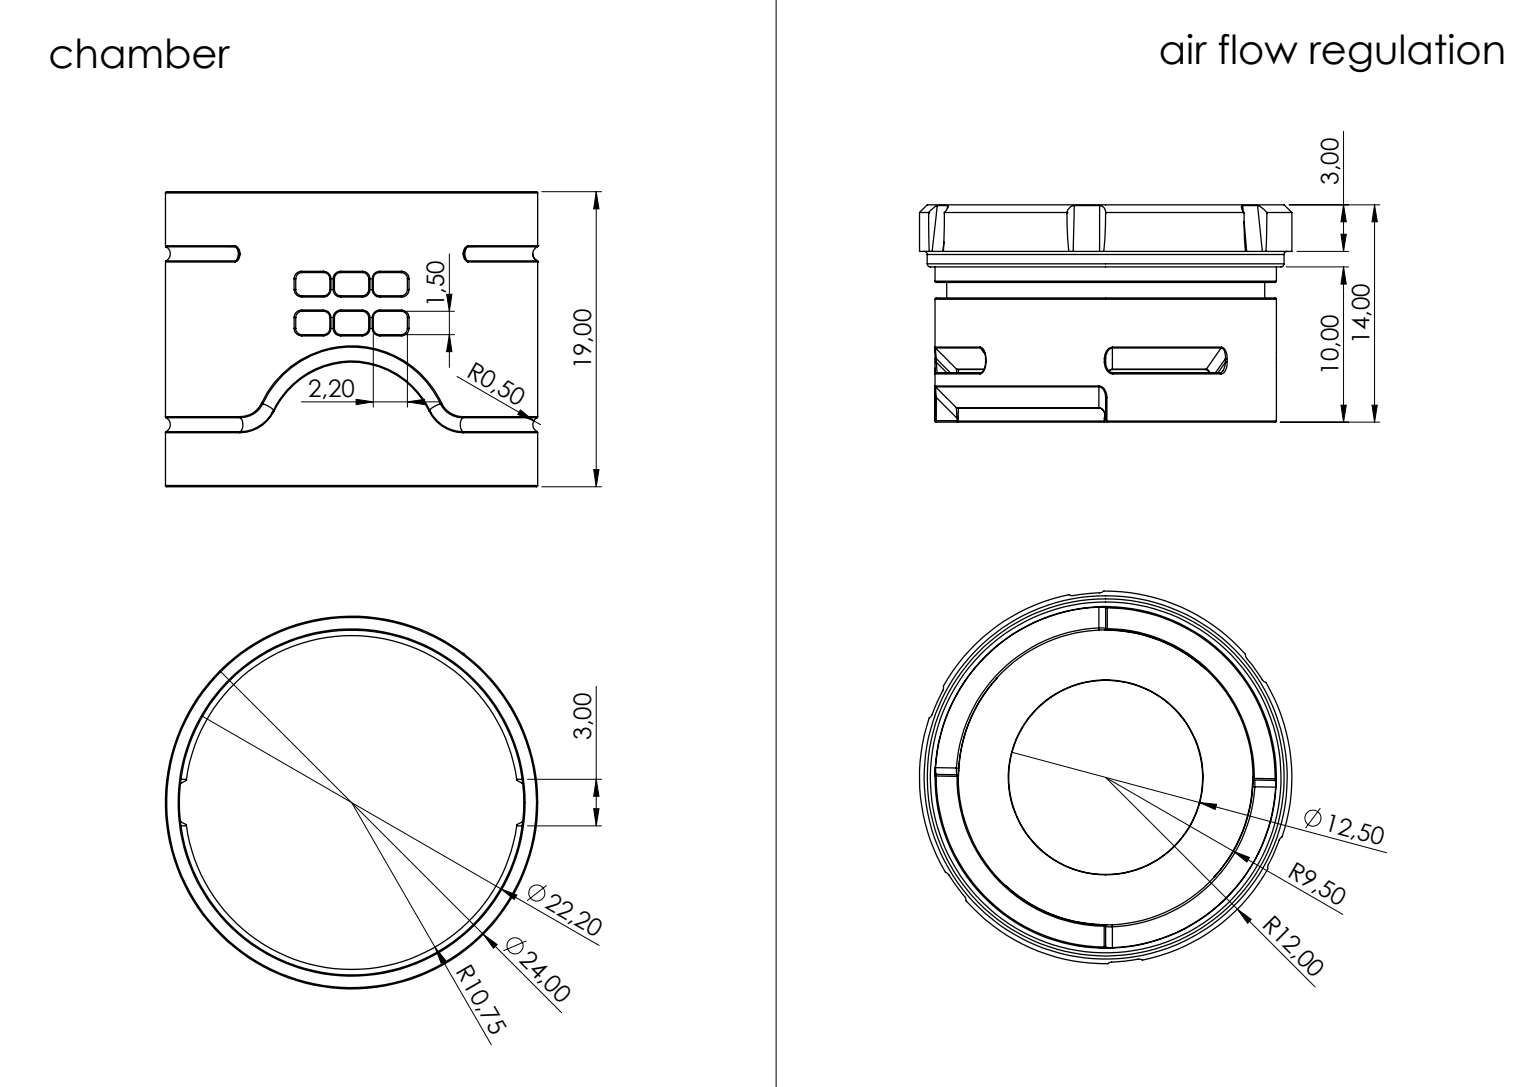
ISO-10303-21;
HEADER;
FILE_DESCRIPTION (('STEP AP214'),
    '1' );
FILE_NAME ('air flow regulation.step',
    '2026-10-05T20:10:51',
    ( '' ),
    ( '' ),
    'SwSTEP 2.0',
    'SolidWorks 2020',
    '' );
FILE_SCHEMA (( 'AUTOMOTIVE_DESIGN' ));
ENDSEC;

DATA;
#10=CARTESIAN_POINT ( 'NONE',  ( 8.996750068618124985, 1.000000000000000888, 7.838941051145326355 ) ) ;
#11=ADVANCED_FACE ( 'NONE', ( #143939 ), #115364, .T. ) ;
#35=CARTESIAN_POINT ( 'NONE',  ( -0.4382560683119374190, -5.166862915010145052, -10.99126615174919408 ) ) ;
#43=CARTESIAN_POINT ( 'NONE',  ( 0.000000000000000000, 4.000000000000003553, 0.000000000000000000 ) ) ;
#68=EDGE_LOOP ( 'NONE', ( #150530, #161755, #187821, #170704 ) ) ;
#69=CARTESIAN_POINT ( 'NONE',  ( 6.731761806397376091, -7.792646766724933727, 6.779954559072931985 ) ) ;
#135=ORIENTED_EDGE ( 'NONE', *, *, #160637, .F. ) ;
#138=CARTESIAN_POINT ( 'NONE',  ( 6.446420058208158110, -6.527411821100059797, 7.058808231563617142 ) ) ;
#156=VERTEX_POINT ( 'NONE', #175348 ) ;
#179=DIRECTION ( 'NONE',  ( 0.000000000000000000, 0.000000000000000000, -1.000000000000000000 ) ) ;
#202=CARTESIAN_POINT ( 'NONE',  ( 0.3663205537283338309, -5.223179855899201307, 10.97093617010627220 ) ) ;
#238=CARTESIAN_POINT ( 'NONE',  ( -6.451695228975252050, -8.176248043968191936, -7.005920419303019564 ) ) ;
#294=CARTESIAN_POINT ( 'NONE',  ( 7.654042494670958593E-16, 3.079999999999999183, -6.250000000000000000 ) ) ;
#317=VECTOR ( 'NONE', #161091, 1000.000000000000114 ) ;
#322=VERTEX_POINT ( 'NONE', #162281 ) ;
#357=PRESENTATION_STYLE_ASSIGNMENT (( #184467 ) ) ;
#401=VERTEX_POINT ( 'NONE', #180650 ) ;
#455=CARTESIAN_POINT ( 'NONE',  ( -10.99896775280371486, -5.324706741106397523, 0.1653080603930973391 ) ) ;
#523=CARTESIAN_POINT ( 'NONE',  ( 10.39230484541318589, 3.447199233515649386, -6.000000000000107470 ) ) ;
#529=( GEOMETRIC_REPRESENTATION_CONTEXT ( 3 ) GLOBAL_UNCERTAINTY_ASSIGNED_CONTEXT ( ( #23794 ) ) GLOBAL_UNIT_ASSIGNED_CONTEXT ( ( #120191, #135322, #18334 ) ) REPRESENTATION_CONTEXT ( 'NONE', 'WORKASPACE' ) );
#551=CARTESIAN_POINT ( 'NONE',  ( 10.99431798667268190, -5.199791778944933718, -0.3617173305618991974 ) ) ;
#571=AXIS2_PLACEMENT_3D ( 'NONE', #49828, #181943, #33573 ) ;
#585=CARTESIAN_POINT ( 'NONE',  ( -6.905598574191406769, -7.287292132484036955, -6.905598574191375683 ) ) ;
#620=CIRCLE ( 'NONE', #184019, 0.07999999999999951594 ) ;
#629=CARTESIAN_POINT ( 'NONE',  ( -0.1007670162816230591, -8.052608368926286175, -9.499791922504428499 ) ) ;
#644=CARTESIAN_POINT ( 'NONE',  ( 10.91970695577495043, 0.000000000000000000, 5.204170427930421283E-15 ) ) ;
#661=ORIENTED_EDGE ( 'NONE', *, *, #178265, .T. ) ;
#727=ORIENTED_EDGE ( 'NONE', *, *, #105154, .T. ) ;
#734=CARTESIAN_POINT ( 'NONE',  ( -7.235142258280575334, -6.594478602024302027, 7.235142258280601091 ) ) ;
#788=CARTESIAN_POINT ( 'NONE',  ( 6.717278222822382183, -7.473374494058216300, -6.830415307812249814 ) ) ;
#833=VECTOR ( 'NONE', #207710, 1000.000000000000000 ) ;
#842=ORIENTED_EDGE ( 'NONE', *, *, #62981, .F. ) ;
#869=AXIS2_PLACEMENT_3D ( 'NONE', #75473, #189221, #172990 ) ;
#886=UNCERTAINTY_MEASURE_WITH_UNIT (LENGTH_MEASURE( 1.000000000000000082E-05 ), #29913, 'distance_accuracy_value', 'NONE');
#918=CARTESIAN_POINT ( 'NONE',  ( -7.986233326679965216, -6.863455982311493564, 7.564733433744408764 ) ) ;
#954=EDGE_CURVE ( 'NONE', #82527, #56186, #181684, .T. ) ;
#1031=MECHANICAL_DESIGN_GEOMETRIC_PRESENTATION_REPRESENTATION('',(#101406),#122221);
#1044=DIRECTION ( 'NONE',  ( 0.000000000000000000, 1.000000000000000000, 0.000000000000000000 ) ) ;
#1055=CARTESIAN_POINT ( 'NONE',  ( 7.721398836998391246, -5.907420853759296264, 7.721398836998372595 ) ) ;
#1065=CARTESIAN_POINT ( 'NONE',  ( 0.000000000000000000, -9.063431457505059186, 0.000000000000000000 ) ) ;
#1080=CARTESIAN_POINT ( 'NONE',  ( 9.000007961041747606, 1.000000000000000888, 7.937244906211794238 ) ) ;
#1108=SURFACE_SIDE_STYLE ('',( #195073 ) ) ;
#1115=DIRECTION ( 'NONE',  ( 0.000000000000000000, 1.000000000000000000, 0.000000000000000000 ) ) ;
#1118=CARTESIAN_POINT ( 'NONE',  ( -5.204170427930421283E-15, -5.907420853759282053, 10.91970695577496997 ) ) ;
#1120=CARTESIAN_POINT ( 'NONE',  ( -0.08058608058609216529, -9.999999999999994671, -10.99970480893080271 ) ) ;
#1172=ADVANCED_FACE ( 'NONE', ( #46789 ), #131277, .T. ) ;
#1181=CARTESIAN_POINT ( 'NONE',  ( 0.07999999999999327094, -8.407420853759283830, 10.91970695577496286 ) ) ;
#1230=ORIENTED_EDGE ( 'NONE', *, *, #175281, .T. ) ;
#1236=CARTESIAN_POINT ( 'NONE',  ( 9.606148981167590861, -6.583980363595129504, -0.4355862708379804604 ) ) ;
#1239=CARTESIAN_POINT ( 'NONE',  ( -2.467126471220350226, 3.603011019375347068, 11.63837686854861886 ) ) ;
#1249=( GEOMETRIC_REPRESENTATION_CONTEXT ( 3 ) GLOBAL_UNCERTAINTY_ASSIGNED_CONTEXT ( ( #40635 ) ) GLOBAL_UNIT_ASSIGNED_CONTEXT ( ( #90258, #110825, #176833 ) ) REPRESENTATION_CONTEXT ( 'NONE', 'WORKASPACE' ) );
#1258=ORIENTED_EDGE ( 'NONE', *, *, #48325, .T. ) ;
#1267=ADVANCED_FACE ( 'NONE', ( #96609 ), #117015, .T. ) ;
#1301=VERTEX_POINT ( 'NONE', #170096 ) ;
#1303=ORIENTED_EDGE ( 'NONE', *, *, #173163, .T. ) ;
#1316=CARTESIAN_POINT ( 'NONE',  ( 9.499633409936901529, -9.910600865424404660, -0.08345703571627054174 ) ) ;
#1328=CARTESIAN_POINT ( 'NONE',  ( 9.578206935409037115, -9.746166700193986898, -0.1671882239534273895 ) ) ;
#1382=CARTESIAN_POINT ( 'NONE',  ( 7.752014238602739730E-16, 1.000000000000002665, -6.329999999999995630 ) ) ;
#1403=CARTESIAN_POINT ( 'NONE',  ( 2.494940289813108780, 3.499999999999989342, -11.73777120880564695 ) ) ;
#1422=CARTESIAN_POINT ( 'NONE',  ( -0.2887529476172396303, 1.000000000000000888, 11.89119375935166012 ) ) ;
#1434=( LENGTH_UNIT ( ) NAMED_UNIT ( * ) SI_UNIT ( .MILLI., .METRE. ) );
#1461=VECTOR ( 'NONE', #26119, 1000.000000000000000 ) ;
#1465=CARTESIAN_POINT ( 'NONE',  ( -6.766604819867150233, -7.256397064628574256, -6.766604819867120035 ) ) ;
#1472=DIRECTION ( 'NONE',  ( 0.000000000000000000, -1.000000000000000000, 0.000000000000000000 ) ) ;
#1528=CARTESIAN_POINT ( 'NONE',  ( -10.96107445065241315, -5.401429653175735979, 0.1376292675369562291 ) ) ;
#1532=( NAMED_UNIT ( * ) SI_UNIT ( $, .STERADIAN. ) SOLID_ANGLE_UNIT ( ) );
#1572=CARTESIAN_POINT ( 'NONE',  ( 9.611540586923190688, -6.723650695528643695, -0.1589091098076216013 ) ) ;
#1578=CARTESIAN_POINT ( 'NONE',  ( -4.480158349507305421E-13, -7.034525084948354490, 10.67552547708289268 ) ) ;
#1583=ORIENTED_EDGE ( 'NONE', *, *, #204878, .F. ) ;
#1589=CARTESIAN_POINT ( 'NONE',  ( -6.756361134959188774, -6.891066458783145166, -6.828399852920279400 ) ) ;
#1658=CARTESIAN_POINT ( 'NONE',  ( -11.00029519899100450, -6.134628647623513231, 8.483881999699072196E-15 ) ) ;
#1659=ADVANCED_FACE ( 'NONE', ( #152790 ), #205507, .T. ) ;
#1684=UNCERTAINTY_MEASURE_WITH_UNIT (LENGTH_MEASURE( 1.000000000000000082E-05 ), #105985, 'distance_accuracy_value', 'NONE');
#1708=CARTESIAN_POINT ( 'NONE',  ( -0.4644097342743139234, -8.233137084989849086, -9.488641820551089623 ) ) ;
#1746=DIRECTION ( 'NONE',  ( 0.03984146075563027578, 0.000000000000000000, 0.9992060137953822085 ) ) ;
#1753=DIRECTION ( 'NONE',  ( 0.000000000000000000, -1.084202172485501594E-14, -1.000000000000000000 ) ) ;
#1763=CARTESIAN_POINT ( 'NONE',  ( -6.735629246274043785E-15, -9.954379061088852509, 9.579665937614933569 ) ) ;
#1771=CARTESIAN_POINT ( 'NONE',  ( -7.721398836998370818, -5.907420853759296264, 7.721398836998400128 ) ) ;
#1785=DIRECTION ( 'NONE',  ( 0.9999455182791219254, 0.000000000000000000, -0.01043841336116897722 ) ) ;
#1801=VERTEX_POINT ( 'NONE', #63560 ) ;
#1811=CARTESIAN_POINT ( 'NONE',  ( -7.636191794455529092, -6.027819618361862197, 7.636191794455553961 ) ) ;
#1832=ORIENTED_EDGE ( 'NONE', *, *, #152899, .F. ) ;
#1838=CARTESIAN_POINT ( 'NONE',  ( 9.490416961614043245, -9.037429132956701139, -0.4317745627846678591 ) ) ;
#1871=VERTEX_POINT ( 'NONE', #114513 ) ;
#1887=CARTESIAN_POINT ( 'NONE',  ( 9.797921721691059460, 3.956598013261175772, 6.103348209225848642 ) ) ;
#1896=SURFACE_STYLE_FILL_AREA ( #165491 ) ;
#1902=ORIENTED_EDGE ( 'NONE', *, *, #91274, .F. ) ;
#1928=EDGE_CURVE ( 'NONE', #32900, #45587, #28933, .T. ) ;
#1931=CARTESIAN_POINT ( 'NONE',  ( 0.3618152180564599973, -5.223163831703878657, 10.97113184882214298 ) ) ;
#1978=DIRECTION ( 'NONE',  ( -0.9988044021632737079, 2.913101175831703182E-16, 0.04888523518676889112 ) ) ;
#2059=CIRCLE ( 'NONE', #123265, 0.08000000000000020983 ) ;
#2106=DIRECTION ( 'NONE',  ( 0.000000000000000000, 1.000000000000000000, 0.000000000000000000 ) ) ;
#2129=FACE_OUTER_BOUND ( 'NONE', #90690, .T. ) ;
#2169=EDGE_CURVE ( 'NONE', #89957, #26009, #98210, .T. ) ;
#2173=CARTESIAN_POINT ( 'NONE',  ( -0.3459972005395436367, -9.006862989983622114, 9.494064636159285087 ) ) ;
#2192=DIRECTION ( 'NONE',  ( 0.000000000000000000, 0.000000000000000000, -1.000000000000000000 ) ) ;
#2211=CARTESIAN_POINT ( 'NONE',  ( 11.29689844398643395, -5.530538574611989056, 9.269928574751062911E-15 ) ) ;
#2212=CIRCLE ( 'NONE', #109479, 10.99999999999999112 ) ;
#2238=CARTESIAN_POINT ( 'NONE',  ( -6.717278222822391953, 7.849261790823902629, 6.830415307812263137 ) ) ;
#2254=ORIENTED_EDGE ( 'NONE', *, *, #31074, .T. ) ;
#2263=CARTESIAN_POINT ( 'NONE',  ( 10.54982673430220252, -8.131911363926706215, -0.6210660986541617357 ) ) ;
#2298=B_SPLINE_CURVE_WITH_KNOTS ( 'NONE', 3,
 ( #197808, #82989, #212983, #98207, #49441, #15846 ),
 .UNSPECIFIED., .F., .F.,
 ( 4, 2, 4 ),
 ( 0.000000000000000000, 0.001226111284895915667, 0.002452222569791831768 ),
 .UNSPECIFIED. ) ;
#2309=CARTESIAN_POINT ( 'NONE',  ( -9.834497819152506537, 3.956598013261176217, -6.044631300485411529 ) ) ;
#2315=CARTESIAN_POINT ( 'NONE',  ( 0.4373225248172820656, -7.723431457505077979, -10.96785329849813273 ) ) ;
#2329=ORIENTED_EDGE ( 'NONE', *, *, #181317, .T. ) ;
#2362=ORIENTED_EDGE ( 'NONE', *, *, #105101, .T. ) ;
#2376=DIRECTION ( 'NONE',  ( 0.000000000000000000, -1.000000000000000000, 0.000000000000000000 ) ) ;
#2379=CARTESIAN_POINT ( 'NONE',  ( -10.99958311221863028, -9.919613946868093279, 0.09579086958121280082 ) ) ;
#2389=EDGE_CURVE ( 'NONE', #80737, #93709, #181246, .T. ) ;
#2405=CARTESIAN_POINT ( 'NONE',  ( 10.99943760478736010, -9.902953797791681723, -0.1112316694888297319 ) ) ;
#2480=CARTESIAN_POINT ( 'NONE',  ( -2.423460580168067757, 1.405705671057797312, 11.75284646727700455 ) ) ;
#2486=( NAMED_UNIT ( * ) PLANE_ANGLE_UNIT ( ) SI_UNIT ( $, .RADIAN. ) );
#2534=ORIENTED_EDGE ( 'NONE', *, *, #164125, .F. ) ;
#2539=CARTESIAN_POINT ( 'NONE',  ( 6.634380643896210294, -6.684699857435318471, 6.783773228136968036 ) ) ;
#2559=ORIENTED_EDGE ( 'NONE', *, *, #185505, .F. ) ;
#2599=CARTESIAN_POINT ( 'NONE',  ( -10.97067990664313264, -5.250949308401990479, 0.2977236940312626978 ) ) ;
#2601=CARTESIAN_POINT ( 'NONE',  ( 4.806723615010448736E-13, -7.868798029037617603, -9.500000000000001776 ) ) ;
#2610=CARTESIAN_POINT ( 'NONE',  ( 0.2619794211619203006, -6.848541063415906294, 10.99716886186657838 ) ) ;
#2635=EDGE_CURVE ( 'NONE', #192481, #119756, #206152, .T. ) ;
#2639=CARTESIAN_POINT ( 'NONE',  ( 9.484899655072776881, -6.713792789267319705, -0.3525790917591882789 ) ) ;
#2656=CARTESIAN_POINT ( 'NONE',  ( -5.204170427930421283E-15, 3.447199233515649386, -11.99999999999998224 ) ) ;
#2666=CARTESIAN_POINT ( 'NONE',  ( 0.4355862708379890647, -6.583980363594969631, 9.606148981167454082 ) ) ;
#2672=( GEOMETRIC_REPRESENTATION_CONTEXT ( 3 ) GLOBAL_UNCERTAINTY_ASSIGNED_CONTEXT ( ( #41987 ) ) GLOBAL_UNIT_ASSIGNED_CONTEXT ( ( #14906, #152407, #132983 ) ) REPRESENTATION_CONTEXT ( 'NONE', 'WORKASPACE' ) );
#2715=SURFACE_STYLE_USAGE ( .BOTH. , #5913 ) ;
#2753=STYLED_ITEM ( 'NONE', ( #168925 ), #37195 ) ;
#2797=ORIENTED_EDGE ( 'NONE', *, *, #2169, .T. ) ;
#2814=DIRECTION ( 'NONE',  ( -1.000000000000000000, 0.000000000000000000, 0.000000000000000000 ) ) ;
#2827=CARTESIAN_POINT ( 'NONE',  ( 1.730579039399254279E-05, -9.953931234596407052, 9.500331159997204011 ) ) ;
#2829=CIRCLE ( 'NONE', #144696, 0.07999999999999993228 ) ;
#2849=CARTESIAN_POINT ( 'NONE',  ( -7.727353211424288659, -6.453073674884717725, 7.679448064523577422 ) ) ;
#2852=CARTESIAN_POINT ( 'NONE',  ( -1.179069862577986269E-15, -8.198316280121948907, -9.513083155459820972 ) ) ;
#2865=EDGE_LOOP ( 'NONE', ( #190728, #42834, #5149, #106081 ) ) ;
#2870=EDGE_LOOP ( 'NONE', ( #204909, #147403, #53351, #186088 ) ) ;
#2889=ORIENTED_EDGE ( 'NONE', *, *, #89791, .F. ) ;
#2907=ORIENTED_EDGE ( 'NONE', *, *, #117967, .T. ) ;
#2920=DIRECTION ( 'NONE',  ( 1.561558963378126405E-12, 1.000000000000000000, 1.535693738323023938E-12 ) ) ;
#2921=CARTESIAN_POINT ( 'NONE',  ( -7.834948825496940827, -6.134628647623485698, -7.720982897393570354 ) ) ;
#2970=B_SPLINE_CURVE_WITH_KNOTS ( 'NONE', 3,
 ( #68679, #58594, #2610, #119655, #169405, #70808 ),
 .UNSPECIFIED., .F., .F.,
 ( 4, 2, 4 ),
 ( 0.000000000000000000, 0.0003147459536107388863, 0.0006294919072214776642 ),
 .UNSPECIFIED. ) ;
#2972=ORIENTED_EDGE ( 'NONE', *, *, #194076, .T. ) ;
#3055=CARTESIAN_POINT ( 'NONE',  ( -7.887197531381538340, -6.766388843766927508, 7.667935170093262975 ) ) ;
#3059=EDGE_LOOP ( 'NONE', ( #52191, #98069, #29595, #193700 ) ) ;
#3073=VECTOR ( 'NONE', #149450, 1000.000000000000000 ) ;
#3089=CARTESIAN_POINT ( 'NONE',  ( -0.3728355200475085285, -6.583727468837148322, -9.609247538825096413 ) ) ;
#3131=CARTESIAN_POINT ( 'NONE',  ( 9.007749180437182090, 1.970899860167747653, 7.589917856494929893 ) ) ;
#3155=CARTESIAN_POINT ( 'NONE',  ( -0.04481625915950731426, -9.999534456186221831, -9.500049708090200440 ) ) ;
#3160=ORIENTED_EDGE ( 'NONE', *, *, #11469, .F. ) ;
#3163=CARTESIAN_POINT ( 'NONE',  ( -0.09481041353608977984, -9.919511983836045488, -9.499526882191805299 ) ) ;
#3172=CARTESIAN_POINT ( 'NONE',  ( 0.07917133907661091929, -6.459673408256485949, 11.00057242252814760 ) ) ;
#3175=ORIENTED_EDGE ( 'NONE', *, *, #3623, .T. ) ;
#3181=CARTESIAN_POINT ( 'NONE',  ( 6.773846765317333762, -7.246166700180801001, 6.773846765317311558 ) ) ;
#3188=CARTESIAN_POINT ( 'NONE',  ( -9.499606442108964544, -9.746166700193986898, 0.08647222121513538362 ) ) ;
#3190=CARTESIAN_POINT ( 'NONE',  ( 0.000000000000000000, -7.723431457505077979, 0.000000000000000000 ) ) ;
#3195=SURFACE_SIDE_STYLE ('',( #85540 ) ) ;
#3197=EDGE_LOOP ( 'NONE', ( #209100, #72520, #9846, #141144 ) ) ;
#3207=CARTESIAN_POINT ( 'NONE',  ( -10.97895254167818990, -5.212340523078042409, 0.4373349612950744314 ) ) ;
#3210=ADVANCED_FACE ( 'NONE', ( #41628 ), #28556, .T. ) ;
#3214=ORIENTED_EDGE ( 'NONE', *, *, #200691, .T. ) ;
#3236=FILL_AREA_STYLE ('',( #151664 ) ) ;
#3309=CARTESIAN_POINT ( 'NONE',  ( -6.940534579975167873, -6.675176078274437153, 6.653311379900154421 ) ) ;
#3313=ORIENTED_EDGE ( 'NONE', *, *, #102930, .F. ) ;
#3370=FACE_OUTER_BOUND ( 'NONE', #25693, .T. ) ;
#3393=( GEOMETRIC_REPRESENTATION_CONTEXT ( 3 ) GLOBAL_UNCERTAINTY_ASSIGNED_CONTEXT ( ( #195972 ) ) GLOBAL_UNIT_ASSIGNED_CONTEXT ( ( #189438, #41080, #178527 ) ) REPRESENTATION_CONTEXT ( 'NONE', 'WORKASPACE' ) );
#3427=EDGE_LOOP ( 'NONE', ( #194768, #195116, #182169, #158522 ) ) ;
#3440=ORIENTED_EDGE ( 'NONE', *, *, #3532, .T. ) ;
#3449=CARTESIAN_POINT ( 'NONE',  ( -6.773376349083140013, -7.473374494058229622, -6.661184041420940893 ) ) ;
#3461=FACE_OUTER_BOUND ( 'NONE', #173063, .T. ) ;
#3469=CARTESIAN_POINT ( 'NONE',  ( 6.756361134959112391, -6.891066458783287274, 6.828399852920186142 ) ) ;
#3472=CARTESIAN_POINT ( 'NONE',  ( 0.000000000000000000, 1.000000000000000888, 0.000000000000000000 ) ) ;
#3532=EDGE_CURVE ( 'NONE', #157260, #71638, #13059, .T. ) ;
#3537=EDGE_CURVE ( 'NONE', #105884, #200355, #58064, .T. ) ;
#3541=B_SPLINE_CURVE_WITH_KNOTS ( 'NONE', 3,
 ( #196882, #64746, #148151, #181682 ),
 .UNSPECIFIED., .F., .F.,
 ( 4, 4 ),
 ( 0.000000000000000000, 9.170750102249441526E-05 ),
 .UNSPECIFIED. ) ;
#3557=DIRECTION ( 'NONE',  ( 0.000000000000000000, 1.000000000000000000, 0.000000000000000000 ) ) ;
#3571=EDGE_CURVE ( 'NONE', #129112, #183707, #115658, .T. ) ;
#3605=DIRECTION ( 'NONE',  ( 0.000000000000000000, -1.000000000000000000, 0.000000000000000000 ) ) ;
#3611=FACE_OUTER_BOUND ( 'NONE', #77172, .T. ) ;
#3621=FACE_OUTER_BOUND ( 'NONE', #70263, .T. ) ;
#3623=EDGE_CURVE ( 'NONE', #183133, #82411, #22756, .T. ) ;
#3629=CARTESIAN_POINT ( 'NONE',  ( -6.661184042391488980, -7.215568602681072363, 6.773376348128680391 ) ) ;
#3669=CIRCLE ( 'NONE', #187065, 8.049999999999993605 ) ;
#3716=CARTESIAN_POINT ( 'NONE',  ( -6.484567079770451770, -6.583980363594983842, -7.100579091573043122 ) ) ;
#3751=CARTESIAN_POINT ( 'NONE',  ( 10.94526678918447971, -5.600264386821002915, -0.03132844593992607785 ) ) ;
#3792=EDGE_CURVE ( 'NONE', #191954, #56186, #148063, .T. ) ;
#3806=UNCERTAINTY_MEASURE_WITH_UNIT (LENGTH_MEASURE( 1.000000000000000082E-05 ), #124958, 'distance_accuracy_value', 'NONE');
#3815=VECTOR ( 'NONE', #3943, 1000.000000000000000 ) ;
#3829=CARTESIAN_POINT ( 'NONE',  ( 0.08058608058607032165, -5.907420853759267843, -10.99970480893079916 ) ) ;
#3861=( NAMED_UNIT ( * ) PLANE_ANGLE_UNIT ( ) SI_UNIT ( $, .RADIAN. ) );
#3864=ORIENTED_EDGE ( 'NONE', *, *, #113758, .T. ) ;
#3916=DIRECTION ( 'NONE',  ( 0.000000000000000000, 0.000000000000000000, -1.000000000000000000 ) ) ;
#3937=AXIS2_PLACEMENT_3D ( 'NONE', #168326, #86007, #119639 ) ;
#3943=DIRECTION ( 'NONE',  ( 0.000000000000000000, 1.000000000000000000, 0.000000000000000000 ) ) ;
#3968=ORIENTED_EDGE ( 'NONE', *, *, #108052, .T. ) ;
#3990=FACE_OUTER_BOUND ( 'NONE', #157458, .T. ) ;
#4030=AXIS2_PLACEMENT_3D ( 'NONE', #178607, #77890, #98413 ) ;
#4095=B_SPLINE_CURVE_WITH_KNOTS ( 'NONE', 3,
 ( #171376, #88001, #55498, #187619, #185480, #54437, #37105, #20833 ),
 .UNSPECIFIED., .F., .F.,
 ( 4, 2, 2, 4 ),
 ( 0.000000000000000000, 0.0002185754043082796050, 0.0004371508086165592100, 0.0008743016172331182032 ),
 .UNSPECIFIED. ) ;
#4097=DIRECTION ( 'NONE',  ( 0.000000000000000000, 1.000000000000000000, 0.000000000000000000 ) ) ;
#4115=( LENGTH_UNIT ( ) NAMED_UNIT ( * ) SI_UNIT ( .MILLI., .METRE. ) );
#4172=EDGE_CURVE ( 'NONE', #157711, #182623, #58845, .T. ) ;
#4190=CARTESIAN_POINT ( 'NONE',  ( 0.000000000000000000, -7.666862915010147717, 0.000000000000000000 ) ) ;
#4201=EDGE_CURVE ( 'NONE', #168636, #175139, #105282, .T. ) ;
#4238=CARTESIAN_POINT ( 'NONE',  ( 0.01400375820003852204, -6.304807775344445808, 11.00039779440905896 ) ) ;
#4241=ORIENTED_EDGE ( 'NONE', *, *, #201124, .T. ) ;
#4271=CARTESIAN_POINT ( 'NONE',  ( -9.827407719474578585, -6.362962251424048254, 0.4359508081056245876 ) ) ;
#4299=ORIENTED_EDGE ( 'NONE', *, *, #14312, .F. ) ;
#4370=CARTESIAN_POINT ( 'NONE',  ( 7.720982897393571243, -5.907420853759296264, -7.834948825496923952 ) ) ;
#4376=CARTESIAN_POINT ( 'NONE',  ( -6.775478006741569637, -7.217909409563595169, 6.775478006741592729 ) ) ;
#4419=VECTOR ( 'NONE', #202531, 1000.000000000000000 ) ;
#4429=ADVANCED_FACE ( 'NONE', ( #170516 ), #84039, .T. ) ;
#4434=CARTESIAN_POINT ( 'NONE',  ( -10.87798840695972302, -6.646059016331640201, 0.1412570932018041570 ) ) ;
#4475=CARTESIAN_POINT ( 'NONE',  ( 10.14031698345507060, 3.934660213246449434, -5.561808457406779205 ) ) ;
#4491=CARTESIAN_POINT ( 'NONE',  ( -2.927345865710861577E-15, -6.948429295162506847, 9.261794192843273876 ) ) ;
#4537=CARTESIAN_POINT ( 'NONE',  ( 0.000000000000000000, -8.233137084989836652, 0.000000000000000000 ) ) ;
#4542=EDGE_CURVE ( 'NONE', #29585, #38980, #65003, .T. ) ;
#4548=CIRCLE ( 'NONE', #18331, 0.07999999999999982125 ) ;
#4566=AXIS2_PLACEMENT_3D ( 'NONE', #192689, #160212, #195917 ) ;
#4569=DIRECTION ( 'NONE',  ( 0.5254827454987551771, 0.7071067811865540120, 0.4731467892558094412 ) ) ;
#4615=CARTESIAN_POINT ( 'NONE',  ( -0.1236583036082171405, 1.000000000000000888, 11.99936284241579898 ) ) ;
#4627=( NAMED_UNIT ( * ) SI_UNIT ( $, .STERADIAN. ) SOLID_ANGLE_UNIT ( ) );
#4635=CARTESIAN_POINT ( 'NONE',  ( 0.08058608058607655278, -9.999999999999994671, 10.99970480893082225 ) ) ;
#4639=AXIS2_PLACEMENT_3D ( 'NONE', #184989, #4097, #134162 ) ;
#4660=FACE_OUTER_BOUND ( 'NONE', #40687, .T. ) ;
#4686=CARTESIAN_POINT ( 'NONE',  ( -4.218316008240990271E-13, -9.350066838357692589, -9.500000000000001776 ) ) ;
#4702=CIRCLE ( 'NONE', #129312, 0.08000000000000020983 ) ;
#4715=PLANE ( 'NONE',  #59335 ) ;
#4737=CARTESIAN_POINT ( 'NONE',  ( -9.579603127937250662, 7.849261790823902629, 0.08720040834116031536 ) ) ;
#4739=EDGE_LOOP ( 'NONE', ( #128508, #164924 ) ) ;
#4750=B_SPLINE_CURVE_WITH_KNOTS ( 'NONE', 3,
 ( #36336, #102414, #20080, #70954 ),
 .UNSPECIFIED., .F., .F.,
 ( 4, 4 ),
 ( 0.000000000000000000, 0.0002909236271752618720 ),
 .UNSPECIFIED. ) ;
#4751=CARTESIAN_POINT ( 'NONE',  ( -10.99915817693634246, -6.765468805240992367, 0.1539349733294695932 ) ) ;
#4765=ORIENTED_EDGE ( 'NONE', *, *, #43078, .F. ) ;
#4771=EDGE_LOOP ( 'NONE', ( #69677, #173344, #50516, #196043 ) ) ;
#4774=CARTESIAN_POINT ( 'NONE',  ( 7.834948825496932834, -5.907420853759296264, 7.720982897393583677 ) ) ;
#4778=CARTESIAN_POINT ( 'NONE',  ( -6.594971855056635412, -6.631671885544847989, -6.818239715405305823 ) ) ;
#4816=LINE ( 'NONE', #124042, #176034 ) ;
#4824=CARTESIAN_POINT ( 'NONE',  ( -7.720982897393583677, -5.907420853759296264, 7.834948825496934610 ) ) ;
#4845=CIRCLE ( 'NONE', #198605, 0.07999999999999993228 ) ;
#4848=EDGE_CURVE ( 'NONE', #183021, #118273, #2829, .T. ) ;
#4893=CARTESIAN_POINT ( 'NONE',  ( -1.572671215950735155E-14, -5.754340240174835586, -10.93220419382470610 ) ) ;
#4931=CARTESIAN_POINT ( 'NONE',  ( 0.000000000000000000, 0.000000000000000000, 0.000000000000000000 ) ) ;
#4952=CARTESIAN_POINT ( 'NONE',  ( 0.09916492693107491208, -9.920000000000095852, 9.499482423651659957 ) ) ;
#4954=CARTESIAN_POINT ( 'NONE',  ( 11.01272219801454888, 3.870433085555837316, -3.737564583532788642 ) ) ;
#4991=ORIENTED_EDGE ( 'NONE', *, *, #160078, .T. ) ;
#5003=AXIS2_PLACEMENT_3D ( 'NONE', #41374, #207035, #158314 ) ;
#5004=CARTESIAN_POINT ( 'NONE',  ( -10.91927143613604301, -9.998067526917992609, 0.1131244342389375046 ) ) ;
#5011=FACE_OUTER_BOUND ( 'NONE', #54886, .T. ) ;
#5044=STYLED_ITEM ( 'NONE', ( #7200 ), #90432 ) ;
#5053=AXIS2_PLACEMENT_3D ( 'NONE', #95542, #28374, #127032 ) ;
#5060=DIRECTION ( 'NONE',  ( -1.224646799147353207E-16, 0.000000000000000000, 1.000000000000000000 ) ) ;
#5108=CARTESIAN_POINT ( 'NONE',  ( -10.99953061226852746, -9.919996481109292219, 0.1022074249660880618 ) ) ;
#5149=ORIENTED_EDGE ( 'NONE', *, *, #164009, .T. ) ;
#5154=UNCERTAINTY_MEASURE_WITH_UNIT (LENGTH_MEASURE( 1.000000000000000082E-05 ), #1434, 'distance_accuracy_value', 'NONE');
#5161=EDGE_CURVE ( 'NONE', #214101, #184826, #67037, .T. ) ;
#5170=CIRCLE ( 'NONE', #77857, 9.636568542494918788 ) ;
#5178=CARTESIAN_POINT ( 'NONE',  ( 0.3868239129443627466, 2.972657967446813654, -11.65375889120575792 ) ) ;
#5201=SURFACE_STYLE_FILL_AREA ( #185033 ) ;
#5208=CARTESIAN_POINT ( 'NONE',  ( -0.4365953560983779069, -5.836144560139977955, -10.35465518852990385 ) ) ;
#5240=FACE_OUTER_BOUND ( 'NONE', #185647, .T. ) ;
#5287=ORIENTED_EDGE ( 'NONE', *, *, #128928, .T. ) ;
#5289=DIRECTION ( 'NONE',  ( 0.000000000000000000, 1.000000000000000000, 0.000000000000000000 ) ) ;
#5297=CARTESIAN_POINT ( 'NONE',  ( 0.4635785636673696586, -6.836568542494932288, 10.85353573482940703 ) ) ;
#5306=CIRCLE ( 'NONE', #119525, 10.86343145750506878 ) ;
#5313=DIRECTION ( 'NONE',  ( 0.000000000000000000, 0.000000000000000000, -1.000000000000000000 ) ) ;
#5319=EDGE_CURVE ( 'NONE', #74967, #176780, #106660, .T. ) ;
#5368=DIRECTION ( 'NONE',  ( 0.000000000000000000, 0.000000000000000000, 1.000000000000000000 ) ) ;
#5370=CIRCLE ( 'NONE', #33087, 10.91999999999999105 ) ;
#5371=CARTESIAN_POINT ( 'NONE',  ( 1.408343819019456176E-15, 0.7999999999999951594, 11.50000000000000000 ) ) ;
#5380=ORIENTED_EDGE ( 'NONE', *, *, #64826, .F. ) ;
#5382=EDGE_CURVE ( 'NONE', #18903, #170487, #159341, .T. ) ;
#5400=DIRECTION ( 'NONE',  ( 0.000000000000000000, 3.252606517456504467E-14, -1.000000000000000000 ) ) ;
#5413=ADVANCED_FACE ( 'NONE', ( #11130 ), #44741, .F. ) ;
#5435=CARTESIAN_POINT ( 'NONE',  ( 7.720982915750170150, -5.743759731405705615, -7.834948807407336346 ) ) ;
#5439=ORIENTED_EDGE ( 'NONE', *, *, #188097, .F. ) ;
#5447=VERTEX_POINT ( 'NONE', #144402 ) ;
#5468=CARTESIAN_POINT ( 'NONE',  ( 3.742823004191514212E-13, -7.217909409572238033, -9.581972888692755319 ) ) ;
#5480=CARTESIAN_POINT ( 'NONE',  ( -1.038038101541534383E-14, -8.644755361503008828, -10.68216772480108823 ) ) ;
#5492=DIRECTION ( 'NONE',  ( 0.000000000000000000, 0.000000000000000000, -1.000000000000000000 ) ) ;
#5506=DIRECTION ( 'NONE',  ( 0.000000000000000000, 1.000000000000000000, 0.000000000000000000 ) ) ;
#5511=ORIENTED_EDGE ( 'NONE', *, *, #96073, .T. ) ;
#5521=CARTESIAN_POINT ( 'NONE',  ( -7.503460210123537699, -6.893136966056810699, -8.043985462411194831 ) ) ;
#5546=ORIENTED_EDGE ( 'NONE', *, *, #102930, .T. ) ;
#5555=DIRECTION ( 'NONE',  ( 0.000000000000000000, 1.000000000000000000, 0.000000000000000000 ) ) ;
#5557=ORIENTED_EDGE ( 'NONE', *, *, #174069, .T. ) ;
#5562=EDGE_CURVE ( 'NONE', #151754, #8301, #113631, .T. ) ;
#5564=CARTESIAN_POINT ( 'NONE',  ( 0.4355862708379926174, -6.583980363595115293, 9.606148981167594414 ) ) ;
#5592=CARTESIAN_POINT ( 'NONE',  ( 0.4356160240586420263, -9.063431457505059186, -9.626717610576610795 ) ) ;
#5597=FACE_OUTER_BOUND ( 'NONE', #187539, .T. ) ;
#5625=CARTESIAN_POINT ( 'NONE',  ( 7.636191794455520210, -6.027819618361872855, -7.636191794455548632 ) ) ;
#5681=CARTESIAN_POINT ( 'NONE',  ( 0.3553982319964839043, -6.532648833121156962, 9.473247973006321487 ) ) ;
#5685=CARTESIAN_POINT ( 'NONE',  ( -5.204170427930421283E-15, -8.763419982614969683, 10.56339547890107688 ) ) ;
#5692=ORIENTED_EDGE ( 'NONE', *, *, #107653, .F. ) ;
#5694=CARTESIAN_POINT ( 'NONE',  ( -0.01138762994425885841, -7.792108994756149265, -9.500479199177400247 ) ) ;
#5732=CARTESIAN_POINT ( 'NONE',  ( 7.019253602638882761, -7.126685749119995528, 7.019253602638860556 ) ) ;
#5782=ADVANCED_FACE ( 'NONE', ( #190567 ), #108992, .T. ) ;
#5783=DIRECTION ( 'NONE',  ( 0.000000000000000000, 0.000000000000000000, -1.000000000000000000 ) ) ;
#5793=DIRECTION ( 'NONE',  ( 0.7408284471490504952, 0.000000000000000000, -0.6716942845482061220 ) ) ;
#5803=CARTESIAN_POINT ( 'NONE',  ( 10.99916818177027622, -10.00038292658552486, -0.1458870414463221132 ) ) ;
#5809=CARTESIAN_POINT ( 'NONE',  ( 0.4350533259329415481, -9.438199013093635514, -9.251577493846877331 ) ) ;
#5826=CARTESIAN_POINT ( 'NONE',  ( -10.99979681685432631, -6.306104522322589112, -0.07019693227476625497 ) ) ;
#5840=ORIENTED_EDGE ( 'NONE', *, *, #84110, .T. ) ;
#5886=FACE_OUTER_BOUND ( 'NONE', #3059, .T. ) ;
#5889=DIRECTION ( 'NONE',  ( -0.000000000000000000, -1.000000000000000000, -0.000000000000000000 ) ) ;
#5913=SURFACE_SIDE_STYLE ('',( #172731 ) ) ;
#5952=DIRECTION ( 'NONE',  ( 0.000000000000000000, 0.000000000000000000, -1.000000000000000000 ) ) ;
#6020=CARTESIAN_POINT ( 'NONE',  ( 10.95855051086948961, -7.723431457505071762, -0.6286713519883982970 ) ) ;
#6111=CARTESIAN_POINT ( 'NONE',  ( 9.499606442108984083, -9.580649465752458127, -0.08647222121308514864 ) ) ;
#6116=EDGE_CURVE ( 'NONE', #186972, #144331, #164280, .T. ) ;
#6124=CARTESIAN_POINT ( 'NONE',  ( -9.609247538824044810, -6.583727468838237229, 0.3728355200474647857 ) ) ;
#6152=CARTESIAN_POINT ( 'NONE',  ( 10.09384670631060921, -7.616807780225003377, 9.269928574751062911E-15 ) ) ;
#6238=DIRECTION ( 'NONE',  ( 0.000000000000000000, 1.000000000000000000, 0.000000000000000000 ) ) ;
#6255=EDGE_LOOP ( 'NONE', ( #29576, #72057, #160236, #82265 ) ) ;
#6259=ORIENTED_EDGE ( 'NONE', *, *, #211265, .F. ) ;
#6275=CARTESIAN_POINT ( 'NONE',  ( -11.40591166468356654, 3.507114751586590362, 3.706005353348402753 ) ) ;
#6313=CARTESIAN_POINT ( 'NONE',  ( 0.08058605481615531418, -8.243759731405756241, 10.99970480911961701 ) ) ;
#6325=EDGE_CURVE ( 'NONE', #54346, #18903, #212804, .T. ) ;
#6373=CARTESIAN_POINT ( 'NONE',  ( 0.000000000000000000, 3.799999999999998046, 0.000000000000000000 ) ) ;
#6381=CARTESIAN_POINT ( 'NONE',  ( -7.142181811248260459E-15, -6.134628647623513231, 10.91970695577494865 ) ) ;
#6397=PLANE ( 'NONE',  #161063 ) ;
#6402=CARTESIAN_POINT ( 'NONE',  ( 0.000000000000000000, 1.000000000000000888, 0.000000000000000000 ) ) ;
#6414=CARTESIAN_POINT ( 'NONE',  ( -9.251576347356463614, -6.938200158402487716, 0.4350533241460385336 ) ) ;
#6442=VERTEX_POINT ( 'NONE', #209050 ) ;
#6480=CARTESIAN_POINT ( 'NONE',  ( -2.494940289813118994, 3.499999999999989342, 11.73777120880565583 ) ) ;
#6485=AXIS2_PLACEMENT_3D ( 'NONE', #32500, #50884, #135352 ) ;
#6540=CARTESIAN_POINT ( 'NONE',  ( 2.494447209962474599, 3.467171072964057910, -11.73545145049397576 ) ) ;
#6558=CARTESIAN_POINT ( 'NONE',  ( -8.029456579251441184, -5.199789852012339786, 7.518896314322614849 ) ) ;
#6592=ORIENTED_EDGE ( 'NONE', *, *, #208257, .F. ) ;
#6599=DIRECTION ( 'NONE',  ( 0.000000000000000000, -1.000000000000000000, 0.000000000000000000 ) ) ;
#6602=CARTESIAN_POINT ( 'NONE',  ( -7.712222144930493073, -6.293595771081174739, -7.712222144930445999 ) ) ;
#6621=EDGE_CURVE ( 'NONE', #175139, #70421, #53455, .T. ) ;
#6637=DIRECTION ( 'NONE',  ( 0.000000000000000000, 0.000000000000000000, 1.000000000000000000 ) ) ;
#6640=B_SPLINE_CURVE_WITH_KNOTS ( 'NONE', 3,
 ( #136123, #105787, #55930, #53796, #167540, #169671, #21258, #87364, #121016, #153432, #188046, #154503, #88441, #5004, #104691, #71077 ),
 .UNSPECIFIED., .F., .F.,
 ( 4, 3, 3, 3, 3, 4 ),
 ( 0.000000000000000000, 2.208392919728564190E-05, 5.593630375490294554E-05, 8.978950068604114713E-05, 0.0001236430975991122182, 0.0001574962648025070408 ),
 .UNSPECIFIED. ) ;
#6641=EDGE_LOOP ( 'NONE', ( #175472, #208962, #21810, #13960 ) ) ;
#6643=VERTEX_POINT ( 'NONE', #57501 ) ;
#6659=CARTESIAN_POINT ( 'NONE',  ( -10.99943760478737786, -9.902953797791679946, 0.1112316694888332708 ) ) ;
#6663=CARTESIAN_POINT ( 'NONE',  ( -9.500370076773343442, -7.189371949516671023, 0.005973655271411463206 ) ) ;
#6678=CARTESIAN_POINT ( 'NONE',  ( 0.3870642018030800990, -8.176227079964631272, 9.516228778038660963 ) ) ;
#6691=DIRECTION ( 'NONE',  ( -0.6783731810844091381, 0.000000000000000000, -0.7347175152297780176 ) ) ;
#6748=CIRCLE ( 'NONE', #41284, 11.99999999999999112 ) ;
#6798=CARTESIAN_POINT ( 'NONE',  ( 0.07999999999999327094, -9.999999999999994671, 10.91970695577496286 ) ) ;
#6833=ORIENTED_EDGE ( 'NONE', *, *, #31446, .T. ) ;
#6852=CARTESIAN_POINT ( 'NONE',  ( 8.832353407160718817, 3.956598013261175772, 7.432338980325266853 ) ) ;
#6860=ORIENTED_EDGE ( 'NONE', *, *, #95154, .F. ) ;
#6880=FACE_OUTER_BOUND ( 'NONE', #198232, .T. ) ;
#6890=CARTESIAN_POINT ( 'NONE',  ( 0.000000000000000000, 7.849261790823902629, 8.049999999999993605 ) ) ;
#6892=AXIS2_PLACEMENT_3D ( 'NONE', #36732, #22605, #119127 ) ;
#6898=EDGE_CURVE ( 'NONE', #90583, #191645, #156657, .T. ) ;
#6925=DIRECTION ( 'NONE',  ( 0.000000000000000000, 1.000000000000000000, 0.000000000000000000 ) ) ;
#6944=CARTESIAN_POINT ( 'NONE',  ( 0.08641082498351806973, -9.914243671626374876, 10.99966068378002326 ) ) ;
#6990=CARTESIAN_POINT ( 'NONE',  ( -10.99622371251743225, -6.863149499369328055, 0.2970643657731258935 ) ) ;
#6993=FILL_AREA_STYLE_COLOUR ( '', #40467 ) ;
#7047=CARTESIAN_POINT ( 'NONE',  ( -0.08097581798161300470, -9.904508987438854106, -10.99970197202148547 ) ) ;
#7069=( LENGTH_UNIT ( ) NAMED_UNIT ( * ) SI_UNIT ( .MILLI., .METRE. ) );
#7086=CARTESIAN_POINT ( 'NONE',  ( -9.499623061593995388, -9.908700546396014275, 0.08463495275094737313 ) ) ;
#7087=CARTESIAN_POINT ( 'NONE',  ( 10.99039737178640230, -7.697079954928647716, -0.4645147939556434347 ) ) ;
#7104=CARTESIAN_POINT ( 'NONE',  ( 6.605500049835216103, -8.049367966558019560, 6.875062624577640058 ) ) ;
#7141=CARTESIAN_POINT ( 'NONE',  ( 9.043854491632929538, 2.018041202054163374, 8.143123160307325747 ) ) ;
#7151=ORIENTED_EDGE ( 'NONE', *, *, #126186, .T. ) ;
#7166=CARTESIAN_POINT ( 'NONE',  ( 2.530224277154552226, 2.018041202053995953, -11.90376931803466931 ) ) ;
#7171=VERTEX_POINT ( 'NONE', #30432 ) ;
#7194=EDGE_LOOP ( 'NONE', ( #98846, #38360, #129656, #61430 ) ) ;
#7195=ORIENTED_EDGE ( 'NONE', *, *, #161057, .F. ) ;
#7200=PRESENTATION_STYLE_ASSIGNMENT (( #189174 ) ) ;
#7307=PLANE ( 'NONE',  #52974 ) ;
#7333=CARTESIAN_POINT ( 'NONE',  ( -9.512045263456275990, -8.176568542494926817, 0.4655551865852147753 ) ) ;
#7358=CARTESIAN_POINT ( 'NONE',  ( -0.4362825330288316317, -6.085430761754772711, -10.10516068267230594 ) ) ;
#7379=CARTESIAN_POINT ( 'NONE',  ( -9.499562137383497529, -9.414773216041247395, 0.1228851354130223589 ) ) ;
#7382=CARTESIAN_POINT ( 'NONE',  ( 0.04325334852941317004, -8.075271019047999488, 11.00023204605253113 ) ) ;
#7438=VERTEX_POINT ( 'NONE', #17335 ) ;
#7451=CARTESIAN_POINT ( 'NONE',  ( -0.4373225248172924462, -7.723431457505077979, 10.96785329849814161 ) ) ;
#7456=EDGE_CURVE ( 'NONE', #6442, #201530, #213028, .T. ) ;
#7477=ORIENTED_EDGE ( 'NONE', *, *, #39920, .F. ) ;
#7484=DIRECTION ( 'NONE',  ( 0.000000000000000000, 0.000000000000000000, 1.000000000000000000 ) ) ;
#7489=ORIENTED_EDGE ( 'NONE', *, *, #207104, .F. ) ;
#7495=CARTESIAN_POINT ( 'NONE',  ( 7.245729715095587942, -5.507058666270979508, 7.863746947443980062 ) ) ;
#7506=CARTESIAN_POINT ( 'NONE',  ( 0.4363033266127375742, -8.563898737988809629, -10.12670668089735138 ) ) ;
#7536=VECTOR ( 'NONE', #199616, 1000.000000000000000 ) ;
#7539=CARTESIAN_POINT ( 'NONE',  ( -10.12536109763334835, -7.563986176625362212, 0.4645846211130850723 ) ) ;
#7559=CARTESIAN_POINT ( 'NONE',  ( 9.251576347356465391, -6.938200158402489492, -0.4350533241460284861 ) ) ;
#7617=CARTESIAN_POINT ( 'NONE',  ( -0.001121896803087802687, -7.189645481337962885, -9.584290747382974374 ) ) ;
#7649=DIRECTION ( 'NONE',  ( -0.000000000000000000, -1.000000000000000000, -0.000000000000000000 ) ) ;
#7685=EDGE_CURVE ( 'NONE', #45106, #127089, #57325, .T. ) ;
#7710=CARTESIAN_POINT ( 'NONE',  ( -3.577867169202164632E-15, -5.221050908132836454, 10.98765602437503652 ) ) ;
#7723=EDGE_CURVE ( 'NONE', #45056, #7438, #135925, .T. ) ;
#7729=DIRECTION ( 'NONE',  ( -0.000000000000000000, 1.000000000000000000, -0.000000000000000000 ) ) ;
#7730=FACE_OUTER_BOUND ( 'NONE', #105285, .T. ) ;
#7778=CARTESIAN_POINT ( 'NONE',  ( 7.821934338880105031, -6.709380320845391488, -7.553974597844388406 ) ) ;
#7819=CARTESIAN_POINT ( 'NONE',  ( -11.40591166468356654, 3.507114751586590362, 3.706005353348402753 ) ) ;
#7840=FILL_AREA_STYLE_COLOUR ( '', #145667 ) ;
#7841=CIRCLE ( 'NONE', #42522, 6.249999999999995559 ) ;
#7850=CARTESIAN_POINT ( 'NONE',  ( 0.07933194154488537597, -7.473374494045017968, -9.499668754385634628 ) ) ;
#7856=EDGE_CURVE ( 'NONE', #146171, #29173, #14129, .T. ) ;
#7893=ORIENTED_EDGE ( 'NONE', *, *, #126677, .T. ) ;
#7899=CARTESIAN_POINT ( 'NONE',  ( 0.000000000000000000, 1.000000000000000888, 0.000000000000000000 ) ) ;
#7932=CARTESIAN_POINT ( 'NONE',  ( -0.05648045292897504316, -9.990726591626529540, -10.91961852020054380 ) ) ;
#7938=SURFACE_STYLE_FILL_AREA ( #86005 ) ;
#7957=CARTESIAN_POINT ( 'NONE',  ( 10.99953061226852746, -9.919996481109301101, -0.1022074249662192763 ) ) ;
#7969=EDGE_CURVE ( 'NONE', #77260, #204799, #204949, .T. ) ;
#8006=DIRECTION ( 'NONE',  ( 0.000000000000000000, 0.000000000000000000, 1.000000000000000000 ) ) ;
#8011=CARTESIAN_POINT ( 'NONE',  ( -6.661184041420952440, -7.246166700180828535, 6.773376349083140013 ) ) ;
#8015=CARTESIAN_POINT ( 'NONE',  ( 8.103009739377979415, -6.893137084989842123, -7.439168848974011539 ) ) ;
#8062=DIRECTION ( 'NONE',  ( 0.000000000000000000, 0.000000000000000000, -1.000000000000000000 ) ) ;
#8122=( BOUNDED_SURFACE ( )  B_SPLINE_SURFACE ( 3, 2, ( 
 ( #131936, #98333, #148159 ),
 ( #78865, #114648, #214160 ),
 ( #64754, #17050, #182766 ),
 ( #48528, #130896, #180641 ) ),
 .UNSPECIFIED., .F., .F., .T. ) 
 B_SPLINE_SURFACE_WITH_KNOTS ( ( 4, 4 ),
 ( 3, 3 ),
 ( 0.000000000000000000, 9.170893476602704462E-05 ),
 ( 0.000000000000000000, 1.000000000000000000 ),
 .UNSPECIFIED. ) 
 GEOMETRIC_REPRESENTATION_ITEM ( )  RATIONAL_B_SPLINE_SURFACE ( (
 ( 1.000000000000000000, 0.7100530722026798802, 1.000000000000000000),
 ( 1.000000000000000000, 0.6998898451682473709, 1.000000000000000000),
 ( 1.000000000000000000, 0.6894756946157520883, 1.000000000000000000),
 ( 1.000000000000000000, 0.6787756258918292707, 1.000000000000000000) ) ) 
 REPRESENTATION_ITEM ( '' )  SURFACE ( )  );
#8158=SURFACE_STYLE_USAGE ( .BOTH. , #72072 ) ;
#8166=FACE_OUTER_BOUND ( 'NONE', #138541, .T. ) ;
#8174=CARTESIAN_POINT ( 'NONE',  ( -9.499607930503637832, -9.902952869712851935, 0.08630915044580420026 ) ) ;
#8191=CARTESIAN_POINT ( 'NONE',  ( 6.734029298721180723, -7.783114986501015409, 6.778728372092625243 ) ) ;
#8195=CARTESIAN_POINT ( 'NONE',  ( 0.000000000000000000, -6.583980363594990948, 0.000000000000000000 ) ) ;
#8224=SURFACE_SIDE_STYLE ('',( #191232 ) ) ;
#8280=CARTESIAN_POINT ( 'NONE',  ( 0.000000000000000000, 4.000000000000003553, 0.000000000000000000 ) ) ;
#8301=VERTEX_POINT ( 'NONE', #127865 ) ;
#8363=ADVANCED_FACE ( 'NONE', ( #62749 ), #34073, .T. ) ;
#8382=B_SPLINE_CURVE_WITH_KNOTS ( 'NONE', 3,
 ( #145180, #14041, #78000, #111641, #62810, #60680, #163527, #178716 ),
 .UNSPECIFIED., .F., .F.,
 ( 4, 2, 2, 4 ),
 ( 1.064888869118105810E-15, 0.0004636157603174413970, 0.0006954236404756280717, 0.0009272315206338146380 ),
 .UNSPECIFIED. ) ;
#8395=CARTESIAN_POINT ( 'NONE',  ( -0.09540182900466381843, -7.837949925775446580, 10.99983588129881618 ) ) ;
#8403=ORIENTED_EDGE ( 'NONE', *, *, #134540, .F. ) ;
#8427=ORIENTED_EDGE ( 'NONE', *, *, #18617, .F. ) ;
#8459=CARTESIAN_POINT ( 'NONE',  ( -0.4382560683119280931, -7.666862915010161039, 10.99126615174920651 ) ) ;
#8517=ORIENTED_EDGE ( 'NONE', *, *, #186328, .T. ) ;
#8544=DIRECTION ( 'NONE',  ( 0.000000000000000000, 1.000000000000000000, 0.000000000000000000 ) ) ;
#8550=DIRECTION ( 'NONE',  ( 0.000000000000000000, 0.000000000000000000, -1.000000000000000000 ) ) ;
#8585=CARTESIAN_POINT ( 'NONE',  ( 0.4373225248172820656, -7.723431457505077979, -10.96785329849813273 ) ) ;
#8630=CARTESIAN_POINT ( 'NONE',  ( 7.962224162659105708, -5.254973434576991842, -7.552496594302672506 ) ) ;
#8665=CARTESIAN_POINT ( 'NONE',  ( 10.91970695577495754, -6.134628647623513231, 0.08000000000000194456 ) ) ;
#8683=ORIENTED_EDGE ( 'NONE', *, *, #9580, .T. ) ;
#8694=ORIENTED_EDGE ( 'NONE', *, *, #200691, .F. ) ;
#8702=CARTESIAN_POINT ( 'NONE',  ( 10.39230484541318589, 3.447199233515649386, -6.000000000000107470 ) ) ;
#8705=CARTESIAN_POINT ( 'NONE',  ( -8.016215341155614738, -5.223177556212601047, 7.499070966594912235 ) ) ;
#8720=B_SPLINE_CURVE_WITH_KNOTS ( 'NONE', 3,
 ( #172114, #101773, #68180, #20504, #106092, #71377, #167841 ),
 .UNSPECIFIED., .F., .F.,
 ( 4, 3, 4 ),
 ( 0.0001932293135873436221, 0.0009000000018422016053, 0.002089330742406769661 ),
 .UNSPECIFIED. ) ;
#8729=DIRECTION ( 'NONE',  ( -0.06263215618328135670, 1.613675268591885659E-12, -0.9980366791916183145 ) ) ;
#8764=ADVANCED_FACE ( 'NONE', ( #64489 ), #70099, .F. ) ;
#8783=FACE_OUTER_BOUND ( 'NONE', #35541, .T. ) ;
#8785=DIRECTION ( 'NONE',  ( 0.000000000000000000, 0.000000000000000000, 1.000000000000000000 ) ) ;
#8792=ORIENTED_EDGE ( 'NONE', *, *, #52063, .F. ) ;
#8797=CARTESIAN_POINT ( 'NONE',  ( -10.99943592164172834, -8.407420853759269619, 0.1113975120798851026 ) ) ;
#8812=EDGE_CURVE ( 'NONE', #82411, #72492, #145783, .T. ) ;
#8825=ORIENTED_EDGE ( 'NONE', *, *, #7969, .T. ) ;
#8826=DIRECTION ( 'NONE',  ( -0.01043841336116890263, 0.000000000000000000, -0.9999455182791217034 ) ) ;
#8856=CARTESIAN_POINT ( 'NONE',  ( 1.255262969126035860E-15, 7.849261790823902629, -10.24999999999998934 ) ) ;
#8858=CARTESIAN_POINT ( 'NONE',  ( -0.005636796283178119316, -9.933099634201859374, -9.579656484007937678 ) ) ;
#8917=DIRECTION ( 'NONE',  ( 0.000000000000000000, 1.000000000000000000, 0.000000000000000000 ) ) ;
#8924=EDGE_LOOP ( 'NONE', ( #165319, #163579, #64494, #119140, #135611 ) ) ;
#8950=ADVANCED_FACE ( 'NONE', ( #72994 ), #17597, .T. ) ;
#8957=ORIENTED_EDGE ( 'NONE', *, *, #129734, .T. ) ;
#8989=FILL_AREA_STYLE ('',( #43654 ) ) ;
#9045=CARTESIAN_POINT ( 'NONE',  ( 0.4366903032816606411, -8.287795860939844772, -10.40306649911374670 ) ) ;
#9054=STYLED_ITEM ( 'NONE', ( #63098 ), #125431 ) ;
#9078=VERTEX_POINT ( 'NONE', #179964 ) ;
#9081=CARTESIAN_POINT ( 'NONE',  ( 6.818239715405162826, -6.631671885545136647, -6.594971855056806831 ) ) ;
#9112=CARTESIAN_POINT ( 'NONE',  ( -0.4648879685169910458, -7.768188185258928513, -9.920930332858617362 ) ) ;
#9155=CARTESIAN_POINT ( 'NONE',  ( -10.85353573482940881, -6.836568542494932288, 0.4635785636673760979 ) ) ;
#9212=CARTESIAN_POINT ( 'NONE',  ( -0.08058608058609216529, -9.902238891812018551, -10.99970480893080271 ) ) ;
#9298=CARTESIAN_POINT ( 'NONE',  ( 8.669853050660773164, 2.974000657017433102, 7.806370750281344861 ) ) ;
#9342=CARTESIAN_POINT ( 'NONE',  ( -0.4635785636673774857, -6.836568542494932288, -10.85353573482939460 ) ) ;
#9353=ORIENTED_EDGE ( 'NONE', *, *, #105154, .F. ) ;
#9354=CARTESIAN_POINT ( 'NONE',  ( 9.579764304849247125, -9.999999999999998224, -0.06720017513376763674 ) ) ;
#9357=CARTESIAN_POINT ( 'NONE',  ( 6.661184041420940005, -7.246166700180828535, -6.773376349083132908 ) ) ;
#9358=EDGE_CURVE ( 'NONE', #125304, #179210, #165876, .T. ) ;
#9360=AXIS2_PLACEMENT_3D ( 'NONE', #50594, #83082, #82023 ) ;
#9398=AXIS2_PLACEMENT_3D ( 'NONE', #1181, #31593, #131278 ) ;
#9414=CARTESIAN_POINT ( 'NONE',  ( 0.005636871015585881439, -9.933099847254503345, 10.91969863820290421 ) ) ;
#9476=ORIENTED_EDGE ( 'NONE', *, *, #200174, .F. ) ;
#9490=CONICAL_SURFACE ( 'NONE', #120261, 10.99999999999999112, 0.7853981633974425058 ) ;
#9496=CARTESIAN_POINT ( 'NONE',  ( 10.91838098853855321, -9.962496060591742975, -0.1694417511252848119 ) ) ;
#9507=CARTESIAN_POINT ( 'NONE',  ( -11.24798771954519871, -6.442483420751891288, 0.4630894006630780213 ) ) ;
#9518=MECHANICAL_DESIGN_GEOMETRIC_PRESENTATION_REPRESENTATION('',(#33791),#2672);
#9559=AXIS2_PLACEMENT_3D ( 'NONE', #91102, #41288, #177671 ) ;
#9567=DIRECTION ( 'NONE',  ( 0.000000000000000000, 0.000000000000000000, 1.000000000000000000 ) ) ;
#9573=CARTESIAN_POINT ( 'NONE',  ( 0.000000000000000000, 3.799999999999998046, 0.000000000000000000 ) ) ;
#9580=EDGE_CURVE ( 'NONE', #114068, #56213, #3541, .T. ) ;
#9635=DIRECTION ( 'NONE',  ( 0.9999580691339164940, -1.693994860858438588E-16, -0.009157509157509135383 ) ) ;
#9653=AXIS2_PLACEMENT_3D ( 'NONE', #148467, #183078, #34690 ) ;
#9711=CARTESIAN_POINT ( 'NONE',  ( -0.3617173305618593959, -5.199791778942955744, -10.99431798667224136 ) ) ;
#9742=COLOUR_RGB ( '', 0.40784314, 0.44705882, 0.49803922) ;
#9771=DIRECTION ( 'NONE',  ( -0.5000000000000102141, 0.000000000000000000, -0.8660254037844328234 ) ) ;
#9783=CARTESIAN_POINT ( 'NONE',  ( 0.08058608058607134861, -6.271284633940159559, -10.99970480893079916 ) ) ;
#9788=CARTESIAN_POINT ( 'NONE',  ( -9.946057155611605083, 2.515145635913770494, -6.189092007093218051 ) ) ;
#9808=ORIENTED_EDGE ( 'NONE', *, *, #78734, .F. ) ;
#9826=CARTESIAN_POINT ( 'NONE',  ( -9.499700864329909678, -7.154544010627095219, -0.07538891330675229208 ) ) ;
#9828=DIRECTION ( 'NONE',  ( -0.08676574618400526018, 0.9962285034897238045, -0.0006885664517735924335 ) ) ;
#9846=ORIENTED_EDGE ( 'NONE', *, *, #44338, .F. ) ;
#9849=CARTESIAN_POINT ( 'NONE',  ( -7.709579522695857001, -6.700642373080281544, -7.846302513400019940 ) ) ;
#9853=ORIENTED_EDGE ( 'NONE', *, *, #12404, .F. ) ;
#9860=CARTESIAN_POINT ( 'NONE',  ( 0.000000000000000000, -6.532648833121157850, 0.000000000000000000 ) ) ;
#9931=ORIENTED_EDGE ( 'NONE', *, *, #73977, .F. ) ;
#9978=ORIENTED_EDGE ( 'NONE', *, *, #82531, .T. ) ;
#10000=EDGE_LOOP ( 'NONE', ( #108378, #59114, #125054, #30437 ) ) ;
#10037=ORIENTED_EDGE ( 'NONE', *, *, #197437, .F. ) ;
#10040=LINE ( 'NONE', #109757, #116756 ) ;
#10143=CARTESIAN_POINT ( 'NONE',  ( 7.661067326845555137, -5.325441678136409784, 7.893838479094928751 ) ) ;
#10145=CARTESIAN_POINT ( 'NONE',  ( 0.08058608058607655278, -8.407420853759283830, 10.99970480893082225 ) ) ;
#10150=B_SPLINE_CURVE_WITH_KNOTS ( 'NONE', 3,
 ( #189465, #58404, #23754, #192645 ),
 .UNSPECIFIED., .F., .F.,
 ( 4, 4 ),
 ( 0.000000000000000000, 0.0002909236271752624683 ),
 .UNSPECIFIED. ) ;
#10155=EDGE_CURVE ( 'NONE', #31187, #101925, #6748, .T. ) ;
#10174=CARTESIAN_POINT ( 'NONE',  ( -0.4645846211130816306, -7.563986176625375535, -10.12536109763332526 ) ) ;
#10208=CIRCLE ( 'NONE', #134720, 10.99999999999999112 ) ;
#10241=VERTEX_POINT ( 'NONE', #173433 ) ;
#10291=ORIENTED_EDGE ( 'NONE', *, *, #105774, .F. ) ;
#10360=ORIENTED_EDGE ( 'NONE', *, *, #101405, .T. ) ;
#10370=CARTESIAN_POINT ( 'NONE',  ( 2.088542702721609690, 3.956598013261175772, -11.35310118413587510 ) ) ;
#10395=CARTESIAN_POINT ( 'NONE',  ( 0.08058608058607032165, -6.134628647623513231, -10.99970480893079916 ) ) ;
#10396=EDGE_CURVE ( 'NONE', #184431, #168636, #192837, .T. ) ;
#10466=CARTESIAN_POINT ( 'NONE',  ( 0.06712591543027901508, -9.995102890834049347, 10.91960056525075906 ) ) ;
#10471=CARTESIAN_POINT ( 'NONE',  ( -10.85277107007939001, 3.956598013261175772, 3.932872935640539414 ) ) ;
#10492=CARTESIAN_POINT ( 'NONE',  ( 6.640718169121218928, -6.363025497629811511, 7.257245574616259631 ) ) ;
#10530=ORIENTED_EDGE ( 'NONE', *, *, #128394, .T. ) ;
#10544=ORIENTED_EDGE ( 'NONE', *, *, #147046, .T. ) ;
#10587=CARTESIAN_POINT ( 'NONE',  ( -9.486534023829914730, -9.006863021369436950, 0.5123739589067574096 ) ) ;
#10610=EDGE_LOOP ( 'NONE', ( #177507, #184502, #89963, #50062 ) ) ;
#10624=PRESENTATION_STYLE_ASSIGNMENT (( #74585 ) ) ;
#10630=CARTESIAN_POINT ( 'NONE',  ( 0.08000000000000020983, 7.849261790823902629, -9.579665964948882007 ) ) ;
#10655=CARTESIAN_POINT ( 'NONE',  ( 0.2959466228873472438, -9.091099919222584091, -9.630212118911142483 ) ) ;
#10657=CARTESIAN_POINT ( 'NONE',  ( -6.937452841262697234, -7.242250812743805000, 6.937452841262715886 ) ) ;
#10699=CARTESIAN_POINT ( 'NONE',  ( 8.002408263930250953, -6.836568542494980250, -7.346809171966436125 ) ) ;
#10711=DIRECTION ( 'NONE',  ( -0.9998476951563912696, 0.000000000000000000, 0.01745240643728004568 ) ) ;
#10715=DIRECTION ( 'NONE',  ( 0.000000000000000000, 1.000000000000000000, 0.000000000000000000 ) ) ;
#10755=CARTESIAN_POINT ( 'NONE',  ( 8.013579835756319270, -5.223163706540481677, -7.501945787865609283 ) ) ;
#10791=EDGE_CURVE ( 'NONE', #160452, #37010, #210978, .T. ) ;
#10806=CARTESIAN_POINT ( 'NONE',  ( -9.797921721691023933, 3.956598013261175772, -6.103348209225892163 ) ) ;
#10871=DIRECTION ( 'NONE',  ( 0.000000000000000000, 0.000000000000000000, 1.000000000000000000 ) ) ;
#10901=CARTESIAN_POINT ( 'NONE',  ( 0.009341296487024523809, -9.943660733012633202, 9.579650209538311145 ) ) ;
#10902=CARTESIAN_POINT ( 'NONE',  ( 6.958662999125706961, -8.148356111791676071, -6.505896022970784287 ) ) ;
#10911=ORIENTED_EDGE ( 'NONE', *, *, #6116, .T. ) ;
#10974=ORIENTED_EDGE ( 'NONE', *, *, #26823, .F. ) ;
#11103=CARTESIAN_POINT ( 'NONE',  ( -10.99962150373186809, -9.919999999999998153, 0.09125116240079125807 ) ) ;
#11130=FACE_OUTER_BOUND ( 'NONE', #207955, .T. ) ;
#11139=CARTESIAN_POINT ( 'NONE',  ( 10.33323920393400286, 4.021557182957047338, 5.965898435991960902 ) ) ;
#11157=DIRECTION ( 'NONE',  ( 1.224646799147353207E-16, 0.000000000000000000, -1.000000000000000000 ) ) ;
#11162=CARTESIAN_POINT ( 'NONE',  ( 6.764690511086886823E-16, -5.511313137147262786, 11.00000000000000178 ) ) ;
#11205=FACE_OUTER_BOUND ( 'NONE', #153685, .T. ) ;
#11248=FACE_OUTER_BOUND ( 'NONE', #80750, .T. ) ;
#11281=( NAMED_UNIT ( * ) SI_UNIT ( $, .STERADIAN. ) SOLID_ANGLE_UNIT ( ) );
#11382=AXIS2_PLACEMENT_3D ( 'NONE', #137681, #202638, #122579 ) ;
#11404=CARTESIAN_POINT ( 'NONE',  ( 10.38894090356631139, 1.970899860167849127, -5.551243578533891387 ) ) ;
#11438=DIRECTION ( 'NONE',  ( 0.000000000000000000, 1.000000000000000000, 0.000000000000000000 ) ) ;
#11465=CARTESIAN_POINT ( 'NONE',  ( -0.2118258318330372425, -6.614835951978776940, -10.99866081003794527 ) ) ;
#11469=EDGE_CURVE ( 'NONE', #121012, #213712, #206703, .T. ) ;
#11471=COLOUR_RGB ( '', 0.31764706, 0.68627451, 0.89019608) ;
#11490=CARTESIAN_POINT ( 'NONE',  ( -1.040834085586084257E-14, -7.126685749120009739, 9.926723642588090257 ) ) ;
#11555=AXIS2_PLACEMENT_3D ( 'NONE', #54180, #33655, #2192 ) ;
#11598=CARTESIAN_POINT ( 'NONE',  ( 7.967649405165779797, -5.251137252134810751, -7.547231044119373067 ) ) ;
#11627=AXIS2_PLACEMENT_3D ( 'NONE', #57571, #123729, #41342 ) ;
#11630=ORIENTED_EDGE ( 'NONE', *, *, #5161, .T. ) ;
#11631=STYLED_ITEM ( 'NONE', ( #120690 ), #56751 ) ;
#11642=CARTESIAN_POINT ( 'NONE',  ( 11.41267819554179042, 3.499999999999989342, -3.708203932499494648 ) ) ;
#11655=CARTESIAN_POINT ( 'NONE',  ( 11.28709712336965332, 1.000000000000000888, -3.871943585350003048 ) ) ;
#11658=CARTESIAN_POINT ( 'NONE',  ( -9.490381562237910629, -9.037089468803426229, 0.4325416218483088548 ) ) ;
#11665=DIRECTION ( 'NONE',  ( 0.000000000000000000, 1.000000000000000000, 0.000000000000000000 ) ) ;
#11694=EDGE_CURVE ( 'NONE', #146105, #41517, #124877, .T. ) ;
#11697=CARTESIAN_POINT ( 'NONE',  ( 7.800371912476624203, -5.581885079358428925, 7.755938900619411491 ) ) ;
#11703=FACE_OUTER_BOUND ( 'NONE', #195943, .T. ) ;
#11725=CARTESIAN_POINT ( 'NONE',  ( -7.019253602638862333, -7.126685749119995528, 7.019253602638880984 ) ) ;
#11734=EDGE_CURVE ( 'NONE', #18521, #148587, #190134, .T. ) ;
#11743=CARTESIAN_POINT ( 'NONE',  ( -6.980013479859874082, -8.233136965322266576, 6.444907381559366932 ) ) ;
#11767=( LENGTH_UNIT ( ) NAMED_UNIT ( * ) SI_UNIT ( .MILLI., .METRE. ) );
#11778=CARTESIAN_POINT ( 'NONE',  ( -11.18654035131441127, 1.000000000000000888, 4.041720556560751021 ) ) ;
#11779=ADVANCED_FACE ( 'NONE', ( #43834 ), #76307, .T. ) ;
#11782=CARTESIAN_POINT ( 'NONE',  ( -10.98241130803290488, 3.975933801733734896, 3.568401746110938966 ) ) ;
#11834=DIRECTION ( 'NONE',  ( 0.000000000000000000, 1.000000000000000000, 0.000000000000000000 ) ) ;
#11864=CARTESIAN_POINT ( 'NONE',  ( 0.03436587256740384483, -7.792803924024841677, 9.554207839743742881 ) ) ;
#11889=CARTESIAN_POINT ( 'NONE',  ( -9.000007961041697868, 1.000000000000000888, -7.937244906211844864 ) ) ;
#11915=DIRECTION ( 'NONE',  ( 0.000000000000000000, 1.000000000000000000, 0.000000000000000000 ) ) ;
#11978=CARTESIAN_POINT ( 'NONE',  ( 7.768428355093493387, -6.306978362809817718, 7.788485247865709837 ) ) ;
#11979=CARTESIAN_POINT ( 'NONE',  ( 6.784764760059096567, -8.039737506397907296, -6.649736275991404710 ) ) ;
#11984=EDGE_LOOP ( 'NONE', ( #37305, #163075 ) ) ;
#11990=CARTESIAN_POINT ( 'NONE',  ( -10.99856159529784883, -8.101932402265175526, 0.2004767358929543664 ) ) ;
#11996=CARTESIAN_POINT ( 'NONE',  ( -10.39230484541323740, 3.447199233515621408, 6.000000000000048850 ) ) ;
#12018=ORIENTED_EDGE ( 'NONE', *, *, #78925, .T. ) ;
#12025=CARTESIAN_POINT ( 'NONE',  ( -7.779015489124656568, -5.502990254781792601, -7.777446446097291854 ) ) ;
#12062=ORIENTED_EDGE ( 'NONE', *, *, #108718, .F. ) ;
#12089=CARTESIAN_POINT ( 'NONE',  ( 6.710064404886807665, -7.791858861492818811, 6.725651841507094275 ) ) ;
#12092=CARTESIAN_POINT ( 'NONE',  ( 0.07999999999999327094, -9.900000000000005684, 10.99970695577496294 ) ) ;
#12127=ORIENTED_EDGE ( 'NONE', *, *, #102286, .F. ) ;
#12153=STYLED_ITEM ( 'NONE', ( #181723 ), #119978 ) ;
#12178=CARTESIAN_POINT ( 'NONE',  ( 11.34781316621058167, 4.021557182957059773, -3.687128006873058972 ) ) ;
#12190=CARTESIAN_POINT ( 'NONE',  ( 7.728718841570989539, -6.124285368609183600, -7.728718841571019738 ) ) ;
#12206=ORIENTED_EDGE ( 'NONE', *, *, #201199, .F. ) ;
#12267=CARTESIAN_POINT ( 'NONE',  ( 7.008396152629535081, -6.708819892820519826, -6.400381488218290116 ) ) ;
#12275=CARTESIAN_POINT ( 'NONE',  ( 0.08865135991732026044, -9.916958638733639475, 9.499586356067553083 ) ) ;
#12310=CARTESIAN_POINT ( 'NONE',  ( -7.657759090810044356, -5.412329794880681888, -7.842350841322879518 ) ) ;
#12329=VERTEX_POINT ( 'NONE', #153044 ) ;
#12404=EDGE_CURVE ( 'NONE', #35104, #168888, #100027, .T. ) ;
#12423=( NAMED_UNIT ( * ) SI_UNIT ( $, .STERADIAN. ) SOLID_ANGLE_UNIT ( ) );
#12446=MECHANICAL_DESIGN_GEOMETRIC_PRESENTATION_REPRESENTATION('',(#64121),#91953);
#12472=CARTESIAN_POINT ( 'NONE',  ( 10.20634067979172421, 1.972237431424189724, -5.892633538921025149 ) ) ;
#12497=EDGE_LOOP ( 'NONE', ( #125717, #95681, #200545, #165254 ) ) ;
#12531=CARTESIAN_POINT ( 'NONE',  ( -0.3183146091065937600, -6.808378554901762136, -10.86152993230180996 ) ) ;
#12568=SURFACE_STYLE_USAGE ( .BOTH. , #165224 ) ;
#12572=CARTESIAN_POINT ( 'NONE',  ( -7.968844136639799736, -5.196967604326695245, 7.583016927391841300 ) ) ;
#12576=CARTESIAN_POINT ( 'NONE',  ( 0.000000000000000000, -2.000000000000001776, 0.000000000000000000 ) ) ;
#12640=ORIENTED_EDGE ( 'NONE', *, *, #170841, .T. ) ;
#12650=SURFACE_SIDE_STYLE ('',( #194608 ) ) ;
#12658=CARTESIAN_POINT ( 'NONE',  ( 8.024185963717927805, -5.166862990899748986, -7.524604700374135646 ) ) ;
#12663=VERTEX_POINT ( 'NONE', #143237 ) ;
#12677=CARTESIAN_POINT ( 'NONE',  ( 7.721398836998367265, -6.134628647623499909, -7.721398836998390358 ) ) ;
#12686=CARTESIAN_POINT ( 'NONE',  ( -10.34804403480111290, -6.705807696129545192, 1.138412281109779656E-15 ) ) ;
#12687=ORIENTED_EDGE ( 'NONE', *, *, #41532, .T. ) ;
#12707=EDGE_CURVE ( 'NONE', #160219, #138893, #179794, .T. ) ;
#12737=VECTOR ( 'NONE', #139743, 1000.000000000000000 ) ;
#12745=B_SPLINE_CURVE_WITH_KNOTS ( 'NONE', 3,
 ( #197392, #145505, #49034, #115154, #32771, #66301, #132450 ),
 .UNSPECIFIED., .F., .F.,
 ( 4, 3, 4 ),
 ( 0.0001126021370636952904, 0.0006031550062628992376, 0.002006790698585253496 ),
 .UNSPECIFIED. ) ;
#12751=( NAMED_UNIT ( * ) PLANE_ANGLE_UNIT ( ) SI_UNIT ( $, .RADIAN. ) );
#12770=CIRCLE ( 'NONE', #133904, 0.07999999999999980738 ) ;
#12783=CARTESIAN_POINT ( 'NONE',  ( -0.3866937364864243554, 3.956598013261175772, 11.53692321988874170 ) ) ;
#12836=CARTESIAN_POINT ( 'NONE',  ( 2.093037498677865482, 1.000000000000000888, -11.70868840297833025 ) ) ;
#12884=CARTESIAN_POINT ( 'NONE',  ( 0.000000000000000000, -5.199999999999996625, 0.000000000000000000 ) ) ;
#12906=CARTESIAN_POINT ( 'NONE',  ( -6.776370306708066948, -7.161464053357560644, -6.781144757626046626 ) ) ;
#12907=EDGE_CURVE ( 'NONE', #40132, #100951, #62610, .T. ) ;
#12915=DIRECTION ( 'NONE',  ( 0.000000000000000000, 1.000000000000000000, 0.000000000000000000 ) ) ;
#12918=FACE_OUTER_BOUND ( 'NONE', #67370, .T. ) ;
#12923=CARTESIAN_POINT ( 'NONE',  ( -0.01181297548617084130, -7.619382996155810162, 9.500232605409157927 ) ) ;
#12936=AXIS2_PLACEMENT_3D ( 'NONE', #22540, #134215, #200224 ) ;
#12956=EDGE_CURVE ( 'NONE', #155393, #174410, #162653, .T. ) ;
#12966=EDGE_CURVE ( 'NONE', #12329, #157711, #152263, .T. ) ;
#13021=DIRECTION ( 'NONE',  ( 0.000000000000000000, -0.7071067811865540120, -0.7071067811865410224 ) ) ;
#13037=CARTESIAN_POINT ( 'NONE',  ( -0.1298625177950053222, -9.252181021551008300, 9.620122301472909143 ) ) ;
#13039=ORIENTED_EDGE ( 'NONE', *, *, #136104, .F. ) ;
#13051=CARTESIAN_POINT ( 'NONE',  ( 0.000000000000000000, -5.223431457505076203, 0.000000000000000000 ) ) ;
#13059=CIRCLE ( 'NONE', #68404, 10.86343145750506700 ) ;
#13065=CARTESIAN_POINT ( 'NONE',  ( -9.579665964947855272, -7.246166700193438892, 1.021860547567587929E-14 ) ) ;
#13075=ORIENTED_EDGE ( 'NONE', *, *, #194704, .T. ) ;
#13078=ORIENTED_EDGE ( 'NONE', *, *, #149988, .F. ) ;
#13118=CARTESIAN_POINT ( 'NONE',  ( -7.653681110113423891, -5.402328468025351604, -7.847520364415503380 ) ) ;
#13152=CARTESIAN_POINT ( 'NONE',  ( -9.578796289607002024, -9.978085408363298825, 0.1296641399399101613 ) ) ;
#13246=CARTESIAN_POINT ( 'NONE',  ( 10.85353573482951717, -6.836568542495036205, -0.4635785636673637189 ) ) ;
#13251=CARTESIAN_POINT ( 'NONE',  ( 11.57407876878489716, 2.018041202053835637, -3.760646157729463646 ) ) ;
#13252=CARTESIAN_POINT ( 'NONE',  ( -6.905598479220833141, -7.287292266636207216, 6.905598479220857122 ) ) ;
#13255=SURFACE_STYLE_USAGE ( .BOTH. , #98787 ) ;
#13262=CARTESIAN_POINT ( 'NONE',  ( 7.960263458884762500, -6.452016312668102493, -7.960263458884791810 ) ) ;
#13277=SURFACE_SIDE_STYLE ('',( #130315 ) ) ;
#13326=ORIENTED_EDGE ( 'NONE', *, *, #167509, .F. ) ;
#13347=CARTESIAN_POINT ( 'NONE',  ( -9.500385102287568273, -7.162053774861992572, 0.01083140255525295165 ) ) ;
#13394=CARTESIAN_POINT ( 'NONE',  ( -7.662794434365309826, -5.790678129197943669, 7.045261094876549279 ) ) ;
#13500=CARTESIAN_POINT ( 'NONE',  ( 0.000000000000000000, 4.000000000000003553, 0.000000000000000000 ) ) ;
#13524=AXIS2_PLACEMENT_3D ( 'NONE', #106642, #173755, #25332 ) ;
#13529=B_SPLINE_CURVE_WITH_KNOTS ( 'NONE', 3,
 ( #100607, #34536, #121218, #84357, #20412, #136327, #51873 ),
 .UNSPECIFIED., .F., .F.,
 ( 4, 3, 4 ),
 ( 0.0001135037245265573214, 0.001517139415464327252, 0.002007692284160955340 ),
 .UNSPECIFIED. ) ;
#13584=CYLINDRICAL_SURFACE ( 'NONE', #200530, 9.499999999999992895 ) ;
#13592=FACE_OUTER_BOUND ( 'NONE', #80481, .T. ) ;
#13601=COLOUR_RGB ( '', 0.09019608, 0.27058824, 0.51372549) ;
#13612=CARTESIAN_POINT ( 'NONE',  ( -0.4659925305415743568, -6.893137084989842123, -10.91005274787796786 ) ) ;
#13614=EDGE_CURVE ( 'NONE', #72492, #401, #96438, .T. ) ;
#13643=CARTESIAN_POINT ( 'NONE',  ( -7.836475020641954004, -5.360178282914185743, 7.719547554928810840 ) ) ;
#13729=CARTESIAN_POINT ( 'NONE',  ( 8.016215341155765728, -5.223177556212426964, -7.499070966595000165 ) ) ;
#13813=CARTESIAN_POINT ( 'NONE',  ( 5.301814855701348250, 3.000000000000002665, 1.561251128379126385E-14 ) ) ;
#13843=CARTESIAN_POINT ( 'NONE',  ( 9.520891725235928860, -8.148349307653536044, -0.3199376857464704682 ) ) ;
#13848=VECTOR ( 'NONE', #89131, 1000.000000000000000 ) ;
#13865=EDGE_CURVE ( 'NONE', #89267, #15203, #135168, .T. ) ;
#13886=CARTESIAN_POINT ( 'NONE',  ( -5.737959331755660019E-16, -8.256136661604607241, -10.93205753685918680 ) ) ;
#13960=ORIENTED_EDGE ( 'NONE', *, *, #149988, .T. ) ;
#13977=CARTESIAN_POINT ( 'NONE',  ( -10.14031698345510080, 3.934660213246443661, 5.561808457406734796 ) ) ;
#14041=CARTESIAN_POINT ( 'NONE',  ( -6.764898216727353919, -7.628386336122861877, -6.764898216730279579 ) ) ;
#14059=EDGE_CURVE ( 'NONE', #157630, #130351, #165718, .T. ) ;
#14084=B_SPLINE_CURVE_WITH_KNOTS ( 'NONE', 3,
 ( #133244, #34634, #166781, #203507, #185133, #188344, #87659, #35697 ),
 .UNSPECIFIED., .F., .F.,
 ( 4, 2, 2, 4 ),
 ( 1.064888869118067945E-15, 0.0004636157603174408007, 0.0006954236404756272043, 0.0009272315206338136622 ),
 .UNSPECIFIED. ) ;
#14092=CARTESIAN_POINT ( 'NONE',  ( 7.503460210123510166, -6.893136966056697901, 8.043985462411230358 ) ) ;
#14093=CARTESIAN_POINT ( 'NONE',  ( 6.779954559072996823, -7.792646766724983465, -6.731761806397363657 ) ) ;
#14106=CARTESIAN_POINT ( 'NONE',  ( 0.000000000000000000, 0.2000000000000057288, 0.000000000000000000 ) ) ;
#14119=CARTESIAN_POINT ( 'NONE',  ( -9.500350659417458488, -7.217450603046464686, 0.002323312720852115966 ) ) ;
#14129=LINE ( 'NONE', #130129, #116313 ) ;
#14167=FACE_OUTER_BOUND ( 'NONE', #190762, .T. ) ;
#14171=ORIENTED_EDGE ( 'NONE', *, *, #111938, .F. ) ;
#14200=CARTESIAN_POINT ( 'NONE',  ( 6.649736275991402934, -8.039737506397919731, 6.784764760059098343 ) ) ;
#14204=MECHANICAL_DESIGN_GEOMETRIC_PRESENTATION_REPRESENTATION('',(#52270),#169921);
#14226=CARTESIAN_POINT ( 'NONE',  ( 0.000000000000000000, -9.919999999999998153, 0.000000000000000000 ) ) ;
#14232=CARTESIAN_POINT ( 'NONE',  ( -6.725445687907764203, -7.162053774861991684, 6.710127771514628137 ) ) ;
#14247=VERTEX_POINT ( 'NONE', #87060 ) ;
#14256=VERTEX_POINT ( 'NONE', #6852 ) ;
#14269=CARTESIAN_POINT ( 'NONE',  ( -10.99970480893081870, -5.907420853759282053, -0.08058608058607828750 ) ) ;
#14292=CARTESIAN_POINT ( 'NONE',  ( -0.08058962652509195357, -9.910877166163972518, -10.99970478295253606 ) ) ;
#14312=EDGE_CURVE ( 'NONE', #144299, #39263, #113849, .T. ) ;
#14329=EDGE_LOOP ( 'NONE', ( #102177, #100842, #104147, #211135, #136774 ) ) ;
#14330=B_SPLINE_CURVE_WITH_KNOTS ( 'NONE', 3,
 ( #146958, #126499, #209776, #62478, #212973, #145903, #46250 ),
 .UNSPECIFIED., .F., .F.,
 ( 4, 3, 4 ),
 ( 0.000000000000000000, 0.0008000000000005097218, 0.002977368225425562533 ),
 .UNSPECIFIED. ) ;
#14336=CARTESIAN_POINT ( 'NONE',  ( -5.204170427930421283E-15, 4.000000000000003553, -11.99999999999998224 ) ) ;
#14342=FACE_OUTER_BOUND ( 'NONE', #161977, .T. ) ;
#14399=DIRECTION ( 'NONE',  ( 0.000000000000000000, 0.000000000000000000, 1.000000000000000000 ) ) ;
#14458=ORIENTED_EDGE ( 'NONE', *, *, #26377, .T. ) ;
#14559=DIRECTION ( 'NONE',  ( 0.000000000000000000, 1.000000000000000000, 0.000000000000000000 ) ) ;
#14591=( BOUNDED_SURFACE ( )  B_SPLINE_SURFACE ( 3, 2, ( 
 ( #85259, #38656, #204316 ),
 ( #6124, #200064, #138301 ),
 ( #76216, #51716, #19184 ),
 ( #151348, #68989, #146589 ),
 ( #64245, #212606, #209394 ),
 ( #161757, #96772, #180128 ),
 ( #160676, #130388, #195315 ),
 ( #62114, #13347, #208336 ) ),
 .UNSPECIFIED., .F., .F., .T. ) 
 B_SPLINE_SURFACE_WITH_KNOTS ( ( 4, 2, 2, 4 ),
 ( 3, 3 ),
 ( 0.000000000000000000, 0.0002204160392919248554, 0.0004408320785838497108, 0.0008816641571676994216 ),
 ( 0.000000000000000000, 1.000000000000000000 ),
 .UNSPECIFIED. ) 
 GEOMETRIC_REPRESENTATION_ITEM ( )  RATIONAL_B_SPLINE_SURFACE ( (
 ( 1.000000000000000000, 0.4127341956165088144, 1.000000000000000000),
 ( 1.000000000000000000, 0.4103180386330694818, 1.000000000000000000),
 ( 1.000000000000000000, 0.4223234233959186623, 1.000000000000000000),
 ( 1.000000000000000000, 0.4613847219397944066, 1.000000000000000000),
 ( 1.000000000000000000, 0.4878744032655861762, 1.000000000000000000),
 ( 1.000000000000000000, 0.5702658980234645014, 1.000000000000000000),
 ( 1.000000000000000000, 0.6280001242509920534, 1.000000000000000000),
 ( 1.000000000000000000, 0.6787756258918242747, 1.000000000000000000) ) ) 
 REPRESENTATION_ITEM ( '' )  SURFACE ( )  );
#14606=VECTOR ( 'NONE', #21533, 1000.000000000000000 ) ;
#14615=VERTEX_POINT ( 'NONE', #29280 ) ;
#14644=ORIENTED_EDGE ( 'NONE', *, *, #190890, .T. ) ;
#14663=CARTESIAN_POINT ( 'NONE',  ( 0.4294425147611402038, -9.199999999999990408, -9.490288674561773163 ) ) ;
#14696=CARTESIAN_POINT ( 'NONE',  ( -7.876942567271134621, -5.350481869465722795, 7.629869294364564070 ) ) ;
#14711=AXIS2_PLACEMENT_3D ( 'NONE', #177849, #198326, #63011 ) ;
#14720=CARTESIAN_POINT ( 'NONE',  ( 0.000000000000000000, -1.000000000000000888, -10.91999999999999105 ) ) ;
#14728=ORIENTED_EDGE ( 'NONE', *, *, #31789, .F. ) ;
#14816=CARTESIAN_POINT ( 'NONE',  ( 8.879134602966002987, 3.426985321572576293, 7.474367077670482473 ) ) ;
#14828=CARTESIAN_POINT ( 'NONE',  ( 0.000000000000000000, -9.999999999999994671, 10.99999999999999112 ) ) ;
#14865=ORIENTED_EDGE ( 'NONE', *, *, #139862, .T. ) ;
#14902=CARTESIAN_POINT ( 'NONE',  ( 9.566809970445889988, -7.630846356335490022, -1.058098698307930843E-15 ) ) ;
#14906=( LENGTH_UNIT ( ) NAMED_UNIT ( * ) SI_UNIT ( .MILLI., .METRE. ) );
#14908=CARTESIAN_POINT ( 'NONE',  ( 10.99970480893080449, -5.740513804456437441, 0.08058608058608245084 ) ) ;
#14948=CARTESIAN_POINT ( 'NONE',  ( 0.000000000000000000, 4.000000000000003553, 0.000000000000000000 ) ) ;
#14956=CARTESIAN_POINT ( 'NONE',  ( 9.716492259128738596, -7.972382850425319134, -0.4652101495396395170 ) ) ;
#14979=ORIENTED_EDGE ( 'NONE', *, *, #185505, .T. ) ;
#14992=UNCERTAINTY_MEASURE_WITH_UNIT (LENGTH_MEASURE( 1.000000000000000082E-05 ), #112474, 'distance_accuracy_value', 'NONE');
#15018=CARTESIAN_POINT ( 'NONE',  ( -9.499766273075886502, -10.00000000000010303, 0.06663900456894483737 ) ) ;
#15048=CARTESIAN_POINT ( 'NONE',  ( -10.14375151705083766, -9.181160345032697734, 0.1770598413457937226 ) ) ;
#15053=B_SPLINE_CURVE_WITH_KNOTS ( 'NONE', 3,
 ( #77076, #27256, #144275, #78144 ),
 .UNSPECIFIED., .F., .F.,
 ( 4, 4 ),
 ( 0.000000000000000000, 9.170750102249612288E-05 ),
 .UNSPECIFIED. ) ;
#15084=AXIS2_PLACEMENT_3D ( 'NONE', #132118, #99580, #165644 ) ;
#15095=CONICAL_SURFACE ( 'NONE', #136187, 6.540947088288920241, 0.7853981633974536081 ) ;
#15103=DIRECTION ( 'NONE',  ( 0.000000000000000000, -1.000000000000000000, 0.000000000000000000 ) ) ;
#15126=ORIENTED_EDGE ( 'NONE', *, *, #166817, .F. ) ;
#15131=CARTESIAN_POINT ( 'NONE',  ( -8.743186976631616147, 3.870433085555829766, -7.668514896535084446 ) ) ;
#15162=ORIENTED_EDGE ( 'NONE', *, *, #105101, .F. ) ;
#15165=CARTESIAN_POINT ( 'NONE',  ( 0.02890288085936086604, -9.971207159576023216, 9.579616049094571650 ) ) ;
#15187=DIRECTION ( 'NONE',  ( 0.000000000000000000, 1.000000000000000000, 0.000000000000000000 ) ) ;
#15203=VERTEX_POINT ( 'NONE', #181893 ) ;
#15232=CIRCLE ( 'NONE', #101678, 6.277139874739035008 ) ;
#15245=ORIENTED_EDGE ( 'NONE', *, *, #135027, .T. ) ;
#15272=CARTESIAN_POINT ( 'NONE',  ( -9.578353140444630043, -9.943513495888055331, 0.1579188828665830657 ) ) ;
#15288=VERTEX_POINT ( 'NONE', #35650 ) ;
#15329=CARTESIAN_POINT ( 'NONE',  ( 10.10286202908859110, -8.578580700073974441, -0.6127037010540555828 ) ) ;
#15332=EDGE_CURVE ( 'NONE', #115124, #19069, #28868, .T. ) ;
#15354=EDGE_CURVE ( 'NONE', #90575, #167635, #47094, .T. ) ;
#15365=CARTESIAN_POINT ( 'NONE',  ( 10.98241130803287646, 3.975933801733736672, -3.568401746111017570 ) ) ;
#15366=CARTESIAN_POINT ( 'NONE',  ( -7.869907033622098425, -7.024005807131032064, 7.214015686748106226 ) ) ;
#15402=ADVANCED_FACE ( 'NONE', ( #175021 ), #89505, .T. ) ;
#15407=CARTESIAN_POINT ( 'NONE',  ( -0.08058608058608779379, -5.907420853759267843, 10.99970480893080804 ) ) ;
#15426=ORIENTED_EDGE ( 'NONE', *, *, #40826, .F. ) ;
#15455=VERTEX_POINT ( 'NONE', #42895 ) ;
#15494=CARTESIAN_POINT ( 'NONE',  ( 2.093037498677865482, 1.000000000000000888, -11.70868840297833025 ) ) ;
#15504=CARTESIAN_POINT ( 'NONE',  ( -7.710915694720370972, -5.615420858948579230, -7.765925996254657626 ) ) ;
#15514=CARTESIAN_POINT ( 'NONE',  ( 0.000000000000000000, 0.7999999999999951594, 0.000000000000000000 ) ) ;
#15528=ADVANCED_FACE ( 'NONE', ( #58047 ), #77083, .F. ) ;
#15571=DIRECTION ( 'NONE',  ( 0.000000000000000000, 0.000000000000000000, 1.000000000000000000 ) ) ;
#15575=MECHANICAL_DESIGN_GEOMETRIC_PRESENTATION_REPRESENTATION('',(#181629),#67362);
#15606=ORIENTED_EDGE ( 'NONE', *, *, #110555, .T. ) ;
#15617=FILL_AREA_STYLE ('',( #30846 ) ) ;
#15624=EDGE_CURVE ( 'NONE', #147438, #81487, #126778, .T. ) ;
#15665=CARTESIAN_POINT ( 'NONE',  ( 10.64229060209973454, 1.016282880930359234, -6.144329343916673736 ) ) ;
#15681=ORIENTED_EDGE ( 'NONE', *, *, #57019, .T. ) ;
#15689=COLOUR_RGB ( '', 0.66274510, 0.83137255, 0.94901961) ;
#15707=ORIENTED_EDGE ( 'NONE', *, *, #177065, .F. ) ;
#15712=EDGE_LOOP ( 'NONE', ( #25730, #38611, #32130, #45142 ) ) ;
#15715=CARTESIAN_POINT ( 'NONE',  ( 0.4645879757426182866, -7.605490376146398113, 10.08385597498928554 ) ) ;
#15737=UNCERTAINTY_MEASURE_WITH_UNIT (LENGTH_MEASURE( 1.000000000000000082E-05 ), #142410, 'distance_accuracy_value', 'NONE');
#15846=CARTESIAN_POINT ( 'NONE',  ( 10.32992389895506413, 1.000000000000000888, 6.106772653521394645 ) ) ;
#15877=DIRECTION ( 'NONE',  ( 0.000000000000000000, 0.000000000000000000, 1.000000000000000000 ) ) ;
#15879=CARTESIAN_POINT ( 'NONE',  ( -0.3123298761244324151, -8.144690279336741057, -9.521443730523929005 ) ) ;
#15928=EDGE_LOOP ( 'NONE', ( #12206, #50682, #166097, #175057, #75827 ) ) ;
#15970=ORIENTED_EDGE ( 'NONE', *, *, #17921, .T. ) ;
#15976=TOROIDAL_SURFACE ( 'NONE', #178517, 10.92000000000000171, 0.08000000000000000167 ) ;
#15984=CARTESIAN_POINT ( 'NONE',  ( -9.499766273075884726, -9.919999999999998153, 0.06663900456894793212 ) ) ;
#16008=CARTESIAN_POINT ( 'NONE',  ( -6.484567079770452658, -6.583980363594976737, -7.100579091573040458 ) ) ;
#16013=FILL_AREA_STYLE_COLOUR ( '', #115960 ) ;
#16045=AXIS2_PLACEMENT_3D ( 'NONE', #96032, #28875, #179401 ) ;
#16064=FACE_OUTER_BOUND ( 'NONE', #158643, .T. ) ;
#16080=CARTESIAN_POINT ( 'NONE',  ( -9.578928831967228774, -10.00000000000000178, 0.1215685829351347697 ) ) ;
#16107=CARTESIAN_POINT ( 'NONE',  ( -7.750016138724920900, -6.480061791515684178, 7.806764249273700607 ) ) ;
#16116=UNCERTAINTY_MEASURE_WITH_UNIT (LENGTH_MEASURE( 1.000000000000000082E-05 ), #64787, 'distance_accuracy_value', 'NONE');
#16181=ORIENTED_EDGE ( 'NONE', *, *, #66045, .T. ) ;
#16220=DIRECTION ( 'NONE',  ( 0.000000000000000000, 1.000000000000000000, 0.000000000000000000 ) ) ;
#16221=CARTESIAN_POINT ( 'NONE',  ( 6.773846765316601903, -7.473374494057218875, -6.773846765316623220 ) ) ;
#16224=DIRECTION ( 'NONE',  ( 0.000000000000000000, -1.000000000000000000, 0.000000000000000000 ) ) ;
#16231=ADVANCED_FACE ( 'NONE', ( #169411 ), #87092, .T. ) ;
#16248=CARTESIAN_POINT ( 'NONE',  ( 9.488725015150309972, -6.691474851359264342, -0.09393477316944856548 ) ) ;
#16273=CARTESIAN_POINT ( 'NONE',  ( 10.98997987423603817, -6.893137084989856334, -0.4694063952341778756 ) ) ;
#16291=CARTESIAN_POINT ( 'NONE',  ( -0.2442642247113720744, -5.209160580580717514, -10.99754090108938875 ) ) ;
#16301=CARTESIAN_POINT ( 'NONE',  ( -0.1329251406260706092, -9.135512438678663472, 9.499304248211860369 ) ) ;
#16346=ORIENTED_EDGE ( 'NONE', *, *, #5319, .T. ) ;
#16355=AXIS2_PLACEMENT_3D ( 'NONE', #45653, #28315, #80263 ) ;
#16358=DIRECTION ( 'NONE',  ( 0.000000000000000000, 1.000000000000000000, 0.000000000000000000 ) ) ;
#16378=ORIENTED_EDGE ( 'NONE', *, *, #103623, .T. ) ;
#16420=EDGE_LOOP ( 'NONE', ( #68221, #187077, #179832, #15162 ) ) ;
#16426=CARTESIAN_POINT ( 'NONE',  ( 1.347111479062087616E-15, -9.999999999999994671, -10.99999999999999112 ) ) ;
#16429=CARTESIAN_POINT ( 'NONE',  ( 6.745922712994594228, -7.817744194000437297, 6.689586359223958389 ) ) ;
#16457=COLOUR_RGB ( '', 0.08235294, 0.09019608, 0.10196078) ;
#16465=VERTEX_POINT ( 'NONE', #121813 ) ;
#16492=VERTEX_POINT ( 'NONE', #71883 ) ;
#16500=ADVANCED_FACE ( 'NONE', ( #74051 ), #144216, .T. ) ;
#16557=CARTESIAN_POINT ( 'NONE',  ( -9.492899823913846902, -8.233137084989849086, 0.3774118403930767918 ) ) ;
#16586=ORIENTED_EDGE ( 'NONE', *, *, #128001, .F. ) ;
#16665=CARTESIAN_POINT ( 'NONE',  ( -0.003376046620573100454, -7.161464053357560644, -9.586610838029425707 ) ) ;
#16675=ORIENTED_EDGE ( 'NONE', *, *, #1928, .T. ) ;
#16725=FILL_AREA_STYLE ('',( #17784 ) ) ;
#16752=AXIS2_PLACEMENT_3D ( 'NONE', #74669, #61611, #139694 ) ;
#16753=CARTESIAN_POINT ( 'NONE',  ( 0.3870405448657153191, 1.264806443676224301, -11.85654951141427560 ) ) ;
#16773=CARTESIAN_POINT ( 'NONE',  ( -2.346281263894411939E-15, -6.452016312669646148, 11.25751254361626685 ) ) ;
#16788=CARTESIAN_POINT ( 'NONE',  ( 0.1412570932018001879, -6.646059016331635760, 10.87798840695972657 ) ) ;
#16816=( NAMED_UNIT ( * ) PLANE_ANGLE_UNIT ( ) SI_UNIT ( $, .RADIAN. ) );
#16836=CONICAL_SURFACE ( 'NONE', #134414, 11.53746066217573762, 0.1181278931043537039 ) ;
#16843=CARTESIAN_POINT ( 'NONE',  ( -0.1309013025973339017, -5.411711732698793575, -10.96028113393447256 ) ) ;
#16847=ORIENTED_EDGE ( 'NONE', *, *, #45640, .F. ) ;
#16901=CARTESIAN_POINT ( 'NONE',  ( -0.4373347461412381287, -7.712532583864843083, 10.97876033714414135 ) ) ;
#16905=CIRCLE ( 'NONE', #196754, 0.08000000000000009881 ) ;
#16913=ORIENTED_EDGE ( 'NONE', *, *, #186479, .F. ) ;
#16931=CARTESIAN_POINT ( 'NONE',  ( 0.000000000000000000, -2.079999999999998295, 10.91999999999999105 ) ) ;
#16939=FACE_OUTER_BOUND ( 'NONE', #130765, .T. ) ;
#16942=CARTESIAN_POINT ( 'NONE',  ( -0.008219159353565024667, -7.627132808484227589, -9.567202289542832361 ) ) ;
#16971=CARTESIAN_POINT ( 'NONE',  ( -7.720982897393580124, -6.134628647623485698, 7.834948825496934610 ) ) ;
#17050=CARTESIAN_POINT ( 'NONE',  ( 6.713552092917008274, -7.189371949512688431, 6.722000117219741000 ) ) ;
#17061=EDGE_LOOP ( 'NONE', ( #77138, #132250, #78062, #39506 ) ) ;
#17156=EDGE_CURVE ( 'NONE', #18033, #7438, #95796, .T. ) ;
#17160=ORIENTED_EDGE ( 'NONE', *, *, #142193, .F. ) ;
#17171=FACE_OUTER_BOUND ( 'NONE', #58730, .T. ) ;
#17182=CARTESIAN_POINT ( 'NONE',  ( -10.39398850336074709, -8.287668210030888716, 0.6181847325715009722 ) ) ;
#17202=LINE ( 'NONE', #116921, #153026 ) ;
#17226=DIRECTION ( 'NONE',  ( 0.9781476007338056888, 0.000000000000000000, 0.2079116908177593703 ) ) ;
#17227=DIRECTION ( 'NONE',  ( 0.000000000000000000, -1.000000000000000000, 0.000000000000000000 ) ) ;
#17232=CARTESIAN_POINT ( 'NONE',  ( -0.08000000000000367928, -9.900000000000005684, -9.579665964948867796 ) ) ;
#17258=SURFACE_STYLE_USAGE ( .BOTH. , #165669 ) ;
#17272=EDGE_CURVE ( 'NONE', #22857, #113870, #95632, .T. ) ;
#17318=CARTESIAN_POINT ( 'NONE',  ( 9.492660725451591119, -6.771447601804259975, -0.03895569783345582265 ) ) ;
#17324=CARTESIAN_POINT ( 'NONE',  ( 0.000000000000000000, -9.006862915010128035, 0.000000000000000000 ) ) ;
#17335=CARTESIAN_POINT ( 'NONE',  ( 10.10176665042273392, 1.000000000000000888, 6.279211784079129721 ) ) ;
#17360=ORIENTED_EDGE ( 'NONE', *, *, #85411, .F. ) ;
#17365=DIRECTION ( 'NONE',  ( -0.000000000000000000, 1.000000000000000000, -0.000000000000000000 ) ) ;
#17368=CARTESIAN_POINT ( 'NONE',  ( -5.152983112885297217E-15, -6.594478602028688741, 10.23203630735471137 ) ) ;
#17393=ORIENTED_EDGE ( 'NONE', *, *, #162539, .F. ) ;
#17431=CARTESIAN_POINT ( 'NONE',  ( 6.661184041422462343, -7.645986912801310709, -6.773376349081635439 ) ) ;
#17451=ORIENTED_EDGE ( 'NONE', *, *, #129734, .F. ) ;
#17507=VERTEX_POINT ( 'NONE', #107428 ) ;
#17552=ORIENTED_EDGE ( 'NONE', *, *, #10791, .F. ) ;
#17564=CIRCLE ( 'NONE', #57048, 8.049999999999993605 ) ;
#17566=CARTESIAN_POINT ( 'NONE',  ( 9.499607930503637832, -9.902952869712851935, -0.08630915044579903772 ) ) ;
#17585=CARTESIAN_POINT ( 'NONE',  ( 0.002323312721274023267, -7.217450603046065893, 9.500350659417536647 ) ) ;
#17593=CARTESIAN_POINT ( 'NONE',  ( 0.000000000000000000, -9.063431457505059186, 0.000000000000000000 ) ) ;
#17595=CARTESIAN_POINT ( 'NONE',  ( 10.99945475518247129, -9.908704762181759662, -0.1095286008944305889 ) ) ;
#17597=( BOUNDED_SURFACE ( )  B_SPLINE_SURFACE ( 3, 2, ( 
 ( #55691, #105538, #171572 ),
 ( #23169, #167319, #18906 ),
 ( #89285, #84990, #151081 ),
 ( #52494, #53561, #134840 ),
 ( #118624, #119694, #9081 ),
 ( #43744, #59963, #142322 ),
 ( #143392, #206202, #157486 ),
 ( #42680, #12267, #176922 ) ),
 .UNSPECIFIED., .F., .F., .T. ) 
 B_SPLINE_SURFACE_WITH_KNOTS ( ( 4, 2, 2, 4 ),
 ( 3, 3 ),
 ( 5.421010862427522170E-20, 0.0004401918256850920631, 0.0006602877385276380946, 0.0008803836513701841261 ),
 ( 0.000000000000000000, 1.000000000000000000 ),
 .UNSPECIFIED. ) 
 GEOMETRIC_REPRESENTATION_ITEM ( )  RATIONAL_B_SPLINE_SURFACE ( (
 ( 1.000000000000000000, 0.6787756258918233865, 1.000000000000000000),
 ( 1.000000000000000000, 0.6284487096100427328, 1.000000000000000000),
 ( 1.000000000000000000, 0.5704014816683798950, 1.000000000000000000),
 ( 1.000000000000000000, 0.4882303283130677296, 1.000000000000000000),
 ( 1.000000000000000000, 0.4617370933884979434, 1.000000000000000000),
 ( 1.000000000000000000, 0.4222438920367950765, 1.000000000000000000),
 ( 1.000000000000000000, 0.4105126989450126884, 1.000000000000000000),
 ( 1.000000000000000000, 0.4127341956164993220, 1.000000000000000000) ) ) 
 REPRESENTATION_ITEM ( '' )  SURFACE ( )  );
#17623=ORIENTED_EDGE ( 'NONE', *, *, #138938, .T. ) ;
#17633=ADVANCED_FACE ( 'NONE', ( #156126 ), #188606, .T. ) ;
#17652=STYLED_ITEM ( 'NONE', ( #131077 ), #56893 ) ;
#17675=CARTESIAN_POINT ( 'NONE',  ( 1.786647480846655257E-05, -9.954793286625724491, 11.00029511060568588 ) ) ;
#17695=CARTESIAN_POINT ( 'NONE',  ( 2.373851744317274193, 1.000000000000000888, -11.76285798163019969 ) ) ;
#17720=VERTEX_POINT ( 'NONE', #169158 ) ;
#17725=CARTESIAN_POINT ( 'NONE',  ( 6.729185404178087637, -6.864242587301018439, 6.701130199342134830 ) ) ;
#17780=LINE ( 'NONE', #31942, #77910 ) ;
#17784=FILL_AREA_STYLE_COLOUR ( '', #197141 ) ;
#17828=CARTESIAN_POINT ( 'NONE',  ( 9.586610838029429260, -7.161464053357567749, -0.003376046620571135446 ) ) ;
#17854=CARTESIAN_POINT ( 'NONE',  ( 0.3728355200474325337, -6.583727468838304731, 9.609247538823966650 ) ) ;
#17859=CIRCLE ( 'NONE', #76645, 0.08000000000000020983 ) ;
#17881=CARTESIAN_POINT ( 'NONE',  ( 11.00020965659335204, -5.765528217051488546, 0.01167607004708704974 ) ) ;
#17892=PLANE ( 'NONE',  #138005 ) ;
#17904=CARTESIAN_POINT ( 'NONE',  ( 0.4382560683119269829, -7.666862915010147717, -10.99126615174920296 ) ) ;
#17921=EDGE_CURVE ( 'NONE', #125480, #146898, #157946, .T. ) ;
#17936=CARTESIAN_POINT ( 'NONE',  ( 0.000000000000000000, 0.000000000000000000, 0.000000000000000000 ) ) ;
#17978=CARTESIAN_POINT ( 'NONE',  ( 9.858406733136194415E-16, 3.000000000000002665, -8.050000000000000711 ) ) ;
#17989=CARTESIAN_POINT ( 'NONE',  ( 9.499668754385638181, -7.246166700194470067, 0.07933194154488365513 ) ) ;
#18033=VERTEX_POINT ( 'NONE', #59299 ) ;
#18041=CARTESIAN_POINT ( 'NONE',  ( -8.103009739378183696, -6.700000000000007283, 7.439168848973805481 ) ) ;
#18067=CARTESIAN_POINT ( 'NONE',  ( 0.4362825330288246928, -6.085430761754772711, 10.10516068267232548 ) ) ;
#18098=ORIENTED_EDGE ( 'NONE', *, *, #91149, .F. ) ;
#18103=AXIS2_PLACEMENT_3D ( 'NONE', #4931, #105708, #185836 ) ;
#18108=VERTEX_POINT ( 'NONE', #62973 ) ;
#18145=CARTESIAN_POINT ( 'NONE',  ( -6.650326532587143902, -8.038658175288281527, -6.784185045882105136 ) ) ;
#18206=CARTESIAN_POINT ( 'NONE',  ( 6.773846765317306229, -7.246166700180828535, -6.773846765317331986 ) ) ;
#18221=CARTESIAN_POINT ( 'NONE',  ( -9.578206920975032901, -9.954640969533237183, 0.1671882237015447359 ) ) ;
#18222=EDGE_CURVE ( 'NONE', #119302, #322, #213252, .T. ) ;
#18309=VECTOR ( 'NONE', #20813, 1000.000000000000000 ) ;
#18331=AXIS2_PLACEMENT_3D ( 'NONE', #204435, #183938, #153590 ) ;
#18334=( NAMED_UNIT ( * ) SI_UNIT ( $, .STERADIAN. ) SOLID_ANGLE_UNIT ( ) );
#18419=FACE_OUTER_BOUND ( 'NONE', #147294, .T. ) ;
#18482=CARTESIAN_POINT ( 'NONE',  ( -11.41267819554182950, 3.038492715500534569, 3.708203932499423594 ) ) ;
#18513=CARTESIAN_POINT ( 'NONE',  ( 11.41267819554178864, 3.038492715500545227, -3.708203932499494204 ) ) ;
#18521=VERTEX_POINT ( 'NONE', #86686 ) ;
#18568=CARTESIAN_POINT ( 'NONE',  ( 9.483599735403714703, -9.201296717416477478, -0.5591315121169913027 ) ) ;
#18574=CARTESIAN_POINT ( 'NONE',  ( -10.90726532705803820, -6.287979527546282199, 0.008173644115966051740 ) ) ;
#18581=DIRECTION ( 'NONE',  ( 0.000000000000000000, 0.000000000000000000, 1.000000000000000000 ) ) ;
#18612=DIRECTION ( 'NONE',  ( 0.000000000000000000, 0.000000000000000000, 1.000000000000000000 ) ) ;
#18617=EDGE_CURVE ( 'NONE', #212186, #201589, #173103, .T. ) ;
#18650=B_SPLINE_CURVE_WITH_KNOTS ( 'NONE', 3,
 ( #152052, #185594, #186666, #4686 ),
 .UNSPECIFIED., .F., .F.,
 ( 4, 4 ),
 ( 0.000000000000000000, 0.0004044236633723155756 ),
 .UNSPECIFIED. ) ;
#18666=CARTESIAN_POINT ( 'NONE',  ( 6.776593369755653740, -7.026643280347737885, 6.796618584847460731 ) ) ;
#18732=ADVANCED_FACE ( 'NONE', ( #41964 ), #178319, .F. ) ;
#18734=CARTESIAN_POINT ( 'NONE',  ( -9.499606442108966320, 7.849261790823902629, 0.08647222121513364890 ) ) ;
#18794=CARTESIAN_POINT ( 'NONE',  ( -6.640718169120819248, -6.363025497629810623, -7.257245574616625561 ) ) ;
#18839=DIRECTION ( 'NONE',  ( 0.000000000000000000, -1.000000000000000000, 0.000000000000000000 ) ) ;
#18860=CARTESIAN_POINT ( 'NONE',  ( 7.228805602686604992, -7.003075417673639613, 7.884707905546937567 ) ) ;
#18861=EDGE_CURVE ( 'NONE', #96467, #97798, #95943, .T. ) ;
#18876=ORIENTED_EDGE ( 'NONE', *, *, #195623, .T. ) ;
#18900=CARTESIAN_POINT ( 'NONE',  ( 9.499801640457391727, -7.008739397177219388, 0.06269018847620325130 ) ) ;
#18903=VERTEX_POINT ( 'NONE', #76565 ) ;
#18906=CARTESIAN_POINT ( 'NONE',  ( 6.672971353126269989, -7.009934032700107842, -6.761775799041030766 ) ) ;
#18954=CARTESIAN_POINT ( 'NONE',  ( 10.97093617010649780, -5.223179855898941959, -0.3663205537283247826 ) ) ;
#18970=EDGE_LOOP ( 'NONE', ( #148266, #98534, #188231, #16913, #112394 ) ) ;
#18977=FACE_OUTER_BOUND ( 'NONE', #208314, .T. ) ;
#18987=DIRECTION ( 'NONE',  ( 0.000000000000000000, 0.000000000000000000, 1.000000000000000000 ) ) ;
#19012=UNCERTAINTY_MEASURE_WITH_UNIT (LENGTH_MEASURE( 1.000000000000000082E-05 ), #20529, 'distance_accuracy_value', 'NONE');
#19047=CARTESIAN_POINT ( 'NONE',  ( -0.08058608058608696112, -9.999999999999994671, 10.99970480893081870 ) ) ;
#19069=VERTEX_POINT ( 'NONE', #79766 ) ;
#19082=CARTESIAN_POINT ( 'NONE',  ( 10.99574878476024153, -7.889012432655408524, -0.3098035853330123324 ) ) ;
#19144=B_SPLINE_CURVE_WITH_KNOTS ( 'NONE', 3,
 ( #186542, #185469, #38171, #8858, #103169, #169230, #152986, #207054, #107503, #86918, #89070, #56559, #40316, #72786, #104244, #136746 ),
 .UNSPECIFIED., .F., .F.,
 ( 4, 3, 3, 3, 3, 4 ),
 ( 0.000000000000000000, 3.357617230303705058E-05, 6.715207102180654238E-05, 0.0001007279560762661569, 0.0001343044553218104679, 0.0001562161319167434893 ),
 .UNSPECIFIED. ) ;
#19165=ORIENTED_EDGE ( 'NONE', *, *, #33910, .F. ) ;
#19184=CARTESIAN_POINT ( 'NONE',  ( -9.477100695693458476, -6.554910290221380720, 0.2834499523633453588 ) ) ;
#19185=ORIENTED_EDGE ( 'NONE', *, *, #166507, .F. ) ;
#19231=CARTESIAN_POINT ( 'NONE',  ( 9.579253414572376002, -9.994362535427860905, -0.1002978391578448342 ) ) ;
#19234=DIRECTION ( 'NONE',  ( -0.000000000000000000, -1.000000000000000000, -0.000000000000000000 ) ) ;
#19237=VERTEX_POINT ( 'NONE', #29966 ) ;
#19286=ORIENTED_EDGE ( 'NONE', *, *, #182418, .T. ) ;
#19316=FILL_AREA_STYLE_COLOUR ( '', #60442 ) ;
#19356=CARTESIAN_POINT ( 'NONE',  ( -0.09872732973945111401, -6.896119493545342038, -9.497255425109710103 ) ) ;
#19391=VERTEX_POINT ( 'NONE', #119796 ) ;
#19397=CARTESIAN_POINT ( 'NONE',  ( 9.132253115921068698, 1.016282880930313937, 8.222717639126729594 ) ) ;
#19402=CARTESIAN_POINT ( 'NONE',  ( 2.423460580168060652, 1.405705671057797312, -11.75284646727698679 ) ) ;
#19438=CARTESIAN_POINT ( 'NONE',  ( 0.03415196713897553082, -6.453216945989479036, 10.89423718502873939 ) ) ;
#19442=EDGE_CURVE ( 'NONE', #7171, #193389, #38817, .T. ) ;
#19447=CARTESIAN_POINT ( 'NONE',  ( 10.91804383151479740, -8.407420853759283830, -0.1905751639681655396 ) ) ;
#19449=CARTESIAN_POINT ( 'NONE',  ( 7.235142258280584215, -6.594478602024285152, 7.235142258280580663 ) ) ;
#19474=DIRECTION ( 'NONE',  ( 0.000000000000000000, 1.000000000000000000, 0.000000000000000000 ) ) ;
#19502=ORIENTED_EDGE ( 'NONE', *, *, #99329, .T. ) ;
#19507=CARTESIAN_POINT ( 'NONE',  ( 0.000000000000000000, -8.327195405469542067, 10.91970695577495931 ) ) ;
#19508=DIRECTION ( 'NONE',  ( 0.000000000000000000, -1.000000000000000000, 0.000000000000000000 ) ) ;
#19529=CARTESIAN_POINT ( 'NONE',  ( 0.07933194154487524519, 7.849261790823902629, 9.499668754385634628 ) ) ;
#19540=CARTESIAN_POINT ( 'NONE',  ( 0.000000000000000000, -9.006862915010128035, 0.000000000000000000 ) ) ;
#19541=DIRECTION ( 'NONE',  ( -0.7366372490352351976, 0.000000000000000000, 0.6762880771785058087 ) ) ;
#19558=ORIENTED_EDGE ( 'NONE', *, *, #130557, .T. ) ;
#19570=ADVANCED_FACE ( 'NONE', ( #152235, #153295 ), #72018, .F. ) ;
#19580=CARTESIAN_POINT ( 'NONE',  ( 7.730132016635857362, -5.756136661604687177, -7.730132016635878678 ) ) ;
#19596=ORIENTED_EDGE ( 'NONE', *, *, #214161, .T. ) ;
#19597=CARTESIAN_POINT ( 'NONE',  ( 10.07455280567994116, 1.264806443676223857, 6.263461699855335851 ) ) ;
#19639=CARTESIAN_POINT ( 'NONE',  ( -2.493461049780994365, 3.507114751586604129, 11.73081193161140590 ) ) ;
#19666=CARTESIAN_POINT ( 'NONE',  ( -7.722692672890413945, -6.459788825448667282, -7.834474503270543622 ) ) ;
#19702=CARTESIAN_POINT ( 'NONE',  ( 1.495620097461134202E-12, -5.796408561410189897, 10.41272866534516695 ) ) ;
#19703=ORIENTED_EDGE ( 'NONE', *, *, #10155, .T. ) ;
#19716=CARTESIAN_POINT ( 'NONE',  ( -6.505896022970769188, -8.148356111791729361, -6.958662999125635018 ) ) ;
#19736=FACE_OUTER_BOUND ( 'NONE', #93501, .T. ) ;
#19745=VECTOR ( 'NONE', #42572, 1000.000000000000000 ) ;
#19767=CARTESIAN_POINT ( 'NONE',  ( -9.495732322661975644, -8.202835266173753581, 0.2934966634902112514 ) ) ;
#19822=CARTESIAN_POINT ( 'NONE',  ( 0.08972248771634809550, -9.919998018256677597, 10.99963958991171786 ) ) ;
#19833=ORIENTED_EDGE ( 'NONE', *, *, #17156, .F. ) ;
#19876=CARTESIAN_POINT ( 'NONE',  ( 0.07933194154487524519, -7.246166700194011767, -9.499668754385622194 ) ) ;
#19920=SURFACE_STYLE_USAGE ( .BOTH. , #171516 ) ;
#19929=CARTESIAN_POINT ( 'NONE',  ( 2.474997580123494245, 0.9706168436483512130, -11.64394813633530923 ) ) ;
#19960=B_SPLINE_CURVE_WITH_KNOTS ( 'NONE', 3,
 ( #187798, #103363, #87107, #4751, #136943, #54610, #120758, #5826, #23150, #138009 ),
 .UNSPECIFIED., .F., .F.,
 ( 4, 2, 2, 2, 4 ),
 ( 0.000000000000000000, 0.0002598598948551708999, 0.0005197197897103416914, 0.0007795796845655125372, 0.001039439579420683383 ),
 .UNSPECIFIED. ) ;
#19970=EDGE_LOOP ( 'NONE', ( #174224, #38105, #87287 ) ) ;
#19986=CARTESIAN_POINT ( 'NONE',  ( 10.99036836684473073, -7.696788179137236341, -0.4651914231089532836 ) ) ;
#19987=CARTESIAN_POINT ( 'NONE',  ( 6.773846765307952822, -7.473374494058216300, -6.773846765307982132 ) ) ;
#20021=CARTESIAN_POINT ( 'NONE',  ( 10.96107445065239538, -5.401429653175719103, -0.1376292675369649998 ) ) ;
#20034=DIRECTION ( 'NONE',  ( 0.000000000000000000, 0.000000000000000000, 1.000000000000000000 ) ) ;
#20080=CARTESIAN_POINT ( 'NONE',  ( 10.44245235073003286, 1.000000000000000888, -5.695529491621821983 ) ) ;
#20145=CARTESIAN_POINT ( 'NONE',  ( 10.96075698767266893, -7.841077028191733689, -0.3746540212967842121 ) ) ;
#20170=ORIENTED_EDGE ( 'NONE', *, *, #140961, .T. ) ;
#20177=CARTESIAN_POINT ( 'NONE',  ( -7.788485247867485306, -6.306978362809775085, 7.768428355091874238 ) ) ;
#20213=DIRECTION ( 'NONE',  ( -0.7408284471490504952, 0.000000000000000000, 0.6716942845482061220 ) ) ;
#20217=CARTESIAN_POINT ( 'NONE',  ( 10.97058181929407716, -5.254568858751050620, -0.2903707658989311269 ) ) ;
#20225=ORIENTED_EDGE ( 'NONE', *, *, #60818, .F. ) ;
#20289=CARTESIAN_POINT ( 'NONE',  ( -6.773376349081642545, -7.645986912801316926, -6.661184041422457902 ) ) ;
#20338=EDGE_CURVE ( 'NONE', #209328, #195818, #50925, .T. ) ;
#20389=CARTESIAN_POINT ( 'NONE',  ( -9.536979704252539491, -7.995840219786908065, 0.1489494290324817893 ) ) ;
#20396=UNCERTAINTY_MEASURE_WITH_UNIT (LENGTH_MEASURE( 1.000000000000000082E-05 ), #111707, 'distance_accuracy_value', 'NONE');
#20408=CIRCLE ( 'NONE', #89561, 10.86343145750506700 ) ;
#20412=CARTESIAN_POINT ( 'NONE',  ( -5.204170427930421283E-15, -7.242250812739418286, -9.811039896441874575 ) ) ;
#20435=CARTESIAN_POINT ( 'NONE',  ( 0.000000000000000000, 0.000000000000000000, 0.000000000000000000 ) ) ;
#20459=ORIENTED_EDGE ( 'NONE', *, *, #188352, .F. ) ;
#20487=CARTESIAN_POINT ( 'NONE',  ( -3.672711609586798782E-15, -9.954379061088836522, -9.579665937615013505 ) ) ;
#20504=CARTESIAN_POINT ( 'NONE',  ( -6.992767129439147133, -7.336076765398686028, -7.649321060469615574 ) ) ;
#20529=( LENGTH_UNIT ( ) NAMED_UNIT ( * ) SI_UNIT ( .MILLI., .METRE. ) );
#20545=CARTESIAN_POINT ( 'NONE',  ( 10.71948157449259043, -8.605866298767898215, -0.1871092468795605146 ) ) ;
#20546=CARTESIAN_POINT ( 'NONE',  ( -6.636492533740866577E-13, -6.372041098632465150, -9.837588353259592466 ) ) ;
#20558=AXIS2_PLACEMENT_3D ( 'NONE', #194790, #81046, #109361 ) ;
#20566=ORIENTED_EDGE ( 'NONE', *, *, #140442, .F. ) ;
#20573=CARTESIAN_POINT ( 'NONE',  ( -0.4356160240586506860, -9.063431457505064515, 9.626717610576623230 ) ) ;
#20615=ORIENTED_EDGE ( 'NONE', *, *, #24925, .T. ) ;
#20634=CARTESIAN_POINT ( 'NONE',  ( -1.138412281109779656E-15, -6.920331743278516967, -9.905860218026836250 ) ) ;
#20645=AXIS2_PLACEMENT_3D ( 'NONE', #208782, #174200, #126573 ) ;
#20668=( BOUNDED_SURFACE ( )  B_SPLINE_SURFACE ( 3, 2, ( 
 ( #189811, #39301, #7850 ),
 ( #161322, #187671, #173604 ),
 ( #145104, #5694, #121708 ),
 ( #127847, #211108, #90204 ),
 ( #105396, #77924, #203907 ),
 ( #112632, #62733, #128893 ),
 ( #206056, #25176, #29184 ),
 ( #194874, #106489, #88053 ) ),
 .UNSPECIFIED., .F., .F., .T. ) 
 B_SPLINE_SURFACE_WITH_KNOTS ( ( 4, 2, 2, 4 ),
 ( 3, 3 ),
 ( 0.000000000000000000, 0.0005123566476021777739, 0.0007685349714032666067, 0.001024713295204355548 ),
 ( 0.000000000000000000, 1.000000000000000000 ),
 .UNSPECIFIED. ) 
 GEOMETRIC_REPRESENTATION_ITEM ( )  RATIONAL_B_SPLINE_SURFACE ( (
 ( 1.000000000000000000, 0.7100530722026823227, 1.000000000000000000),
 ( 1.000000000000000000, 0.7667719522827138867, 1.000000000000000000),
 ( 1.000000000000000000, 0.8160440554223366005, 1.000000000000000000),
 ( 1.000000000000000000, 0.8737249316769485352, 1.000000000000000000),
 ( 1.000000000000000000, 0.8903164784319946845, 1.000000000000000000),
 ( 1.000000000000000000, 0.9150853305241298807, 1.000000000000000000),
 ( 1.000000000000000000, 0.9227739504732653808, 1.000000000000000000),
 ( 1.000000000000000000, 0.9238795325112855172, 1.000000000000000000) ) ) 
 REPRESENTATION_ITEM ( '' )  SURFACE ( )  );
#20677=CARTESIAN_POINT ( 'NONE',  ( -7.968353659517141807, -5.197284395437294258, 7.583532603600725785 ) ) ;
#20690=CARTESIAN_POINT ( 'NONE',  ( 9.855659161987905037, -6.334709917115484146, -0.4359479416626658166 ) ) ;
#20696=CARTESIAN_POINT ( 'NONE',  ( -10.88932262995847822, -6.511064858252409771, 0.06814526087293559797 ) ) ;
#20712=STYLED_ITEM ( 'NONE', ( #207806 ), #160339 ) ;
#20717=CARTESIAN_POINT ( 'NONE',  ( -8.758160245763034979, 1.972237431423827347, -7.885882905893924821 ) ) ;
#20743=ORIENTED_EDGE ( 'NONE', *, *, #110343, .T. ) ;
#20747=DIRECTION ( 'NONE',  ( 0.000000000000000000, 0.000000000000000000, 1.000000000000000000 ) ) ;
#20749=ADVANCED_FACE ( 'NONE', ( #63784 ), #9490, .T. ) ;
#20753=CARTESIAN_POINT ( 'NONE',  ( -2.331034670843834533E-15, -6.105866302529035394, 10.72111444838893135 ) ) ;
#20763=CARTESIAN_POINT ( 'NONE',  ( -9.093502852636577316, 1.000000000000000888, -7.666967846417613863 ) ) ;
#20789=CARTESIAN_POINT ( 'NONE',  ( 6.400381488218092052, -6.708819892820498509, 7.008396152629734033 ) ) ;
#20797=CARTESIAN_POINT ( 'NONE',  ( -8.694134400161971216E-15, 3.603753425775781505, -11.89624657422419673 ) ) ;
#20800=CARTESIAN_POINT ( 'NONE',  ( 6.825879202496176745, -6.900108348306368988, -6.758184431511345736 ) ) ;
#20813=DIRECTION ( 'NONE',  ( 0.000000000000000000, 1.000000000000000000, 0.000000000000000000 ) ) ;
#20821=CARTESIAN_POINT ( 'NONE',  ( 7.792125355486789751, -6.646943093533971947, -7.591565991045878370 ) ) ;
#20833=CARTESIAN_POINT ( 'NONE',  ( 0.07538891330674882263, -7.154544010627095219, -9.499700864329891914 ) ) ;
#20848=EDGE_LOOP ( 'NONE', ( #208730, #207265, #122997, #16586 ) ) ;
#20857=LINE ( 'NONE', #18734, #7536 ) ;
#20872=CARTESIAN_POINT ( 'NONE',  ( 0.000000000000000000, 0.000000000000000000, 0.000000000000000000 ) ) ;
#20883=CARTESIAN_POINT ( 'NONE',  ( -3.469446951953614189E-15, 3.507114751586604129, 11.99288524841339054 ) ) ;
#20926=DIRECTION ( 'NONE',  ( 0.000000000000000000, 0.000000000000000000, -1.000000000000000000 ) ) ;
#20937=DIRECTION ( 'NONE',  ( -0.000000000000000000, -1.000000000000000000, -0.000000000000000000 ) ) ;
#20950=CARTESIAN_POINT ( 'NONE',  ( 7.553974597844359096, -6.709380320845432344, 7.821934338880126347 ) ) ;
#21002=LINE ( 'NONE', #120750, #100658 ) ;
#21010=EDGE_LOOP ( 'NONE', ( #139408, #208304, #1303, #139435 ) ) ;
#21022=CARTESIAN_POINT ( 'NONE',  ( 9.500385102287568273, -7.162053774861992572, -0.01083140255524948393 ) ) ;
#21039=CARTESIAN_POINT ( 'NONE',  ( -6.558483974469827338, -6.776276029125435585, -6.864213375409891071 ) ) ;
#21047=CARTESIAN_POINT ( 'NONE',  ( 0.05436647835300240789, -9.474608021433732929, 9.500000000000147438 ) ) ;
#21086=VERTEX_POINT ( 'NONE', #69095 ) ;
#21171=DIRECTION ( 'NONE',  ( 0.000000000000000000, 0.000000000000000000, 1.000000000000000000 ) ) ;
#21181=FILL_AREA_STYLE ('',( #184761 ) ) ;
#21183=ORIENTED_EDGE ( 'NONE', *, *, #89270, .F. ) ;
#21185=VERTEX_POINT ( 'NONE', #153585 ) ;
#21188=CARTESIAN_POINT ( 'NONE',  ( -9.886825906824906696, 3.934660213246447658, -6.000867881395567593 ) ) ;
#21197=FACE_OUTER_BOUND ( 'NONE', #48616, .T. ) ;
#21210=CARTESIAN_POINT ( 'NONE',  ( 0.4644097342742965484, -8.233137084989849086, 9.488641820551103834 ) ) ;
#21223=VERTEX_POINT ( 'NONE', #204430 ) ;
#21258=CARTESIAN_POINT ( 'NONE',  ( -10.91828647086820858, -9.953005061877725268, 0.1753736836078399752 ) ) ;
#21271=CARTESIAN_POINT ( 'NONE',  ( 2.069187086148546406, 1.970899860167973694, -11.59589854942352893 ) ) ;
#21291=STYLED_ITEM ( 'NONE', ( #187970 ), #172604 ) ;
#21316=CARTESIAN_POINT ( 'NONE',  ( 0.000000000000000000, -7.154544010627095219, 0.000000000000000000 ) ) ;
#21354=CIRCLE ( 'NONE', #66347, 0.08000000000000020983 ) ;
#21366=ORIENTED_EDGE ( 'NONE', *, *, #101879, .T. ) ;
#21438=CARTESIAN_POINT ( 'NONE',  ( -9.495223711095324148, -8.169755926620650754, 0.3080734816350879646 ) ) ;
#21461=CARTESIAN_POINT ( 'NONE',  ( -0.4355862708379995563, -6.583980363595115293, -9.606148981167580203 ) ) ;
#21471=CARTESIAN_POINT ( 'NONE',  ( -0.1589091098076596542, -6.723650695528558430, -9.611540586923219109 ) ) ;
#21525=FACE_OUTER_BOUND ( 'NONE', #20848, .T. ) ;
#21533=DIRECTION ( 'NONE',  ( -0.000000000000000000, 1.000000000000000000, -0.000000000000000000 ) ) ;
#21589=CARTESIAN_POINT ( 'NONE',  ( 9.818302567231148359, -8.862962251182139539, -0.6073963244357859503 ) ) ;
#21616=CARTESIAN_POINT ( 'NONE',  ( -10.93186801223271409, -5.758458176070771373, 3.167056189783827390E-15 ) ) ;
#21617=ORIENTED_EDGE ( 'NONE', *, *, #95057, .T. ) ;
#21618=CARTESIAN_POINT ( 'NONE',  ( -0.3931996164520709103, -9.201308816821677894, 9.491928691056637390 ) ) ;
#21635=CARTESIAN_POINT ( 'NONE',  ( 9.488641820551102057, -8.233137084989836652, -0.4644097342743017665 ) ) ;
#21682=CARTESIAN_POINT ( 'NONE',  ( -6.672971353125990213, -7.009934032700016360, 6.761775799041313206 ) ) ;
#21707=ADVANCED_FACE ( 'NONE', ( #137383 ), #179480, .T. ) ;
#21716=FACE_OUTER_BOUND ( 'NONE', #12497, .T. ) ;
#21725=EDGE_LOOP ( 'NONE', ( #131808, #96762, #164675, #104687 ) ) ;
#21748=AXIS2_PLACEMENT_3D ( 'NONE', #49886, #34688, #181997 ) ;
#21750=CARTESIAN_POINT ( 'NONE',  ( -10.85353573482952072, -6.836568542495036205, 0.4635785636673775967 ) ) ;
#21780=EDGE_LOOP ( 'NONE', ( #81064, #36126, #92101, #200527 ) ) ;
#21791=CARTESIAN_POINT ( 'NONE',  ( 10.16279779336423772, 3.829867255648782720, -5.736760595005132579 ) ) ;
#21808=CARTESIAN_POINT ( 'NONE',  ( -2.331034670843834533E-15, -7.256398209935973398, 9.569423160902228886 ) ) ;
#21810=ORIENTED_EDGE ( 'NONE', *, *, #166214, .F. ) ;
#21817=CARTESIAN_POINT ( 'NONE',  ( 0.3689019803512919582, -6.583711573986999355, 9.609441814500817358 ) ) ;
#21823=CARTESIAN_POINT ( 'NONE',  ( -10.99960280095053378, -9.919999999999998153, 0.09350563796403016381 ) ) ;
#21826=B_SPLINE_CURVE_WITH_KNOTS ( 'NONE', 3,
 ( #41392, #25104, #54423, #7778, #20821, #137819, #74937, #119482 ),
 .UNSPECIFIED., .F., .F.,
 ( 4, 2, 2, 4 ),
 ( 6.987453456569233415E-16, 0.0002305131806122158098, 0.0004610263612237329054, 0.0009220527224467680184 ),
 .UNSPECIFIED. ) ;
#21855=DIRECTION ( 'NONE',  ( 0.9992060137953822085, -3.484297484817962848E-16, -0.03984146075563036599 ) ) ;
#21865=STYLED_ITEM ( 'NONE', ( #160832 ), #81437 ) ;
#21878=CARTESIAN_POINT ( 'NONE',  ( 7.235142258280562899, -6.594478602024301139, -7.235142258280586880 ) ) ;
#21894=EDGE_CURVE ( 'NONE', #33092, #113056, #185941, .T. ) ;
#21906=ORIENTED_EDGE ( 'NONE', *, *, #15354, .F. ) ;
#21939=( NAMED_UNIT ( * ) PLANE_ANGLE_UNIT ( ) SI_UNIT ( $, .RADIAN. ) );
#21943=FILL_AREA_STYLE_COLOUR ( '', #164606 ) ;
#22012=CARTESIAN_POINT ( 'NONE',  ( -6.717748655459615748, -7.246166700180828535, 6.717748655459638840 ) ) ;
#22028=CIRCLE ( 'NONE', #70426, 0.07999999999999993228 ) ;
#22041=CARTESIAN_POINT ( 'NONE',  ( -0.08058608058608696112, -6.134628647623513231, 10.99970480893081870 ) ) ;
#22055=DIRECTION ( 'NONE',  ( 0.000000000000000000, 0.000000000000000000, -1.000000000000000000 ) ) ;
#22062=CARTESIAN_POINT ( 'NONE',  ( -0.1412570932018016034, -6.646059016331633096, -10.87798840695972657 ) ) ;
#22098=CARTESIAN_POINT ( 'NONE',  ( -6.429544252029797846, -6.709867743870402634, -6.981856502304072620 ) ) ;
#22107=CARTESIAN_POINT ( 'NONE',  ( 7.846302513400016387, -6.700642373080272662, -7.709579522695857889 ) ) ;
#22111=ADVANCED_FACE ( 'NONE', ( #208744 ), #175220, .T. ) ;
#22148=ORIENTED_EDGE ( 'NONE', *, *, #75556, .F. ) ;
#22175=EDGE_CURVE ( 'NONE', #119302, #182623, #180980, .T. ) ;
#22193=B_SPLINE_CURVE_WITH_KNOTS ( 'NONE', 3,
 ( #89068, #154057, #73867, #41390 ),
 .UNSPECIFIED., .F., .F.,
 ( 4, 4 ),
 ( 0.000000000000000000, 6.033646489354490427E-05 ),
 .UNSPECIFIED. ) ;
#22222=CARTESIAN_POINT ( 'NONE',  ( -0.09924927195301232186, -9.920000000000094076, -10.99955234463955556 ) ) ;
#22264=CARTESIAN_POINT ( 'NONE',  ( 10.93053916617009413, -8.254340240174414589, -0.1907932708458892346 ) ) ;
#22301=CARTESIAN_POINT ( 'NONE',  ( -9.617648866954029430, -9.063431457505044975, 0.6035590660249372519 ) ) ;
#22326=CIRCLE ( 'NONE', #84509, 0.08000000000000050127 ) ;
#22335=ORIENTED_EDGE ( 'NONE', *, *, #201684, .T. ) ;
#22345=AXIS2_PLACEMENT_3D ( 'NONE', #96853, #63254, #82693 ) ;
#22380=B_SPLINE_CURVE_WITH_KNOTS ( 'NONE', 3,
 ( #117514, #18860, #84945, #186704, #152090, #102260, #118577 ),
 .UNSPECIFIED., .F., .F.,
 ( 4, 3, 4 ),
 ( 0.0001932293135873427547, 0.0009000000018422016053, 0.002089330742406778334 ),
 .UNSPECIFIED. ) ;
#22384=B_SPLINE_CURVE_WITH_KNOTS ( 'NONE', 3,
 ( #114443, #33121, #133855, #199865, #16843, #82925, #148998, #205192 ),
 .UNSPECIFIED., .F., .F.,
 ( 4, 2, 2, 4 ),
 ( 1.138412281109825108E-18, 0.0002224730689913802315, 0.0004449461379827593247, 0.0008898922759655175652 ),
 .UNSPECIFIED. ) ;
#22398=ORIENTED_EDGE ( 'NONE', *, *, #188204, .F. ) ;
#22417=CARTESIAN_POINT ( 'NONE',  ( -6.784185045882110465, -8.038658175288270868, 6.650326532587137685 ) ) ;
#22487=CARTESIAN_POINT ( 'NONE',  ( 0.000000000000000000, 0.9200000000000041478, 0.000000000000000000 ) ) ;
#22503=DIRECTION ( 'NONE',  ( 0.04888523518676873847, 0.000000000000000000, 0.9988044021632734859 ) ) ;
#22504=CARTESIAN_POINT ( 'NONE',  ( 1.423015351387224570E-15, 0.9706168436483911810, -11.90408086427858692 ) ) ;
#22509=ORIENTED_EDGE ( 'NONE', *, *, #110743, .F. ) ;
#22513=CARTESIAN_POINT ( 'NONE',  ( -9.492905263954453332, -8.233136995002796610, 0.3773006915670363282 ) ) ;
#22521=PRESENTATION_STYLE_ASSIGNMENT (( #170924 ) ) ;
#22530=CIRCLE ( 'NONE', #29372, 9.479622692290801567 ) ;
#22536=EDGE_CURVE ( 'NONE', #22857, #53554, #210687, .T. ) ;
#22540=CARTESIAN_POINT ( 'NONE',  ( 7.752014238602739730E-16, 0.03624871340549007392, 6.329999999999995630 ) ) ;
#22552=CARTESIAN_POINT ( 'NONE',  ( -0.01083140255525823388, -7.162053774861992572, -9.500385102287555839 ) ) ;
#22562=FILL_AREA_STYLE_COLOUR ( '', #27621 ) ;
#22586=ORIENTED_EDGE ( 'NONE', *, *, #169387, .F. ) ;
#22591=ORIENTED_EDGE ( 'NONE', *, *, #42234, .F. ) ;
#22605=DIRECTION ( 'NONE',  ( 0.000000000000000000, -1.000000000000000000, 0.000000000000000000 ) ) ;
#22621=CARTESIAN_POINT ( 'NONE',  ( 7.952857047017175773, -6.836289462023034780, -7.401194801147395808 ) ) ;
#22635=STYLED_ITEM ( 'NONE', ( #29335 ), #121837 ) ;
#22661=CARTESIAN_POINT ( 'NONE',  ( -9.837588353263715391, -6.372041098637188483, 1.678902898539189045E-12 ) ) ;
#22667=ORIENTED_EDGE ( 'NONE', *, *, #100462, .F. ) ;
#22673=AXIS2_PLACEMENT_3D ( 'NONE', #39160, #102025, #167030 ) ;
#22727=CARTESIAN_POINT ( 'NONE',  ( -7.649321060469629785, -7.336076765398686028, 6.992767129439145357 ) ) ;
#22756=B_SPLINE_CURVE_WITH_KNOTS ( 'NONE', 3,
 ( #192703, #96317, #193781, #95253 ),
 .UNSPECIFIED., .F., .F.,
 ( 4, 4 ),
 ( 0.000000000000000000, 8.505390838610418455E-05 ),
 .UNSPECIFIED. ) ;
#22759=CARTESIAN_POINT ( 'NONE',  ( 7.747753938335137924, -5.575271019048081200, -7.808923410443490809 ) ) ;
#22784=CARTESIAN_POINT ( 'NONE',  ( 2.494940289813108780, 3.447199233515649386, -11.73777120880564695 ) ) ;
#22796=MECHANICAL_DESIGN_GEOMETRIC_PRESENTATION_REPRESENTATION('',(#29641),#71185);
#22805=CARTESIAN_POINT ( 'NONE',  ( -7.721398836998369042, -5.907420853759296264, 7.721398836998396575 ) ) ;
#22857=VERTEX_POINT ( 'NONE', #115581 ) ;
#22883=ORIENTED_EDGE ( 'NONE', *, *, #105983, .F. ) ;
#22889=CARTESIAN_POINT ( 'NONE',  ( 0.000000000000000000, -2.000000000000001776, 10.91999999999999105 ) ) ;
#22891=CARTESIAN_POINT ( 'NONE',  ( 0.01387835396682936609, -7.030163990561721477, 9.597420367780074457 ) ) ;
#22901=DIRECTION ( 'NONE',  ( 0.06183953750878252997, 0.9962285034897218061, 0.06086575749408946329 ) ) ;
#22922=CARTESIAN_POINT ( 'NONE',  ( 6.653311379900189948, -6.675176078274398961, 6.940534579975176754 ) ) ;
#22930=CARTESIAN_POINT ( 'NONE',  ( 0.000000000000000000, 1.000000000000000888, 0.000000000000000000 ) ) ;
#22956=DIRECTION ( 'NONE',  ( 0.000000000000000000, 1.000000000000000000, 0.000000000000000000 ) ) ;
#23013=FACE_OUTER_BOUND ( 'NONE', #135708, .T. ) ;
#23063=CARTESIAN_POINT ( 'NONE',  ( 6.855650617048460127, -7.357813805523313988, 6.855650617048437923 ) ) ;
#23073=DIRECTION ( 'NONE',  ( 0.000000000000000000, 1.000000000000000000, 0.000000000000000000 ) ) ;
#23076=SURFACE_SIDE_STYLE ('',( #107622 ) ) ;
#23077=DIRECTION ( 'NONE',  ( -0.9989735196462988798, 0.000000000000000000, 0.04529798058948708572 ) ) ;
#23111=CARTESIAN_POINT ( 'NONE',  ( 0.000000000000000000, 0.000000000000000000, 0.000000000000000000 ) ) ;
#23118=DIRECTION ( 'NONE',  ( -0.9999655912483514930, 0.000000000000000000, 0.008295560218254021193 ) ) ;
#23134=ORIENTED_EDGE ( 'NONE', *, *, #6116, .F. ) ;
#23150=CARTESIAN_POINT ( 'NONE',  ( -10.99970480893082403, -6.221252899067775566, -0.08058608058607830138 ) ) ;
#23154=CIRCLE ( 'NONE', #36941, 9.499999999999992895 ) ;
#23169=CARTESIAN_POINT ( 'NONE',  ( 6.796618584847125000, -7.026643280347811604, -6.776593369755265606 ) ) ;
#23175=CARTESIAN_POINT ( 'NONE',  ( 7.547231044119296683, -5.251137252134833844, 7.967649405165770915 ) ) ;
#23177=CARTESIAN_POINT ( 'NONE',  ( 10.98194350564910415, -7.666862915010147717, -0.6300133639306100264 ) ) ;
#23186=CARTESIAN_POINT ( 'NONE',  ( 0.01424860406314341042, -7.025535116234668642, 9.597801448741886787 ) ) ;
#23203=ADVANCED_FACE ( 'NONE', ( #3611 ), #72444, .T. ) ;
#23227=CARTESIAN_POINT ( 'NONE',  ( -0.4356160240586524068, -9.063431457505059186, 9.626717610576628559 ) ) ;
#23341=CARTESIAN_POINT ( 'NONE',  ( -9.499633409936905082, -9.910600865424404660, 0.08345703571627748063 ) ) ;
#23342=CARTESIAN_POINT ( 'NONE',  ( 10.99931799034184365, -8.075210796978272043, -0.1485693272543584520 ) ) ;
#23354=EDGE_CURVE ( 'NONE', #193316, #182484, #145013, .T. ) ;
#23378=DIRECTION ( 'NONE',  ( 0.000000000000000000, 1.000000000000000000, 0.000000000000000000 ) ) ;
#23443=CIRCLE ( 'NONE', #144580, 9.499999999999992895 ) ;
#23464=B_SPLINE_CURVE_WITH_KNOTS ( 'NONE', 3,
 ( #210014, #128868, #174366, #45424, #61656, #107274, #60583, #8630, #10755, #192701 ),
 .UNSPECIFIED., .F., .F.,
 ( 4, 2, 2, 2, 4 ),
 ( 0.000000000000000000, 0.0002216178067634668662, 0.0004432356135269337324, 0.0006648534202904005444, 0.0008864712270538674648 ),
 .UNSPECIFIED. ) ;
#23545=DIRECTION ( 'NONE',  ( -1.000000000000000000, 0.000000000000000000, 0.000000000000000000 ) ) ;
#23550=ORIENTED_EDGE ( 'NONE', *, *, #42077, .T. ) ;
#23569=STYLED_ITEM ( 'NONE', ( #161685 ), #5413 ) ;
#23578=ORIENTED_EDGE ( 'NONE', *, *, #101879, .F. ) ;
#23597=( NAMED_UNIT ( * ) PLANE_ANGLE_UNIT ( ) SI_UNIT ( $, .RADIAN. ) );
#23625=B_SPLINE_CURVE_WITH_KNOTS ( 'NONE', 3,
 ( #119420, #22891, #186475, #54363, #103109, #170232, #21817, #5564 ),
 .UNSPECIFIED., .F., .F.,
 ( 4, 2, 2, 4 ),
 ( 0.000000000000000000, 0.0003954713701971529841, 0.0005932070552957304519, 0.0007909427403943080281 ),
 .UNSPECIFIED. ) ;
#23684=SURFACE_STYLE_USAGE ( .BOTH. , #190447 ) ;
#23706=CIRCLE ( 'NONE', #158552, 10.97656854249491509 ) ;
#23712=ORIENTED_EDGE ( 'NONE', *, *, #204878, .T. ) ;
#23715=CARTESIAN_POINT ( 'NONE',  ( 10.95632728729436067, -7.911711732698780253, -0.3221646467111924927 ) ) ;
#23725=DIRECTION ( 'NONE',  ( 0.000000000000000000, 0.000000000000000000, 1.000000000000000000 ) ) ;
#23733=CARTESIAN_POINT ( 'NONE',  ( -6.932145363377542502, -8.169775483750512990, 6.496114076516009916 ) ) ;
#23741=LINE ( 'NONE', #205688, #147056 ) ;
#23749=CARTESIAN_POINT ( 'NONE',  ( 10.41114276008972617, -8.296408557652583227, -0.1817271728525790275 ) ) ;
#23754=CARTESIAN_POINT ( 'NONE',  ( 0.2887529476172369103, 1.000000000000000888, -11.89119375935163880 ) ) ;
#23794=UNCERTAINTY_MEASURE_WITH_UNIT (LENGTH_MEASURE( 1.000000000000000082E-05 ), #120191, 'distance_accuracy_value', 'NONE');
#23859=ORIENTED_EDGE ( 'NONE', *, *, #105774, .T. ) ;
#23870=CARTESIAN_POINT ( 'NONE',  ( -0.003376046620571447263, -7.161464053357565973, -9.586610838029429260 ) ) ;
#23897=CARTESIAN_POINT ( 'NONE',  ( 9.549252947205625119, -7.850763007174478503, -0.06856108760741426444 ) ) ;
#23924=CARTESIAN_POINT ( 'NONE',  ( -8.912450614902597934, 3.507114751586604129, -8.024806578263023127 ) ) ;
#23926=CARTESIAN_POINT ( 'NONE',  ( -7.565242077046479885, -6.863172033215950485, -7.985752187169511629 ) ) ;
#23934=B_SPLINE_CURVE_WITH_KNOTS ( 'NONE', 3,
 ( #155014, #59636, #72680, #205881, #57515, #26062 ),
 .UNSPECIFIED., .F., .F.,
 ( 4, 2, 4 ),
 ( 0.0004044236633723155756, 0.0006920484658239215488, 0.0009796732682755275763 ),
 .UNSPECIFIED. ) ;
#24009=CARTESIAN_POINT ( 'NONE',  ( 0.000000000000000000, -6.527411821100059797, 0.000000000000000000 ) ) ;
#24097=SURFACE_STYLE_FILL_AREA ( #106484 ) ;
#24121=MECHANICAL_DESIGN_GEOMETRIC_PRESENTATION_REPRESENTATION('',(#107226),#145249);
#24175=CARTESIAN_POINT ( 'NONE',  ( -0.03750003396568979408, -9.978860739388867529, -10.91964959838800731 ) ) ;
#24201=CARTESIAN_POINT ( 'NONE',  ( 10.91804383151492530, -9.900000000000074962, -0.1905751639682747856 ) ) ;
#24211=CARTESIAN_POINT ( 'NONE',  ( -1.760028585276028923E-15, -6.211932585243245875, -10.91339599544321537 ) ) ;
#24232=ORIENTED_EDGE ( 'NONE', *, *, #184591, .T. ) ;
#24245=CARTESIAN_POINT ( 'NONE',  ( 7.834948807407927873, -5.743759731405710056, 7.720982915749591058 ) ) ;
#24257=CARTESIAN_POINT ( 'NONE',  ( 7.887197531381540117, -6.766388843766935501, -7.667935170093256758 ) ) ;
#24271=CARTESIAN_POINT ( 'NONE',  ( -0.4642244361878701819, -7.321523296574937056, -10.36809559534895975 ) ) ;
#24302=ORIENTED_EDGE ( 'NONE', *, *, #176359, .F. ) ;
#24308=PRESENTATION_STYLE_ASSIGNMENT (( #2715 ) ) ;
#24315=CARTESIAN_POINT ( 'NONE',  ( -10.99740610014212550, -6.654245765634820842, 0.2680151545362552401 ) ) ;
#24318=( NAMED_UNIT ( * ) PLANE_ANGLE_UNIT ( ) SI_UNIT ( $, .RADIAN. ) );
#24331=DIRECTION ( 'NONE',  ( 0.000000000000000000, 0.000000000000000000, 1.000000000000000000 ) ) ;
#24373=ORIENTED_EDGE ( 'NONE', *, *, #156157, .F. ) ;
#24403=CARTESIAN_POINT ( 'NONE',  ( -9.499656837482767457, -9.914216672575012268, 0.08076498840997262119 ) ) ;
#24427=DIRECTION ( 'NONE',  ( -0.7347175152297782397, 3.929830605827906454E-15, 0.6783731810844091381 ) ) ;
#24452=LINE ( 'NONE', #123153, #165063 ) ;
#24470=ORIENTED_EDGE ( 'NONE', *, *, #51899, .F. ) ;
#24477=DIRECTION ( 'NONE',  ( 0.000000000000000000, 1.000000000000000000, 0.000000000000000000 ) ) ;
#24478=VERTEX_POINT ( 'NONE', #101142 ) ;
#24519=CARTESIAN_POINT ( 'NONE',  ( -9.567202289542830584, -7.627132808484212489, 0.008219159353564688131 ) ) ;
#24520=CARTESIAN_POINT ( 'NONE',  ( -0.2534910766302378438, 3.934660213246439220, 11.56267633880227130 ) ) ;
#24530=CARTESIAN_POINT ( 'NONE',  ( 0.000000000000000000, 0.9200000000000041478, 6.249999999999995559 ) ) ;
#24569=CARTESIAN_POINT ( 'NONE',  ( 0.08058608058607655278, -9.900000000000005684, 10.99970480893082225 ) ) ;
#24583=ORIENTED_EDGE ( 'NONE', *, *, #115695, .T. ) ;
#24647=CARTESIAN_POINT ( 'NONE',  ( 0.3870774458628380987, 0.9691415390508764105, -11.89165654491649526 ) ) ;
#24658=DIRECTION ( 'NONE',  ( -0.9989777552170296948, -3.541417115716614946E-16, -0.04520447523801517098 ) ) ;
#24664=CARTESIAN_POINT ( 'NONE',  ( 10.91893890296302416, -9.990657656777852225, -0.1342453211083859954 ) ) ;
#24665=FACE_OUTER_BOUND ( 'NONE', #156276, .T. ) ;
#24704=CARTESIAN_POINT ( 'NONE',  ( -9.481348452320373710, -9.006862915010128035, 0.5950054837411746789 ) ) ;
#24712=DIRECTION ( 'NONE',  ( 0.000000000000000000, 0.000000000000000000, 1.000000000000000000 ) ) ;
#24764=CARTESIAN_POINT ( 'NONE',  ( -7.664830294503444996, -6.134628647623485698, 7.777967379493320621 ) ) ;
#24797=CARTESIAN_POINT ( 'NONE',  ( -6.849430810391480939, -7.996947095390788185, 6.637758778446722907 ) ) ;
#24807=CARTESIAN_POINT ( 'NONE',  ( 8.917737905728806425, 4.000000000000003553, 8.029567276306217138 ) ) ;
#24820=CARTESIAN_POINT ( 'NONE',  ( 7.446209719563365859, -5.223431457505076203, 8.064677165291195493 ) ) ;
#24825=B_SPLINE_CURVE_WITH_KNOTS ( 'NONE', 3,
 ( #48065, #115232, #133588, #167123, #212646, #118428, #36033 ),
 .UNSPECIFIED., .F., .F.,
 ( 4, 3, 4 ),
 ( 0.000000000000000000, 0.0008000000000005100470, 0.002977368225425562533 ),
 .UNSPECIFIED. ) ;
#24836=CARTESIAN_POINT ( 'NONE',  ( -10.85075961359308216, 3.974415841077576061, 3.932216895623811936 ) ) ;
#24871=DIRECTION ( 'NONE',  ( 0.000000000000000000, 0.000000000000000000, -1.000000000000000000 ) ) ;
#24881=PLANE ( 'NONE',  #54202 ) ;
#24887=ORIENTED_EDGE ( 'NONE', *, *, #107493, .T. ) ;
#24913=UNCERTAINTY_MEASURE_WITH_UNIT (LENGTH_MEASURE( 1.000000000000000082E-05 ), #170060, 'distance_accuracy_value', 'NONE');
#24924=ORIENTED_EDGE ( 'NONE', *, *, #17272, .T. ) ;
#24925=EDGE_CURVE ( 'NONE', #71638, #155393, #33257, .T. ) ;
#24928=COLOUR_RGB ( '', 0.40784314, 0.44705882, 0.49803922) ;
#24941=CARTESIAN_POINT ( 'NONE',  ( 0.000000000000000000, -6.527411821100059797, 0.000000000000000000 ) ) ;
#24984=CARTESIAN_POINT ( 'NONE',  ( 0.1236583036082015280, 1.000000000000000888, -11.99936284241577233 ) ) ;
#25007=CARTESIAN_POINT ( 'NONE',  ( 0.4330238300980764898, -6.527411821100045586, 9.549638505170038982 ) ) ;
#25043=( NAMED_UNIT ( * ) PLANE_ANGLE_UNIT ( ) SI_UNIT ( $, .RADIAN. ) );
#25069=EDGE_LOOP ( 'NONE', ( #86281, #156172, #1583, #58580 ) ) ;
#25070=CARTESIAN_POINT ( 'NONE',  ( -9.579603127937250662, -9.900000000000005684, 0.08720040834116031536 ) ) ;
#25104=CARTESIAN_POINT ( 'NONE',  ( 7.949604103952363054, -6.836271202499947464, -7.404765023120915224 ) ) ;
#25109=EDGE_CURVE ( 'NONE', #96541, #14256, #110828, .T. ) ;
#25147=AXIS2_PLACEMENT_3D ( 'NONE', #65891, #98431, #213222 ) ;
#25176=CARTESIAN_POINT ( 'NONE',  ( -0.3846410972798977590, -8.199730735666003412, -9.492545994385777064 ) ) ;
#25201=ORIENTED_EDGE ( 'NONE', *, *, #172906, .F. ) ;
#25207=ADVANCED_FACE ( 'NONE', ( #202371 ), #153661, .F. ) ;
#25220=EDGE_CURVE ( 'NONE', #83638, #192862, #176369, .T. ) ;
#25228=PRESENTATION_STYLE_ASSIGNMENT (( #158444 ) ) ;
#25234=DIRECTION ( 'NONE',  ( 0.000000000000000000, -1.000000000000000000, 0.000000000000000000 ) ) ;
#25256=ADVANCED_FACE ( 'NONE', ( #91885 ), #81516, .T. ) ;
#25265=CARTESIAN_POINT ( 'NONE',  ( 7.629869294364564958, -5.350481869465718354, 7.876942567271134621 ) ) ;
#25290=CARTESIAN_POINT ( 'NONE',  ( 0.4373347461412347426, -7.712532583864853741, -10.97876033714413069 ) ) ;
#25316=ORIENTED_EDGE ( 'NONE', *, *, #53487, .T. ) ;
#25332=DIRECTION ( 'NONE',  ( 0.000000000000000000, 0.000000000000000000, -1.000000000000000000 ) ) ;
#25384=CARTESIAN_POINT ( 'NONE',  ( 0.000000000000000000, -9.331509131462439655, 0.000000000000000000 ) ) ;
#25435=( NAMED_UNIT ( * ) PLANE_ANGLE_UNIT ( ) SI_UNIT ( $, .RADIAN. ) );
#25457=AXIS2_PLACEMENT_3D ( 'NONE', #154990, #55353, #138751 ) ;
#25464=CARTESIAN_POINT ( 'NONE',  ( 0.000000000000000000, 1.000000000000000888, 0.000000000000000000 ) ) ;
#25491=CARTESIAN_POINT ( 'NONE',  ( -0.1007326007324986367, -10.00000000000001243, -10.99953876047305812 ) ) ;
#25533=CARTESIAN_POINT ( 'NONE',  ( 0.4382560683119193223, -5.166862915010159263, 10.99126615174921007 ) ) ;
#25568=ORIENTED_EDGE ( 'NONE', *, *, #137968, .T. ) ;
#25581=DIRECTION ( 'NONE',  ( -0.000000000000000000, -1.000000000000000000, -0.000000000000000000 ) ) ;
#25592=CARTESIAN_POINT ( 'NONE',  ( 9.499766273075879397, -10.00000000000009592, -0.06663900456897582647 ) ) ;
#25614=ORIENTED_EDGE ( 'NONE', *, *, #85807, .T. ) ;
#25631=CARTESIAN_POINT ( 'NONE',  ( -6.661184041422474778, -7.645986912801312485, 6.773376349081643433 ) ) ;
#25677=CARTESIAN_POINT ( 'NONE',  ( 7.362820735712755749, -5.796536394784340018, 7.362820735709910025 ) ) ;
#25693=EDGE_LOOP ( 'NONE', ( #208329, #166933, #49311, #196295 ) ) ;
#25711=CARTESIAN_POINT ( 'NONE',  ( -2.173285075505815599E-15, -8.011313137147263674, 11.00000000000000178 ) ) ;
#25730=ORIENTED_EDGE ( 'NONE', *, *, #25801, .F. ) ;
#25734=CARTESIAN_POINT ( 'NONE',  ( 10.91812205866965613, -9.932868363016993385, -0.1856806763506236857 ) ) ;
#25789=( BOUNDED_SURFACE ( )  B_SPLINE_SURFACE ( 3, 2, ( 
 ( #188804, #90252, #32701 ),
 ( #15366, #176827, #79323 ),
 ( #48970, #195213, #13252 ),
 ( #114037, #46849, #115087 ) ),
 .UNSPECIFIED., .F., .F., .F. ) 
 B_SPLINE_SURFACE_WITH_KNOTS ( ( 4, 4 ),
 ( 3, 3 ),
 ( 0.01090518310586315390, 0.01337341879808987347 ),
 ( 0.000000000000000000, 1.000000000000000000 ),
 .UNSPECIFIED. ) 
 GEOMETRIC_REPRESENTATION_ITEM ( )  RATIONAL_B_SPLINE_SURFACE ( (
 ( 1.000000000000000000, 0.6967468848055786701, 1.000000000000000000),
 ( 1.000000000000000000, 0.6961913616436842256, 1.000000000000000000),
 ( 1.000000000000000000, 0.6955505937921928616, 1.000000000000000000),
 ( 1.000000000000000000, 0.6947640035364115452, 1.000000000000000000) ) ) 
 REPRESENTATION_ITEM ( '' )  SURFACE ( )  );
#25801=EDGE_CURVE ( 'NONE', #201551, #8301, #179514, .T. ) ;
#25827=ORIENTED_EDGE ( 'NONE', *, *, #115899, .T. ) ;
#25863=CARTESIAN_POINT ( 'NONE',  ( -6.844216539294140311, -8.074889850123483370, 6.588752024304639576 ) ) ;
#25878=ORIENTED_EDGE ( 'NONE', *, *, #201882, .F. ) ;
#25901=AXIS2_PLACEMENT_3D ( 'NONE', #3190, #186225, #5313 ) ;
#25912=CARTESIAN_POINT ( 'NONE',  ( -10.97058181929407716, -5.254568858751056837, 0.2903707658989288509 ) ) ;
#25913=CARTESIAN_POINT ( 'NONE',  ( -10.68054077891638265, -8.644755361503008828, 0.1864295327644238942 ) ) ;
#25927=UNCERTAINTY_MEASURE_WITH_UNIT (LENGTH_MEASURE( 1.000000000000000082E-05 ), #94783, 'distance_accuracy_value', 'NONE');
#25957=CARTESIAN_POINT ( 'NONE',  ( -0.4373225248172954438, -5.223431457505083308, -10.96785329849813273 ) ) ;
#25978=DIRECTION ( 'NONE',  ( 1.000000000000000000, 0.000000000000000000, 0.000000000000000000 ) ) ;
#25987=ORIENTED_EDGE ( 'NONE', *, *, #81885, .T. ) ;
#26006=CARTESIAN_POINT ( 'NONE',  ( -8.996750068618080576, 1.000000000000000888, -7.838941051145383199 ) ) ;
#26009=VERTEX_POINT ( 'NONE', #66771 ) ;
#26047=CARTESIAN_POINT ( 'NONE',  ( -5.204170427930421283E-15, 3.447199233515649386, -11.99999999999998224 ) ) ;
#26062=CARTESIAN_POINT ( 'NONE',  ( 0.4294425147611385940, -9.006862915010128035, -9.490288674561771387 ) ) ;
#26064=CARTESIAN_POINT ( 'NONE',  ( 6.905598574191389005, -7.287292132484016527, 6.905598574191363248 ) ) ;
#26073=CARTESIAN_POINT ( 'NONE',  ( -9.495347311156809411, -6.857257212219918685, 3.422217897015904270E-15 ) ) ;
#26088=B_SPLINE_CURVE_WITH_KNOTS ( 'NONE', 3,
 ( #200970, #198845, #629, #101364, #164246, #1708 ),
 .UNSPECIFIED., .F., .F.,
 ( 4, 2, 4 ),
 ( 0.0004037790303856098246, 0.0007126936173801977749, 0.001021608204374785563 ),
 .UNSPECIFIED. ) ;
#26109=FACE_OUTER_BOUND ( 'NONE', #128209, .T. ) ;
#26119=DIRECTION ( 'NONE',  ( 0.000000000000000000, 1.000000000000000000, 0.000000000000000000 ) ) ;
#26151=DIRECTION ( 'NONE',  ( 0.000000000000000000, 1.000000000000000000, 0.000000000000000000 ) ) ;
#26154=CARTESIAN_POINT ( 'NONE',  ( -9.499668754385632852, -7.473374494045003757, -0.07933194154487524519 ) ) ;
#26170=DIRECTION ( 'NONE',  ( 0.000000000000000000, 0.000000000000000000, -1.000000000000000000 ) ) ;
#26246=ORIENTED_EDGE ( 'NONE', *, *, #130785, .F. ) ;
#26247=ORIENTED_EDGE ( 'NONE', *, *, #99329, .F. ) ;
#26250=AXIS2_PLACEMENT_3D ( 'NONE', #94587, #175828, #160629 ) ;
#26267=ORIENTED_EDGE ( 'NONE', *, *, #7685, .F. ) ;
#26297=( NAMED_UNIT ( * ) SI_UNIT ( $, .STERADIAN. ) SOLID_ANGLE_UNIT ( ) );
#26327=CARTESIAN_POINT ( 'NONE',  ( 7.710915694720367419, -5.615420858948574789, 7.765925996254662067 ) ) ;
#26348=CARTESIAN_POINT ( 'NONE',  ( 10.91877484692250277, -9.999999999999973355, -0.1449562030364739129 ) ) ;
#26377=EDGE_CURVE ( 'NONE', #74902, #7171, #67089, .T. ) ;
#26384=ORIENTED_EDGE ( 'NONE', *, *, #184656, .F. ) ;
#26411=FACE_OUTER_BOUND ( 'NONE', #37940, .T. ) ;
#26427=CIRCLE ( 'NONE', #43782, 10.99999999999999112 ) ;
#26468=CARTESIAN_POINT ( 'NONE',  ( -10.85699613886989390, -6.836286050428373784, 0.3891817118475745518 ) ) ;
#26505=( NAMED_UNIT ( * ) SI_UNIT ( $, .STERADIAN. ) SOLID_ANGLE_UNIT ( ) );
#26520=CIRCLE ( 'NONE', #147606, 0.2000000000000005107 ) ;
#26585=ADVANCED_FACE ( 'NONE', ( #135345 ), #111958, .T. ) ;
#26608=DIRECTION ( 'NONE',  ( 0.7071067811865489050, 0.000000000000000000, 0.7071067811865462405 ) ) ;
#26628=CARTESIAN_POINT ( 'NONE',  ( 6.773846765317306229, 0.000000000000000000, -6.773846765317331986 ) ) ;
#26659=CARTESIAN_POINT ( 'NONE',  ( 9.602438852202270780, -9.449361760816692879, -0.1964824153909916216 ) ) ;
#26717=CARTESIAN_POINT ( 'NONE',  ( 0.000000000000000000, -5.166862915010159263, 0.000000000000000000 ) ) ;
#26786=CARTESIAN_POINT ( 'NONE',  ( 0.07999999999998980149, -5.907420853759267843, -10.91970695577493800 ) ) ;
#26800=ORIENTED_EDGE ( 'NONE', *, *, #166752, .T. ) ;
#26805=SURFACE_STYLE_FILL_AREA ( #121202 ) ;
#26823=EDGE_CURVE ( 'NONE', #111346, #120494, #125409, .T. ) ;
#26824=FACE_OUTER_BOUND ( 'NONE', #2870, .T. ) ;
#26840=CARTESIAN_POINT ( 'NONE',  ( 11.18654035131437219, 1.000000000000000888, -4.041720556560823852 ) ) ;
#26878=DIRECTION ( 'NONE',  ( 0.000000000000000000, -1.000000000000000000, 0.000000000000000000 ) ) ;
#26909=CARTESIAN_POINT ( 'NONE',  ( 0.03130284803985262237, -9.439835433791190056, -9.605218923937751896 ) ) ;
#26928=CARTESIAN_POINT ( 'NONE',  ( -6.880414557363809358, -8.057948861126629225, 6.598949805828049797 ) ) ;
#26937=CARTESIAN_POINT ( 'NONE',  ( -9.261794192842831563, -6.948429295162966035, 5.421010862427522170E-16 ) ) ;
#26938=CARTESIAN_POINT ( 'NONE',  ( 10.15369940311294350, 1.000000000000000888, 6.195664267729887875 ) ) ;
#26961=CARTESIAN_POINT ( 'NONE',  ( 0.4360851681528739587, -8.730413173480727096, -9.960047168614391211 ) ) ;
#26963=AXIS2_PLACEMENT_3D ( 'NONE', #185194, #118150, #122447 ) ;
#27019=CARTESIAN_POINT ( 'NONE',  ( -9.093502852636577316, 1.000000000000000888, -7.666967846417613863 ) ) ;
#27020=ORIENTED_EDGE ( 'NONE', *, *, #114510, .T. ) ;
#27032=( LENGTH_UNIT ( ) NAMED_UNIT ( * ) SI_UNIT ( .MILLI., .METRE. ) );
#27046=CARTESIAN_POINT ( 'NONE',  ( 0.4644097342742973811, -8.233137084989863297, 9.488641820551102057 ) ) ;
#27051=ORIENTED_EDGE ( 'NONE', *, *, #137968, .F. ) ;
#27069=ADVANCED_FACE ( 'NONE', ( #41042 ), #57276, .T. ) ;
#27075=ORIENTED_EDGE ( 'NONE', *, *, #202413, .F. ) ;
#27109=CARTESIAN_POINT ( 'NONE',  ( -7.550983558724452926, -6.148216694138056937, -7.550983558724408518 ) ) ;
#27130=DIRECTION ( 'NONE',  ( 0.000000000000000000, 0.000000000000000000, 1.000000000000000000 ) ) ;
#27132=CARTESIAN_POINT ( 'NONE',  ( -10.35465518852992517, -5.836144560139977955, 0.4365953560983814041 ) ) ;
#27140=EDGE_CURVE ( 'NONE', #6643, #156, #156415, .T. ) ;
#27166=CARTESIAN_POINT ( 'NONE',  ( 7.037870247915954280, -8.233137084989836652, -6.381095703207985359 ) ) ;
#27208=CARTESIAN_POINT ( 'NONE',  ( -7.583016927391839523, -5.196967604326691692, -7.968844136639799736 ) ) ;
#27214=CARTESIAN_POINT ( 'NONE',  ( 9.617648866954018771, -9.063431457505044975, -0.6035590660249217088 ) ) ;
#27231=ORIENTED_EDGE ( 'NONE', *, *, #127420, .F. ) ;
#27242=ADVANCED_FACE ( 'NONE', ( #11703 ), #190453, .F. ) ;
#27256=CARTESIAN_POINT ( 'NONE',  ( 6.773376349083131132, -7.215597533173308875, 6.661184041420955992 ) ) ;
#27315=COLOUR_RGB ( '', 0.40784314, 0.44705882, 0.49803922) ;
#27385=COLOUR_RGB ( '', 0.31764706, 0.68627451, 0.89019608) ;
#27433=ORIENTED_EDGE ( 'NONE', *, *, #30312, .F. ) ;
#27463=DIRECTION ( 'NONE',  ( -0.000000000000000000, -1.000000000000000000, -0.000000000000000000 ) ) ;
#27466=CARTESIAN_POINT ( 'NONE',  ( 7.462104991928524278, -5.166862915010159263, 8.081892667527540652 ) ) ;
#27531=AXIS2_PLACEMENT_3D ( 'NONE', #64759, #112514, #33325 ) ;
#27621=COLOUR_RGB ( '', 0.72549020, 0.75294118, 0.79215686) ;
#27667=CARTESIAN_POINT ( 'NONE',  ( 10.00050683067318502, 3.975933801733730011, -5.773795310722014129 ) ) ;
#27683=ORIENTED_EDGE ( 'NONE', *, *, #113758, .F. ) ;
#27693=CARTESIAN_POINT ( 'NONE',  ( -10.79920600060118119, -6.027819618361849763, 1.138412281109779656E-15 ) ) ;
#27702=DIRECTION ( 'NONE',  ( -0.000000000000000000, -1.000000000000000000, -0.000000000000000000 ) ) ;
#27727=CARTESIAN_POINT ( 'NONE',  ( -0.1480828224388838488, -6.655928102867010310, -10.87712779691733722 ) ) ;
#27791=FACE_OUTER_BOUND ( 'NONE', #209897, .T. ) ;
#27811=EDGE_CURVE ( 'NONE', #34393, #193316, #58954, .T. ) ;
#27859=CARTESIAN_POINT ( 'NONE',  ( 8.081892667527538876, -5.166862915010159263, -7.462104991928523390 ) ) ;
#27860=ORIENTED_EDGE ( 'NONE', *, *, #156157, .T. ) ;
#27864=VERTEX_POINT ( 'NONE', #195557 ) ;
#27892=CARTESIAN_POINT ( 'NONE',  ( -10.67552548858665418, -7.034525073436785902, -2.052149754785371264E-12 ) ) ;
#27916=CARTESIAN_POINT ( 'NONE',  ( 11.21996551234715866, 1.000000000000000888, -3.949207502427110938 ) ) ;
#27919=CARTESIAN_POINT ( 'NONE',  ( -9.578206935421272661, -9.746166700192988586, 0.1671882239536542636 ) ) ;
#28020=B_SPLINE_CURVE_WITH_KNOTS ( 'NONE', 3,
 ( #33760, #98780, #99837, #135544, #50018, #20690, #1236 ),
 .UNSPECIFIED., .F., .F.,
 ( 4, 3, 4 ),
 ( 3.314949680322580664E-05, 0.0009000000012044581665, 0.001958074173707496923 ),
 .UNSPECIFIED. ) ;
#28024=VERTEX_POINT ( 'NONE', #197664 ) ;
#28026=CARTESIAN_POINT ( 'NONE',  ( 0.03146710860973583185, -8.100320323339554207, -10.94525894661336629 ) ) ;
#28060=CARTESIAN_POINT ( 'NONE',  ( 4.593150236022219428E-15, -8.011313137147251240, -11.00000000000000178 ) ) ;
#28073=UNCERTAINTY_MEASURE_WITH_UNIT (LENGTH_MEASURE( 1.000000000000000082E-05 ), #48390, 'distance_accuracy_value', 'NONE');
#28084=ORIENTED_EDGE ( 'NONE', *, *, #125699, .F. ) ;
#28100=CARTESIAN_POINT ( 'NONE',  ( 0.08058606168048106089, -5.741816521215585389, -10.99970480906930526 ) ) ;
#28114=SURFACE_STYLE_USAGE ( .BOTH. , #44380 ) ;
#28136=CIRCLE ( 'NONE', #128569, 9.499999999999991118 ) ;
#28183=ORIENTED_EDGE ( 'NONE', *, *, #54696, .T. ) ;
#28187=CARTESIAN_POINT ( 'NONE',  ( -0.008366613517340566394, 2.629643693813620953, 12.00001160347414775 ) ) ;
#28191=B_SPLINE_CURVE_WITH_KNOTS ( 'NONE', 3,
 ( #155350, #154289, #21047, #55712 ),
 .UNSPECIFIED., .F., .F.,
 ( 4, 4 ),
 ( 0.000000000000000000, 0.0004044236633722958431 ),
 .UNSPECIFIED. ) ;
#28241=CARTESIAN_POINT ( 'NONE',  ( 7.626802973668208807, -6.615717645446816064, 7.927630635717502372 ) ) ;
#28255=PRESENTATION_STYLE_ASSIGNMENT (( #190735 ) ) ;
#28260=CARTESIAN_POINT ( 'NONE',  ( -10.38819714233664193, 3.487142912321087973, 5.997628416523025585 ) ) ;
#28314=CARTESIAN_POINT ( 'NONE',  ( -7.834948807406196813, -5.743759731405707392, -7.720982915751337217 ) ) ;
#28315=DIRECTION ( 'NONE',  ( 0.000000000000000000, 1.000000000000000000, 0.000000000000000000 ) ) ;
#28318=ADVANCED_FACE ( 'NONE', ( #99123 ), #46748, .T. ) ;
#28360=ORIENTED_EDGE ( 'NONE', *, *, #40097, .F. ) ;
#28374=DIRECTION ( 'NONE',  ( 0.000000000000000000, 1.000000000000000000, 0.000000000000000000 ) ) ;
#28411=ORIENTED_EDGE ( 'NONE', *, *, #34950, .F. ) ;
#28440=LINE ( 'NONE', #97728, #192970 ) ;
#28467=DIRECTION ( 'NONE',  ( 0.000000000000000000, 1.000000000000000000, 0.000000000000000000 ) ) ;
#28477=CARTESIAN_POINT ( 'NONE',  ( 10.53927507717371803, 2.018041202054265071, 6.084853302869627889 ) ) ;
#28500=ORIENTED_EDGE ( 'NONE', *, *, #38304, .F. ) ;
#28520=B_SPLINE_CURVE_WITH_KNOTS ( 'NONE', 3,
 ( #173146, #86540, #54046, #120183 ),
 .UNSPECIFIED., .F., .F.,
 ( 4, 4 ),
 ( 0.000000000000000000, 6.033646489354577163E-05 ),
 .UNSPECIFIED. ) ;
#28532=ORIENTED_EDGE ( 'NONE', *, *, #73745, .T. ) ;
#28556=CYLINDRICAL_SURFACE ( 'NONE', #116874, 0.08000000000000020983 ) ;
#28574=CARTESIAN_POINT ( 'NONE',  ( 0.000000000000000000, 1.000000000000000888, 0.000000000000000000 ) ) ;
#28595=DIRECTION ( 'NONE',  ( 0.000000000000000000, 0.000000000000000000, 1.000000000000000000 ) ) ;
#28605=ORIENTED_EDGE ( 'NONE', *, *, #184032, .F. ) ;
#28627=EDGE_CURVE ( 'NONE', #96195, #89267, #156404, .T. ) ;
#28692=ORIENTED_EDGE ( 'NONE', *, *, #72060, .T. ) ;
#28730=VECTOR ( 'NONE', #194395, 1000.000000000000000 ) ;
#28782=DIRECTION ( 'NONE',  ( 0.000000000000000000, 1.000000000000000000, 0.000000000000000000 ) ) ;
#28788=CARTESIAN_POINT ( 'NONE',  ( -2.075332711124689311, 1.720726420432414860, 11.62496126974821919 ) ) ;
#28806=CIRCLE ( 'NONE', #180938, 0.07999999999999940492 ) ;
#28807=CARTESIAN_POINT ( 'NONE',  ( 0.3107038660269477726, -6.804704122739857475, 10.86205067566995552 ) ) ;
#28829=EDGE_CURVE ( 'NONE', #184758, #167216, #141483, .T. ) ;
#28868=B_SPLINE_CURVE_WITH_KNOTS ( 'NONE', 3,
 ( #63901, #31416, #196051, #131103, #179797, #81219, #115907, #113794 ),
 .UNSPECIFIED., .F., .F.,
 ( 4, 2, 2, 4 ),
 ( 0.000000000000000000, 0.0004365159022973243174, 0.0006547738534459874790, 0.0008730318045946505864 ),
 .UNSPECIFIED. ) ;
#28875=DIRECTION ( 'NONE',  ( -0.0006885664517736270196, 0.9962285034897218061, 0.08676574618402708994 ) ) ;
#28884=EDGE_CURVE ( 'NONE', #113279, #68165, #67128, .T. ) ;
#28933=LINE ( 'NONE', #80880, #39327 ) ;
#28934=ORIENTED_EDGE ( 'NONE', *, *, #201067, .F. ) ;
#28956=CARTESIAN_POINT ( 'NONE',  ( -9.926723642588102692, -7.126685749119995528, 0.000000000000000000 ) ) ;
#28971=CARTESIAN_POINT ( 'NONE',  ( 0.4655551865852050608, -8.176568542494919711, 9.512045263456268884 ) ) ;
#29045=ORIENTED_EDGE ( 'NONE', *, *, #12956, .T. ) ;
#29075=SURFACE_SIDE_STYLE ('',( #156955 ) ) ;
#29109=DIRECTION ( 'NONE',  ( -0.06263215618080143765, 4.385051216238358438E-12, -0.9980366791917739677 ) ) ;
#29125=EDGE_CURVE ( 'NONE', #44666, #172003, #180178, .T. ) ;
#29173=VERTEX_POINT ( 'NONE', #121320 ) ;
#29184=CARTESIAN_POINT ( 'NONE',  ( -0.3773006915670014116, -8.233136995002810821, -9.492905263954437345 ) ) ;
#29187=CARTESIAN_POINT ( 'NONE',  ( -0.3870774458628380987, 0.9691415390508737460, 11.89165654491649349 ) ) ;
#29192=CARTESIAN_POINT ( 'NONE',  ( -10.18461545817740088, 3.956598013261175772, 5.433575010662861082 ) ) ;
#29197=CARTESIAN_POINT ( 'NONE',  ( 0.000000000000000000, -9.900000000000005684, 0.000000000000000000 ) ) ;
#29224=ORIENTED_EDGE ( 'NONE', *, *, #125699, .T. ) ;
#29228=MECHANICAL_DESIGN_GEOMETRIC_PRESENTATION_REPRESENTATION('',(#87974),#63689);
#29257=ORIENTED_EDGE ( 'NONE', *, *, #205822, .F. ) ;
#29280=CARTESIAN_POINT ( 'NONE',  ( -1.387778780781445676E-14, -5.907420853759282053, -10.91970695577495398 ) ) ;
#29290=ORIENTED_EDGE ( 'NONE', *, *, #186606, .F. ) ;
#29311=CARTESIAN_POINT ( 'NONE',  ( 7.586197045692582464, -6.654700410849454961, 7.966449380362582211 ) ) ;
#29312=CARTESIAN_POINT ( 'NONE',  ( -6.855650617048461903, -7.357813805523316653, -6.855650617048431705 ) ) ;
#29325=CARTESIAN_POINT ( 'NONE',  ( -10.98677171181893186, -7.666863022246093173, 0.5458515184425656308 ) ) ;
#29335=PRESENTATION_STYLE_ASSIGNMENT (( #49837 ) ) ;
#29337=MECHANICAL_DESIGN_GEOMETRIC_PRESENTATION_REPRESENTATION('',(#198903),#192107);
#29354=ORIENTED_EDGE ( 'NONE', *, *, #19442, .T. ) ;
#29372=AXIS2_PLACEMENT_3D ( 'NONE', #91664, #40768, #58061 ) ;
#29385=EDGE_LOOP ( 'NONE', ( #1258, #38347, #171331, #6860 ) ) ;
#29409=EDGE_CURVE ( 'NONE', #179385, #194999, #169810, .T. ) ;
#29425=CARTESIAN_POINT ( 'NONE',  ( -9.579089671862764277, -9.990657512341117652, 0.1108584966531582228 ) ) ;
#29437=EDGE_CURVE ( 'NONE', #169582, #206352, #208541, .T. ) ;
#29450=DIRECTION ( 'NONE',  ( 0.000000000000000000, 1.000000000000000000, 0.000000000000000000 ) ) ;
#29480=CARTESIAN_POINT ( 'NONE',  ( -10.99970480893081870, -5.907420853759282053, -0.08058608058607828750 ) ) ;
#29489=AXIS2_PLACEMENT_3D ( 'NONE', #167630, #169760, #101562 ) ;
#29514=CARTESIAN_POINT ( 'NONE',  ( 11.20845505065560666, 1.972237431423869314, -3.641847810296739762 ) ) ;
#29554=VERTEX_POINT ( 'NONE', #70324 ) ;
#29576=ORIENTED_EDGE ( 'NONE', *, *, #65507, .F. ) ;
#29585=VERTEX_POINT ( 'NONE', #201394 ) ;
#29595=ORIENTED_EDGE ( 'NONE', *, *, #127031, .T. ) ;
#29608=B_SPLINE_CURVE_WITH_KNOTS ( 'NONE', 3,
 ( #19639, #53217, #1239, #86783, #186402, #51089, #165905, #83576, #117213, #70499 ),
 .UNSPECIFIED., .F., .F.,
 ( 4, 2, 2, 2, 4 ),
 ( 0.000000000000000000, 0.0002021113321160284890, 0.0004042226642320569780, 0.0006063339963480854399, 0.0008084453284641139560 ),
 .UNSPECIFIED. ) ;
#29621=CARTESIAN_POINT ( 'NONE',  ( 0.09481041353608110622, -9.919511983836045488, 9.499526882191826616 ) ) ;
#29641=STYLED_ITEM ( 'NONE', ( #357 ), #192497 ) ;
#29677=ORIENTED_EDGE ( 'NONE', *, *, #190890, .F. ) ;
#29686=B_SPLINE_CURVE_WITH_KNOTS ( 'NONE', 3,
 ( #71579, #185339, #18574, #169098, #20696, #4434, #136619, #202645, #54294, #21750 ),
 .UNSPECIFIED., .F., .F.,
 ( 4, 2, 2, 2, 4 ),
 ( 0.000000000000000000, 0.0002299353307164169933, 0.0004598706614328339866, 0.0006898059921492511425, 0.0009197413228656684068 ),
 .UNSPECIFIED. ) ;
#29702=CARTESIAN_POINT ( 'NONE',  ( 6.773376349083131132, -7.246166700180801001, 6.661184041420955992 ) ) ;
#29770=SURFACE_STYLE_FILL_AREA ( #15617 ) ;
#29818=DIRECTION ( 'NONE',  ( 0.000000000000000000, 1.000000000000000000, 0.000000000000000000 ) ) ;
#29860=VERTEX_POINT ( 'NONE', #32266 ) ;
#29861=CARTESIAN_POINT ( 'NONE',  ( -2.033424464989782354, 3.426985321572576737, 11.42673966862524537 ) ) ;
#29865=CARTESIAN_POINT ( 'NONE',  ( -0.08000000000000714873, -9.999999999999994671, 10.91970695577494865 ) ) ;
#29913=( LENGTH_UNIT ( ) NAMED_UNIT ( * ) SI_UNIT ( .MILLI., .METRE. ) );
#29917=CARTESIAN_POINT ( 'NONE',  ( -8.024744567526244765, -5.166862915010145052, 7.523999700038795702 ) ) ;
#29966=CARTESIAN_POINT ( 'NONE',  ( -7.100579091573050228, -6.583980363594990948, 6.484567079770452658 ) ) ;
#30020=CARTESIAN_POINT ( 'NONE',  ( 8.002408263930250953, -6.836568542494980250, -7.346809171966436125 ) ) ;
#30024=ADVANCED_FACE ( 'NONE', ( #213124 ), #8122, .T. ) ;
#30029=CYLINDRICAL_SURFACE ( 'NONE', #172710, 10.99999999999999112 ) ;
#30087=ADVANCED_FACE ( 'NONE', ( #36518 ), #197973, .T. ) ;
#30120=AXIS2_PLACEMENT_3D ( 'NONE', #112645, #25978, #74746 ) ;
#30121=SURFACE_STYLE_FILL_AREA ( #46381 ) ;
#30125=CARTESIAN_POINT ( 'NONE',  ( -6.773846765317339980, -7.552951973956472997, -6.773846765317302676 ) ) ;
#30164=CARTESIAN_POINT ( 'NONE',  ( -10.38614328979765489, 3.507114751586604129, -5.996442624206661520 ) ) ;
#30172=CARTESIAN_POINT ( 'NONE',  ( 9.920930332858631573, -7.768188185258914302, -0.4648879685169824416 ) ) ;
#30210=UNCERTAINTY_MEASURE_WITH_UNIT (LENGTH_MEASURE( 1.000000000000000082E-05 ), #27032, 'distance_accuracy_value', 'NONE');
#30242=CARTESIAN_POINT ( 'NONE',  ( -0.2726351642629555871, -5.197079954928571333, -10.99683038201373719 ) ) ;
#30269=CARTESIAN_POINT ( 'NONE',  ( 0.1796516426514959408, -8.073984524010706210, 9.498564853506346495 ) ) ;
#30282=CIRCLE ( 'NONE', #161868, 0.07999999999999907185 ) ;
#30312=EDGE_CURVE ( 'NONE', #172003, #121557, #94429, .T. ) ;
#30332=CARTESIAN_POINT ( 'NONE',  ( -7.235142258280603755, -6.594478602024295810, -7.235142258280561123 ) ) ;
#30351=CARTESIAN_POINT ( 'NONE',  ( -8.832353407160665526, 3.956598013261175772, -7.432338980325321920 ) ) ;
#30432=CARTESIAN_POINT ( 'NONE',  ( 9.579665964935223599, -7.246166700194470067, 5.204170427930421283E-15 ) ) ;
#30437=ORIENTED_EDGE ( 'NONE', *, *, #63361, .F. ) ;
#30438=CARTESIAN_POINT ( 'NONE',  ( 10.87712779691733544, -6.655928102867018303, -0.1480828224388737735 ) ) ;
#30442=VECTOR ( 'NONE', #203391, 1000.000000000000000 ) ;
#30461=CARTESIAN_POINT ( 'NONE',  ( -7.717216217110848042, -5.600320323339640360, -7.761717428875279268 ) ) ;
#30467=CARTESIAN_POINT ( 'NONE',  ( 0.000000000000000000, -9.900000000000005684, 0.000000000000000000 ) ) ;
#30493=CARTESIAN_POINT ( 'NONE',  ( 6.598949805828054238, -8.057948861126666529, 6.880414557363697448 ) ) ;
#30530=CARTESIAN_POINT ( 'NONE',  ( 6.784185045882113130, -8.038658175288276198, -6.650326532587137685 ) ) ;
#30586=DIRECTION ( 'NONE',  ( 0.000000000000000000, 0.000000000000000000, 1.000000000000000000 ) ) ;
#30588=CARTESIAN_POINT ( 'NONE',  ( 11.19002393767583747, 0.9691415390508388850, -4.042856490848130591 ) ) ;
#30663=DIRECTION ( 'NONE',  ( 0.000000000000000000, 1.000000000000000000, 0.000000000000000000 ) ) ;
#30679=ORIENTED_EDGE ( 'NONE', *, *, #210461, .T. ) ;
#30718=DIRECTION ( 'NONE',  ( 0.000000000000000000, 1.000000000000000000, 0.000000000000000000 ) ) ;
#30733=CARTESIAN_POINT ( 'NONE',  ( 0.000000000000000000, -6.893137084989842123, 0.000000000000000000 ) ) ;
#30788=ORIENTED_EDGE ( 'NONE', *, *, #2169, .F. ) ;
#30846=FILL_AREA_STYLE_COLOUR ( '', #91045 ) ;
#30871=CARTESIAN_POINT ( 'NONE',  ( 10.85277107007934205, 3.956598013261175772, -3.932872935640606915 ) ) ;
#30920=CARTESIAN_POINT ( 'NONE',  ( 0.3870072406890456840, 1.529612873802629780, -11.82510647457160147 ) ) ;
#30921=CARTESIAN_POINT ( 'NONE',  ( 9.597420367780058470, -7.030163990561723253, -0.01387835396682351140 ) ) ;
#30930=CARTESIAN_POINT ( 'NONE',  ( 0.000000000000000000, 7.849261790823902629, 0.000000000000000000 ) ) ;
#30946=ORIENTED_EDGE ( 'NONE', *, *, #43574, .T. ) ;
#30948=COLOUR_RGB ( '', 0.40784314, 0.44705882, 0.49803922) ;
#30953=CARTESIAN_POINT ( 'NONE',  ( 10.99943592164172657, -8.407420853759269619, -0.1113975120798811613 ) ) ;
#30959=AXIS2_PLACEMENT_3D ( 'NONE', #119293, #172259, #89954 ) ;
#30960=CARTESIAN_POINT ( 'NONE',  ( -9.499668754385632852, 7.849261790823902629, -0.07933194154487524519 ) ) ;
#30961=DIRECTION ( 'NONE',  ( 0.000000000000000000, 1.000000000000000000, 0.000000000000000000 ) ) ;
#30987=CARTESIAN_POINT ( 'NONE',  ( -10.53927507717126666, 2.018041202053943994, -6.084853302868306280 ) ) ;
#31005=FACE_OUTER_BOUND ( 'NONE', #18970, .T. ) ;
#31048=CYLINDRICAL_SURFACE ( 'NONE', #82018, 0.08000000000000020983 ) ;
#31074=EDGE_CURVE ( 'NONE', #95548, #90583, #108388, .T. ) ;
#31107=( LENGTH_UNIT ( ) NAMED_UNIT ( * ) SI_UNIT ( .MILLI., .METRE. ) );
#31160=PLANE ( 'NONE',  #46701 ) ;
#31187=VERTEX_POINT ( 'NONE', #187846 ) ;
#31197=VECTOR ( 'NONE', #212434, 1000.000000000000000 ) ;
#31233=EDGE_CURVE ( 'NONE', #162811, #21086, #89566, .T. ) ;
#31239=( NAMED_UNIT ( * ) SI_UNIT ( $, .STERADIAN. ) SOLID_ANGLE_UNIT ( ) );
#31312=VERTEX_POINT ( 'NONE', #131449 ) ;
#31336=CARTESIAN_POINT ( 'NONE',  ( -10.41114276008726058, -8.296408557650112314, 0.1817271728542615705 ) ) ;
#31338=ORIENTED_EDGE ( 'NONE', *, *, #166799, .F. ) ;
#31416=CARTESIAN_POINT ( 'NONE',  ( 6.673079560224744355, -7.008190897455786939, -6.761669295867157814 ) ) ;
#31446=EDGE_CURVE ( 'NONE', #89957, #121080, #87603, .T. ) ;
#31448=CARTESIAN_POINT ( 'NONE',  ( 0.000000000000000000, -9.911192057434348612, 9.579665964948883783 ) ) ;
#31452=VERTEX_POINT ( 'NONE', #113085 ) ;
#31480=CARTESIAN_POINT ( 'NONE',  ( 9.474246188248169886, -6.532648833121171172, -0.3333842132581051887 ) ) ;
#31549=CARTESIAN_POINT ( 'NONE',  ( 0.000000000000000000, 3.799999999999998046, 0.000000000000000000 ) ) ;
#31558=CARTESIAN_POINT ( 'NONE',  ( -9.579592329540000506, -9.999999999999994671, 0.07839159645131747733 ) ) ;
#31561=FACE_OUTER_BOUND ( 'NONE', #74634, .T. ) ;
#31593=DIRECTION ( 'NONE',  ( 0.000000000000000000, 1.000000000000000000, 0.000000000000000000 ) ) ;
#31646=CARTESIAN_POINT ( 'NONE',  ( 10.91339599544321892, -6.211932585243247651, 5.201946966443877167E-15 ) ) ;
#31649=CARTESIAN_POINT ( 'NONE',  ( -0.09999999999989878097, -10.00000000000009592, -10.91954211494242877 ) ) ;
#31652=CARTESIAN_POINT ( 'NONE',  ( 6.609253696060806149, -8.104785249476799791, 6.824425546749157689 ) ) ;
#31663=CARTESIAN_POINT ( 'NONE',  ( 7.806764249273698830, -6.480061791515699277, 7.750016138724927117 ) ) ;
#31759=CARTESIAN_POINT ( 'NONE',  ( 0.09916492693110359746, -9.919999999999998153, 9.499482423651659957 ) ) ;
#31789=EDGE_CURVE ( 'NONE', #125304, #116857, #37081, .T. ) ;
#31820=STYLED_ITEM ( 'NONE', ( #42619 ), #74846 ) ;
#31900=ORIENTED_EDGE ( 'NONE', *, *, #29437, .T. ) ;
#31942=CARTESIAN_POINT ( 'NONE',  ( 0.000000000000000000, 15.50000000000019362, 0.000000000000000000 ) ) ;
#31972=AXIS2_PLACEMENT_3D ( 'NONE', #195993, #132089, #96378 ) ;
#32006=CARTESIAN_POINT ( 'NONE',  ( 0.000000000000000000, -2.079999999999998295, 0.000000000000000000 ) ) ;
#32036=CARTESIAN_POINT ( 'NONE',  ( -10.10493793804576868, 0.9691415390508768546, -6.281047173807432493 ) ) ;
#32072=CARTESIAN_POINT ( 'NONE',  ( -9.586610838029429260, -7.161464053357574855, 0.003376046620574835178 ) ) ;
#32117=CARTESIAN_POINT ( 'NONE',  ( -1.138412281109779656E-15, -9.756397064627572391, 9.569424307476239733 ) ) ;
#32130=ORIENTED_EDGE ( 'NONE', *, *, #133645, .F. ) ;
#32142=CARTESIAN_POINT ( 'NONE',  ( 9.499700864329909678, -7.154544010627095219, 0.07538891330675548397 ) ) ;
#32150=AXIS2_PLACEMENT_3D ( 'NONE', #175874, #27463, #110921 ) ;
#32156=CARTESIAN_POINT ( 'NONE',  ( -11.31269326259043062, 3.603011019375360391, 3.682594235848481556 ) ) ;
#32207=EDGE_CURVE ( 'NONE', #170100, #101997, #163678, .T. ) ;
#32257=COLOUR_RGB ( '', 0.31764706, 0.68627451, 0.89019608) ;
#32266=CARTESIAN_POINT ( 'NONE',  ( -0.07933194154489606187, -9.746166700180788567, -9.499668754385620417 ) ) ;
#32268=CARTESIAN_POINT ( 'NONE',  ( 0.08058608058607655278, -8.407420853759283830, 10.99970480893082225 ) ) ;
#32270=DIRECTION ( 'NONE',  ( -1.561558963378126405E-12, 1.000000000000000000, -1.535693738323023938E-12 ) ) ;
#32271=CARTESIAN_POINT ( 'NONE',  ( 10.33293948230768144, 2.515145635913765165, -5.518992160705104233 ) ) ;
#32293=CARTESIAN_POINT ( 'NONE',  ( -0.04325334852942971930, -8.075271019047999488, -11.00023204605253113 ) ) ;
#32310=CARTESIAN_POINT ( 'NONE',  ( 2.189868734255736360, 1.000000000000000888, -11.69137891449145172 ) ) ;
#32360=DIRECTION ( 'NONE',  ( 0.000000000000000000, 1.000000000000000000, 0.000000000000000000 ) ) ;
#32385=EDGE_CURVE ( 'NONE', #35700, #401, #22380, .T. ) ;
#32395=DIRECTION ( 'NONE',  ( 0.000000000000000000, 0.000000000000000000, -1.000000000000000000 ) ) ;
#32500=CARTESIAN_POINT ( 'NONE',  ( 0.000000000000000000, -6.583980363594976737, 0.000000000000000000 ) ) ;
#32552=CARTESIAN_POINT ( 'NONE',  ( 10.99622371251743225, -6.863149499369291640, -0.2970643657731165121 ) ) ;
#32565=AXIS2_PLACEMENT_3D ( 'NONE', #119250, #185234, #5400 ) ;
#32567=DIRECTION ( 'NONE',  ( 0.000000000000000000, 0.000000000000000000, 1.000000000000000000 ) ) ;
#32569=CARTESIAN_POINT ( 'NONE',  ( -0.03952929641551498896, -5.422159130394869742, -11.00000000000004974 ) ) ;
#32581=CARTESIAN_POINT ( 'NONE',  ( 0.07933191607487939667, -9.582912294610213877, 9.499668754598326714 ) ) ;
#32695=CARTESIAN_POINT ( 'NONE',  ( 10.87798840695972657, -6.646059016331632208, -0.1412570932017882808 ) ) ;
#32701=CARTESIAN_POINT ( 'NONE',  ( -7.728718841570993092, -6.124285368609180047, 7.728718841571021514 ) ) ;
#32705=FILL_AREA_STYLE_COLOUR ( '', #172428 ) ;
#32759=CARTESIAN_POINT ( 'NONE',  ( 0.000000000000000000, 1.000000000000000888, 0.000000000000000000 ) ) ;
#32771=CARTESIAN_POINT ( 'NONE',  ( 7.253312916980309666, -6.796015482748904546, -7.253312916980335423 ) ) ;
#32781=COLOUR_RGB ( '', 0.72549020, 0.75294118, 0.79215686) ;
#32782=B_SPLINE_CURVE_WITH_KNOTS ( 'NONE', 3,
 ( #165785, #182008, #17368, #118160, #69313, #83452, #1118 ),
 .UNSPECIFIED., .F., .F.,
 ( 4, 3, 4 ),
 ( 0.0001126021369358783168, 0.001495765174703651531, 0.002006790696433101342 ),
 .UNSPECIFIED. ) ;
#32900=VERTEX_POINT ( 'NONE', #160574 ) ;
#33000=CARTESIAN_POINT ( 'NONE',  ( -10.99683038201373719, -5.197079954928573109, 0.2726351642629477601 ) ) ;
#33019=ORIENTED_EDGE ( 'NONE', *, *, #185379, .T. ) ;
#33026=TOROIDAL_SURFACE ( 'NONE', #36416, 6.330000000000000959, 0.08000000000000000167 ) ;
#33075=PRODUCT_DEFINITION_CONTEXT ( 'detailed design', #211010, 'design' ) ;
#33087=AXIS2_PLACEMENT_3D ( 'NONE', #170549, #5889, #71962 ) ;
#33092=VERTEX_POINT ( 'NONE', #163791 ) ;
#33097=CARTESIAN_POINT ( 'NONE',  ( -6.773846765307993678, -7.473374494058229622, -6.773846765307958151 ) ) ;
#33100=B_SPLINE_CURVE_WITH_KNOTS ( 'NONE', 3,
 ( #74789, #36942, #5480, #86767, #103023, #107347, #152838 ),
 .UNSPECIFIED., .F., .F.,
 ( 4, 3, 4 ),
 ( 0.0001135037246156260884, 0.0006171834326598004457, 0.002007692286214980693 ),
 .UNSPECIFIED. ) ;
#33112=CARTESIAN_POINT ( 'NONE',  ( 6.662118508819760088, -7.185026885899511662, -6.772457744868767726 ) ) ;
#33121=CARTESIAN_POINT ( 'NONE',  ( -0.3618152180564696563, -5.223163831703879545, -10.97113184882213055 ) ) ;
#33157=DIRECTION ( 'NONE',  ( 0.000000000000000000, 1.000000000000000000, 0.000000000000000000 ) ) ;
#33184=DIRECTION ( 'NONE',  ( 0.000000000000000000, 0.000000000000000000, 1.000000000000000000 ) ) ;
#33195=ADVANCED_FACE ( 'NONE', ( #162728 ), #16836, .T. ) ;
#33245=CARTESIAN_POINT ( 'NONE',  ( -7.845789747616925602, -6.699703214240756211, 7.710100441483631606 ) ) ;
#33257=B_SPLINE_CURVE_WITH_KNOTS ( 'NONE', 3,
 ( #160575, #122317, #88667, #154727, #84382, #136350, #86515, #36686 ),
 .UNSPECIFIED., .F., .F.,
 ( 4, 2, 2, 4 ),
 ( 7.043516722447106004E-16, 0.0002305131806122208513, 0.0004610263612237373507, 0.0009220527224467680184 ),
 .UNSPECIFIED. ) ;
#33268=FILL_AREA_STYLE ('',( #180589 ) ) ;
#33270=CARTESIAN_POINT ( 'NONE',  ( -0.09916492693111574053, -9.919999999999998153, -9.499482423651645746 ) ) ;
#33311=DIRECTION ( 'NONE',  ( 0.000000000000000000, -1.000000000000000000, 0.000000000000000000 ) ) ;
#33325=DIRECTION ( 'NONE',  ( 0.000000000000000000, 0.000000000000000000, -1.000000000000000000 ) ) ;
#33353=( LENGTH_UNIT ( ) NAMED_UNIT ( * ) SI_UNIT ( .MILLI., .METRE. ) );
#33372=ORIENTED_EDGE ( 'NONE', *, *, #130785, .T. ) ;
#33383=CIRCLE ( 'NONE', #154467, 0.08000000000000001554 ) ;
#33388=CARTESIAN_POINT ( 'NONE',  ( 0.4373225248172890045, -5.223431457505089526, 10.96785329849812385 ) ) ;
#33457=UNCERTAINTY_MEASURE_WITH_UNIT (LENGTH_MEASURE( 1.000000000000000082E-05 ), #151033, 'distance_accuracy_value', 'NONE');
#33466=ORIENTED_EDGE ( 'NONE', *, *, #53547, .T. ) ;
#33507=DIRECTION ( 'NONE',  ( 0.000000000000000000, 1.000000000000000000, 0.000000000000000000 ) ) ;
#33514=AXIS2_PLACEMENT_3D ( 'NONE', #139362, #53829, #187014 ) ;
#33531=CARTESIAN_POINT ( 'NONE',  ( -7.346809171966454777, -6.836568542494980250, -8.002408263930250953 ) ) ;
#33554=EDGE_CURVE ( 'NONE', #184431, #18108, #61717, .T. ) ;
#33559=ORIENTED_EDGE ( 'NONE', *, *, #37862, .F. ) ;
#33565=CARTESIAN_POINT ( 'NONE',  ( 8.917737905728804648, 3.038492715500545227, 8.029567276306215362 ) ) ;
#33573=DIRECTION ( 'NONE',  ( 0.000000000000000000, 0.000000000000000000, -1.000000000000000000 ) ) ;
#33574=CARTESIAN_POINT ( 'NONE',  ( 9.499668754385625746, -7.215597533182398493, 0.07933194154557826616 ) ) ;
#33591=DIRECTION ( 'NONE',  ( 0.000000000000000000, 0.000000000000000000, 1.000000000000000000 ) ) ;
#33596=DIRECTION ( 'NONE',  ( 0.000000000000000000, -0.000000000000000000, 1.000000000000000000 ) ) ;
#33597=( BOUNDED_SURFACE ( )  B_SPLINE_SURFACE ( 3, 2, ( 
 ( #76946, #209064, #210137 ),
 ( #26064, #78020, #60701 ),
 ( #92177, #143071, #58579 ),
 ( #175543, #107396, #158227 ) ),
 .UNSPECIFIED., .F., .F., .T. ) 
 B_SPLINE_SURFACE_WITH_KNOTS ( ( 4, 4 ),
 ( 3, 3 ),
 ( 0.01127358803094578865, 0.01374177962974961961 ),
 ( 0.000000000000000000, 1.000000000000000000 ),
 .UNSPECIFIED. ) 
 GEOMETRIC_REPRESENTATION_ITEM ( )  RATIONAL_B_SPLINE_SURFACE ( (
 ( 1.000000000000000000, 0.6947640035331666963, 1.000000000000000000),
 ( 1.000000000000000000, 0.6955505939615598265, 1.000000000000000000),
 ( 1.000000000000000000, 0.6961913616428399010, 1.000000000000000000),
 ( 1.000000000000000000, 0.6967468848049991337, 1.000000000000000000) ) ) 
 REPRESENTATION_ITEM ( '' )  SURFACE ( )  );
#33600=ORIENTED_EDGE ( 'NONE', *, *, #132620, .T. ) ;
#33616=CARTESIAN_POINT ( 'NONE',  ( -2.927345865710862366E-15, -5.221050908132846224, -10.98765602437502764 ) ) ;
#33637=CYLINDRICAL_SURFACE ( 'NONE', #54652, 11.99999999999999112 ) ;
#33655=DIRECTION ( 'NONE',  ( 0.000000000000000000, -1.000000000000000000, 0.000000000000000000 ) ) ;
#33674=EDGE_CURVE ( 'NONE', #76748, #157260, #29686, .T. ) ;
#33676=CARTESIAN_POINT ( 'NONE',  ( -11.37385970535894231, 1.000000000000000888, 3.825613075418397457 ) ) ;
#33760=CARTESIAN_POINT ( 'NONE',  ( 10.96785329849812562, -5.223431457505089526, -0.4373225248172959434 ) ) ;
#33783=CARTESIAN_POINT ( 'NONE',  ( 10.20626665084801843, 3.700502905159948508, 5.921468070729023481 ) ) ;
#33791=STYLED_ITEM ( 'NONE', ( #146031 ), #200496 ) ;
#33828=ORIENTED_EDGE ( 'NONE', *, *, #212430, .T. ) ;
#33857=CARTESIAN_POINT ( 'NONE',  ( 0.005973655272069301574, -7.189371949516782934, 9.500370076773188899 ) ) ;
#33865=CARTESIAN_POINT ( 'NONE',  ( 0.09053139919706915117, -9.918143888366140359, 9.499568811299539561 ) ) ;
#33871=FACE_OUTER_BOUND ( 'NONE', #143798, .T. ) ;
#33910=EDGE_CURVE ( 'NONE', #169582, #16492, #162069, .T. ) ;
#33917=CIRCLE ( 'NONE', #213707, 9.636568542494918788 ) ;
#33933=( GEOMETRIC_REPRESENTATION_CONTEXT ( 3 ) GLOBAL_UNCERTAINTY_ASSIGNED_CONTEXT ( ( #184986 ) ) GLOBAL_UNIT_ASSIGNED_CONTEXT ( ( #182006, #53086, #82385 ) ) REPRESENTATION_CONTEXT ( 'NONE', 'WORKASPACE' ) );
#33934=AXIS2_PLACEMENT_3D ( 'NONE', #124618, #174369, #92055 ) ;
#33969=EDGE_CURVE ( 'NONE', #213712, #139878, #127519, .T. ) ;
#33993=CARTESIAN_POINT ( 'NONE',  ( -6.956180625286119579, -6.372104534813793464, -6.956180625285381502 ) ) ;
#34056=CARTESIAN_POINT ( 'NONE',  ( -10.99948089704804843, -5.389012432655393425, 0.1178541238725522855 ) ) ;
#34073=( BOUNDED_SURFACE ( )  B_SPLINE_SURFACE ( 3, 2, ( 
 ( #177589, #212189, #77941 ),
 ( #147231, #12923, #211125 ),
 ( #11864, #144062, #46528 ),
 ( #96355, #176516, #159192 ),
 ( #110516, #30269, #60622 ),
 ( #64886, #93154, #81146 ),
 ( #131032, #114775, #162410 ),
 ( #63827, #129985, #27046 ) ),
 .UNSPECIFIED., .F., .F., .T. ) 
 B_SPLINE_SURFACE_WITH_KNOTS ( ( 4, 2, 2, 4 ),
 ( 3, 3 ),
 ( 0.000000000000000000, 0.0005123566476021777739, 0.0007685349714032666067, 0.001024713295204355548 ),
 ( 0.000000000000000000, 1.000000000000000000 ),
 .UNSPECIFIED. ) 
 GEOMETRIC_REPRESENTATION_ITEM ( )  RATIONAL_B_SPLINE_SURFACE ( (
 ( 1.000000000000000000, 0.7100530722026825448, 1.000000000000000000),
 ( 1.000000000000000000, 0.7667719522827929346, 1.000000000000000000),
 ( 1.000000000000000000, 0.8160440554222314624, 1.000000000000000000),
 ( 1.000000000000000000, 0.8737249316770007157, 1.000000000000000000),
 ( 1.000000000000000000, 0.8903164784319989034, 1.000000000000000000),
 ( 1.000000000000000000, 0.9150853305241244406, 1.000000000000000000),
 ( 1.000000000000000000, 0.9227739504732713760, 1.000000000000000000),
 ( 1.000000000000000000, 0.9238795325112854062, 1.000000000000000000) ) ) 
 REPRESENTATION_ITEM ( '' )  SURFACE ( )  );
#34118=DIRECTION ( 'NONE',  ( 0.000000000000000000, 0.000000000000000000, 1.000000000000000000 ) ) ;
#34154=CARTESIAN_POINT ( 'NONE',  ( 10.99462479582585317, -5.166863022246526604, -0.3540227772641220683 ) ) ;
#34238=AXIS2_PLACEMENT_3D ( 'NONE', #177445, #176382, #195821 ) ;
#34242=CARTESIAN_POINT ( 'NONE',  ( 0.000000000000000000, -5.166862915010159263, 0.000000000000000000 ) ) ;
#34259=CARTESIAN_POINT ( 'NONE',  ( 9.579665964947855272, -7.246166700193438892, -1.544988095791843818E-15 ) ) ;
#34294=CARTESIAN_POINT ( 'NONE',  ( -10.23541933785880431, 1.000000000000000888, -6.134053304049098543 ) ) ;
#34312=STYLED_ITEM ( 'NONE', ( #25228 ), #44250 ) ;
#34321=VECTOR ( 'NONE', #10711, 1000.000000000000000 ) ;
#34352=ORIENTED_EDGE ( 'NONE', *, *, #102667, .T. ) ;
#34393=VERTEX_POINT ( 'NONE', #170708 ) ;
#34418=DIRECTION ( 'NONE',  ( 0.000000000000000000, 0.000000000000000000, -1.000000000000000000 ) ) ;
#34453=CARTESIAN_POINT ( 'NONE',  ( 7.720982897393566802, -6.134628647623485698, -7.834948825496929281 ) ) ;
#34478=CARTESIAN_POINT ( 'NONE',  ( 0.000000000000000000, -8.233137084989836652, 0.000000000000000000 ) ) ;
#34484=CARTESIAN_POINT ( 'NONE',  ( -9.498884434226665618, -9.954196546781716393, 0.1657939142878951944 ) ) ;
#34536=CARTESIAN_POINT ( 'NONE',  ( -1.138412281109779656E-15, -6.465328379374292389, -10.58872653680446696 ) ) ;
#34593=DIRECTION ( 'NONE',  ( -1.000000000000000000, -0.000000000000000000, -0.000000000000000000 ) ) ;
#34634=CARTESIAN_POINT ( 'NONE',  ( -6.764898216730284908, -7.628386336122852995, 6.764898216727350366 ) ) ;
#34651=CARTESIAN_POINT ( 'NONE',  ( 10.39230484541330313, 3.447199233515649386, 5.999999999999906741 ) ) ;
#34672=CARTESIAN_POINT ( 'NONE',  ( 10.99917004716958857, -6.764708007038256810, -0.1531059978909480312 ) ) ;
#34676=( BOUNDED_SURFACE ( )  B_SPLINE_SURFACE ( 3, 2, ( 
 ( #189866, #64146, #30588 ),
 ( #13251, #29514, #128169 ),
 ( #95607, #177901, #44712 ),
 ( #12178, #15365, #196277 ) ),
 .UNSPECIFIED., .F., .F., .T. ) 
 B_SPLINE_SURFACE_WITH_KNOTS ( ( 4, 4 ),
 ( 3, 3 ),
 ( 0.005241070803109281785, 0.008267458746840847944 ),
 ( 0.000000000000000000, 1.000000000000000000 ),
 .UNSPECIFIED. ) 
 GEOMETRIC_REPRESENTATION_ITEM ( )  RATIONAL_B_SPLINE_SURFACE ( (
 ( 1.000000000000000000, 0.7184380228464080087, 1.000000000000000000),
 ( 1.000000000000000000, 0.7185467277397550312, 1.000000000000000000),
 ( 1.000000000000000000, 0.7186585579881030750, 1.000000000000000000),
 ( 1.000000000000000000, 0.7187737999613691420, 1.000000000000000000) ) ) 
 REPRESENTATION_ITEM ( '' )  SURFACE ( )  );
#34688=DIRECTION ( 'NONE',  ( 0.000000000000000000, 1.000000000000000000, 0.000000000000000000 ) ) ;
#34690=DIRECTION ( 'NONE',  ( 0.000000000000000000, 0.000000000000000000, 1.000000000000000000 ) ) ;
#34760=CARTESIAN_POINT ( 'NONE',  ( 6.689586359223958389, -7.817744194000435520, -6.745922712994591564 ) ) ;
#34765=CARTESIAN_POINT ( 'NONE',  ( -6.777912011469602760, -7.189630408300049069, 6.776323704810609527 ) ) ;
#34775=ORIENTED_EDGE ( 'NONE', *, *, #130557, .F. ) ;
#34790=AXIS2_PLACEMENT_3D ( 'NONE', #207291, #113075, #76228 ) ;
#34827=CARTESIAN_POINT ( 'NONE',  ( 9.579665964948885559, -7.473374494045003757, 0.07999999999999847511 ) ) ;
#34835=ORIENTED_EDGE ( 'NONE', *, *, #137674, .T. ) ;
#34851=CARTESIAN_POINT ( 'NONE',  ( 7.058808231563191704, -6.527411821100059797, -6.446420058208622628 ) ) ;
#34882=DIRECTION ( 'NONE',  ( -0.000000000000000000, -1.000000000000000000, -0.000000000000000000 ) ) ;
#34887=ORIENTED_EDGE ( 'NONE', *, *, #201882, .T. ) ;
#34900=EDGE_CURVE ( 'NONE', #61589, #142909, #162218, .T. ) ;
#34907=VERTEX_POINT ( 'NONE', #92190 ) ;
#34926=CARTESIAN_POINT ( 'NONE',  ( 7.407835137441771245, -5.166862915010159263, 8.023115266309158500 ) ) ;
#34950=EDGE_CURVE ( 'NONE', #82080, #119302, #20408, .T. ) ;
#34961=B_SPLINE_CURVE_WITH_KNOTS ( 'NONE', 3,
 ( #210890, #47364, #14816, #130791, #115590, #178419, #113478 ),
 .UNSPECIFIED., .F., .F.,
 ( 4, 3, 4 ),
 ( 8.673617379884028731E-19, 0.0008000000000005099386, 0.002977368225425562967 ),
 .UNSPECIFIED. ) ;
#34962=DIRECTION ( 'NONE',  ( 0.000000000000000000, 1.000000000000000000, 0.000000000000000000 ) ) ;
#34973=AXIS2_PLACEMENT_3D ( 'NONE', #153626, #72347, #40955 ) ;
#35004=CARTESIAN_POINT ( 'NONE',  ( 0.2834499351972658010, -6.554910260573309166, 9.477100694337659448 ) ) ;
#35095=DIRECTION ( 'NONE',  ( 0.000000000000000000, 0.000000000000000000, -1.000000000000000000 ) ) ;
#35104=VERTEX_POINT ( 'NONE', #94314 ) ;
#35114=CARTESIAN_POINT ( 'NONE',  ( 0.07933194154487524519, -7.473374494045017968, -9.499668754385622194 ) ) ;
#35116=CARTESIAN_POINT ( 'NONE',  ( -7.097136523687877840, -8.233137084989836652, 6.434831245971847302 ) ) ;
#35224=ORIENTED_EDGE ( 'NONE', *, *, #143273, .F. ) ;
#35229=CIRCLE ( 'NONE', #59054, 0.08000000000000040412 ) ;
#35298=EDGE_LOOP ( 'NONE', ( #26267, #204045, #141329, #12018, #181001, #164791 ) ) ;
#35348=CONICAL_SURFACE ( 'NONE', #204797, 8.368490868537556082, 0.7853981633974479459 ) ;
#35372=B_SPLINE_CURVE_WITH_KNOTS ( 'NONE', 3,
 ( #91559, #9212, #7047, #43873, #59026, #192211, #142452, #56896, #109989, #123071, #171706, #40666, #140317, #156545, #22222, #88335 ),
 .UNSPECIFIED., .F., .F.,
 ( 4, 3, 3, 3, 3, 4 ),
 ( 0.000000000000000000, 6.716675436053851645E-06, 1.344324725955300992E-05, 2.018532118335282307E-05, 2.694176617306668026E-05, 3.135538808400729303E-05 ),
 .UNSPECIFIED. ) ;
#35373=LINE ( 'NONE', #51649, #70580 ) ;
#35410=ORIENTED_EDGE ( 'NONE', *, *, #182811, .T. ) ;
#35422=ORIENTED_EDGE ( 'NONE', *, *, #38065, .T. ) ;
#35429=ORIENTED_EDGE ( 'NONE', *, *, #180435, .T. ) ;
#35432=CIRCLE ( 'NONE', #204881, 6.249999999999995559 ) ;
#35436=CARTESIAN_POINT ( 'NONE',  ( 10.99970480893080627, -6.134628647623513231, 0.08058608058608522640 ) ) ;
#35450=ADVANCED_FACE ( 'NONE', ( #8783 ), #206119, .T. ) ;
#35457=( BOUNDED_SURFACE ( )  B_SPLINE_SURFACE ( 3, 2, ( 
 ( #101447, #122059, #69985 ),
 ( #167520, #188023, #54840 ),
 ( #89493, #136097, #37516 ),
 ( #67846, #2852, #199999 ) ),
 .UNSPECIFIED., .F., .F., .T. ) 
 B_SPLINE_SURFACE_WITH_KNOTS ( ( 4, 4 ),
 ( 3, 3 ),
 ( 0.01090155471707268328, 0.01336979040894267431 ),
 ( 0.000000000000000000, 1.000000000000000000 ),
 .UNSPECIFIED. ) 
 GEOMETRIC_REPRESENTATION_ITEM ( )  RATIONAL_B_SPLINE_SURFACE ( (
 ( 1.000000000000000000, 0.6967468848055766717, 1.000000000000000000),
 ( 1.000000000000000000, 0.6961913616436843366, 1.000000000000000000),
 ( 1.000000000000000000, 0.6955505937926286242, 1.000000000000000000),
 ( 1.000000000000000000, 0.6947640035364027744, 1.000000000000000000) ) ) 
 REPRESENTATION_ITEM ( '' )  SURFACE ( )  );
#35476=CARTESIAN_POINT ( 'NONE',  ( -6.745922712994596893, -7.817744194000435520, -6.689586359223953060 ) ) ;
#35490=ORIENTED_EDGE ( 'NONE', *, *, #172906, .T. ) ;
#35515=AXIS2_PLACEMENT_3D ( 'NONE', #47107, #14559, #111083 ) ;
#35516=CARTESIAN_POINT ( 'NONE',  ( 0.1749484593404549426, -5.350147675656140578, 10.96499746917716855 ) ) ;
#35541=EDGE_LOOP ( 'NONE', ( #193946, #196270, #118097, #35422, #115470 ) ) ;
#35550=DIRECTION ( 'NONE',  ( 0.000000000000000000, 1.000000000000000000, 0.000000000000000000 ) ) ;
#35565=SURFACE_STYLE_FILL_AREA ( #150412 ) ;
#35599=EDGE_CURVE ( 'NONE', #94234, #34907, #148623, .T. ) ;
#35615=EDGE_CURVE ( 'NONE', #12329, #167635, #126896, .T. ) ;
#35650=CARTESIAN_POINT ( 'NONE',  ( -6.277139874739040337, -0.02379966007286238305, 0.000000000000000000 ) ) ;
#35651=STYLED_ITEM ( 'NONE', ( #47325 ), #80971 ) ;
#35654=CARTESIAN_POINT ( 'NONE',  ( 1.347111479062088799E-15, -0.9200000000000041478, -11.00000000000000178 ) ) ;
#35678=CARTESIAN_POINT ( 'NONE',  ( -0.09999999999991612820, -10.00000000000009592, -9.579478065114042096 ) ) ;
#35687=CARTESIAN_POINT ( 'NONE',  ( -0.08044988649999126884, -9.906619926850268598, -9.499659352616909302 ) ) ;
#35697=CARTESIAN_POINT ( 'NONE',  ( -7.055228938194283650, -8.176568542494891290, 6.396834479292372144 ) ) ;
#35698=CARTESIAN_POINT ( 'NONE',  ( 9.499668754385636404, -7.246166700194470067, 0.07933194154488391880 ) ) ;
#35700=VERTEX_POINT ( 'NONE', #165700 ) ;
#35716=DIRECTION ( 'NONE',  ( 0.000000000000000000, 1.000000000000000000, 0.000000000000000000 ) ) ;
#35731=EDGE_CURVE ( 'NONE', #29554, #172976, #51500, .T. ) ;
#35737=ORIENTED_EDGE ( 'NONE', *, *, #128001, .T. ) ;
#35738=CARTESIAN_POINT ( 'NONE',  ( 10.14375151705082878, -9.181160345032706616, -0.1770598413457902254 ) ) ;
#35739=DIRECTION ( 'NONE',  ( 0.3090169943749516146, 0.000000000000000000, 0.9510565162951523099 ) ) ;
#35761=EDGE_LOOP ( 'NONE', ( #118774, #64947, #176888, #139517 ) ) ;
#35768=EDGE_LOOP ( 'NONE', ( #120296, #8957, #173232, #190200 ) ) ;
#35786=CARTESIAN_POINT ( 'NONE',  ( 9.499668754385638181, -7.559700871049417792, 0.07933194154488390493 ) ) ;
#35793=ORIENTED_EDGE ( 'NONE', *, *, #196420, .T. ) ;
#35794=FILL_AREA_STYLE ('',( #118186 ) ) ;
#35849=B_SPLINE_CURVE_WITH_KNOTS ( 'NONE', 3,
 ( #39463, #170524, #105559, #22107, #24257, #169461, #204059, #8015 ),
 .UNSPECIFIED., .F., .F.,
 ( 4, 2, 2, 4 ),
 ( 0.000000000000000000, 0.0005156231957999669446, 0.0007734347936999512842, 0.001031246391599935624 ),
 .UNSPECIFIED. ) ;
#35869=( BOUNDED_SURFACE ( )  B_SPLINE_SURFACE ( 3, 2, ( 
 ( #136845, #68606, #54518 ),
 ( #186641, #101118, #83804 ),
 ( #167205, #33993, #18794 ),
 ( #1465, #100067, #67530 ) ),
 .UNSPECIFIED., .F., .F., .T. ) 
 B_SPLINE_SURFACE_WITH_KNOTS ( ( 4, 4 ),
 ( 3, 3 ),
 ( 0.04893088146668654603, 0.05137248493452926251 ),
 ( 0.000000000000000000, 1.000000000000000000 ),
 .UNSPECIFIED. ) 
 GEOMETRIC_REPRESENTATION_ITEM ( )  RATIONAL_B_SPLINE_SURFACE ( (
 ( 1.000000000000000000, 0.7169884966214677968, 1.000000000000000000),
 ( 1.000000000000000000, 0.7174883642158075281, 1.000000000000000000),
 ( 1.000000000000000000, 0.7180610417773349852, 1.000000000000000000),
 ( 1.000000000000000000, 0.7187540717311197147, 1.000000000000000000) ) ) 
 REPRESENTATION_ITEM ( '' )  SURFACE ( )  );
#35918=CARTESIAN_POINT ( 'NONE',  ( -8.955454528939414516, 3.019799309333212722, -8.063527476382400749 ) ) ;
#35921=ORIENTED_EDGE ( 'NONE', *, *, #28829, .F. ) ;
#35957=ORIENTED_EDGE ( 'NONE', *, *, #29125, .F. ) ;
#35964=DIRECTION ( 'NONE',  ( -0.000000000000000000, -1.000000000000000000, -0.000000000000000000 ) ) ;
#35981=CARTESIAN_POINT ( 'NONE',  ( 10.23394195678221763, -9.091017468561378934, -0.1786341213271995521 ) ) ;
#35995=CARTESIAN_POINT ( 'NONE',  ( -8.673617379884035472E-15, 3.507114751586604129, -11.99288524841337455 ) ) ;
#36008=EDGE_CURVE ( 'NONE', #159583, #138893, #54087, .T. ) ;
#36033=CARTESIAN_POINT ( 'NONE',  ( -11.18654035131441127, 1.000000000000000888, 4.041720556560751021 ) ) ;
#36034=DIRECTION ( 'NONE',  ( 0.000000000000000000, 0.000000000000000000, 1.000000000000000000 ) ) ;
#36083=VERTEX_POINT ( 'NONE', #183006 ) ;
#36125=CARTESIAN_POINT ( 'NONE',  ( 6.392587740394330531, -6.532648833121157850, 6.999862025036990509 ) ) ;
#36126=ORIENTED_EDGE ( 'NONE', *, *, #153215, .T. ) ;
#36152=EDGE_CURVE ( 'NONE', #169714, #143658, #45780, .T. ) ;
#36167=MECHANICAL_DESIGN_GEOMETRIC_PRESENTATION_REPRESENTATION('',(#91564),#67377);
#36176=CARTESIAN_POINT ( 'NONE',  ( -0.4355862708379995563, -6.583980363595115293, -9.606148981167580203 ) ) ;
#36183=CARTESIAN_POINT ( 'NONE',  ( -10.96562622554683664, -5.341077028191769216, 0.1833053738655391618 ) ) ;
#36207=DIRECTION ( 'NONE',  ( 0.000000000000000000, 1.000000000000000000, 0.000000000000000000 ) ) ;
#36218=DIRECTION ( 'NONE',  ( 0.9988044021632737079, 8.339466111204228823E-16, -0.04888523518676889112 ) ) ;
#36239=CARTESIAN_POINT ( 'NONE',  ( -6.761775799040186996, -7.009934032700144257, -6.672971353127118199 ) ) ;
#36247=CARTESIAN_POINT ( 'NONE',  ( 0.3106162252735343854, -6.604184692106362498, 9.611175950047659455 ) ) ;
#36256=AXIS2_PLACEMENT_3D ( 'NONE', #196111, #193959, #33591 ) ;
#36287=CYLINDRICAL_SURFACE ( 'NONE', #120755, 0.09999999999999990841 ) ;
#36300=DIRECTION ( 'NONE',  ( 0.000000000000000000, -1.000000000000000000, 0.000000000000000000 ) ) ;
#36336=CARTESIAN_POINT ( 'NONE',  ( 10.45358220256315285, 1.000000000000000888, -5.892590188894412329 ) ) ;
#36376=EDGE_CURVE ( 'NONE', #12663, #1871, #38086, .T. ) ;
#36416=AXIS2_PLACEMENT_3D ( 'NONE', #132195, #15187, #162544 ) ;
#36426=CARTESIAN_POINT ( 'NONE',  ( -9.623628927379540343, -9.094708467121344952, 0.4567741993462124950 ) ) ;
#36430=ADVANCED_FACE ( 'NONE', ( #3461 ), #201659, .T. ) ;
#36439=CARTESIAN_POINT ( 'NONE',  ( -8.043985462411137988, -6.893136966056773396, 7.503460210123606977 ) ) ;
#36441=B_SPLINE_CURVE_WITH_KNOTS ( 'NONE', 3,
 ( #190954, #209327, #126057, #26327, #107660, #176863, #25265, #43682, #45816, #60974 ),
 .UNSPECIFIED., .F., .F.,
 ( 4, 2, 2, 2, 4 ),
 ( 0.000000000000000000, 0.0002216178067634645894, 0.0004432356135269291788, 0.0006648534202903938223, 0.0008864712270538583575 ),
 .UNSPECIFIED. ) ;
#36443=DIRECTION ( 'NONE',  ( 0.000000000000000000, 1.000000000000000000, 0.000000000000000000 ) ) ;
#36518=FACE_OUTER_BOUND ( 'NONE', #186431, .T. ) ;
#36550=DIRECTION ( 'NONE',  ( 0.000000000000000000, -1.000000000000000000, 0.000000000000000000 ) ) ;
#36602=AXIS2_PLACEMENT_3D ( 'NONE', #58859, #90304, #74049 ) ;
#36622=AXIS2_PLACEMENT_3D ( 'NONE', #37589, #203266, #151352 ) ;
#36643=CARTESIAN_POINT ( 'NONE',  ( -9.579665964948885559, -7.473374494045003757, 1.020505294851981049E-14 ) ) ;
#36647=VERTEX_POINT ( 'NONE', #174555 ) ;
#36677=CARTESIAN_POINT ( 'NONE',  ( -0.3561222683123435040, -6.532648913095006726, -9.473215147174805395 ) ) ;
#36686=CARTESIAN_POINT ( 'NONE',  ( -7.721398836998378812, -6.134628647623499909, 7.721398836998403681 ) ) ;
#36692=COLOUR_RGB ( '', 0.72549020, 0.75294118, 0.79215686) ;
#36719=DIRECTION ( 'NONE',  ( 0.000000000000000000, -1.000000000000000000, 0.000000000000000000 ) ) ;
#36732=CARTESIAN_POINT ( 'NONE',  ( 0.07999999999998980149, -6.134628647623513231, -10.91970695577493977 ) ) ;
#36734=( BOUNDED_SURFACE ( )  B_SPLINE_SURFACE ( 3, 2, ( 
 ( #125879, #128025, #157240 ),
 ( #74912, #45627, #177750 ),
 ( #195056, #207029, #58658 ),
 ( #124811, #108541, #30438 ),
 ( #34672, #97579, #84493 ),
 ( #32552, #98628, #48816 ),
 ( #134353, #132224, #164689 ),
 ( #16273, #166824, #113886 ) ),
 .UNSPECIFIED., .F., .F., .T. ) 
 B_SPLINE_SURFACE_WITH_KNOTS ( ( 4, 2, 2, 4 ),
 ( 3, 3 ),
 ( 0.000000000000000000, 0.0005109843281227146802, 0.0007664764921840720203, 0.001021968656245429360 ),
 ( 0.000000000000000000, 1.000000000000000000 ),
 .UNSPECIFIED. ) 
 GEOMETRIC_REPRESENTATION_ITEM ( )  RATIONAL_B_SPLINE_SURFACE ( (
 ( 1.000000000000000000, 0.7045118851637687252, 1.000000000000000000),
 ( 1.000000000000000000, 0.6478559580219998004, 1.000000000000000000),
 ( 1.000000000000000000, 0.5832506164449653419, 1.000000000000000000),
 ( 1.000000000000000000, 0.4879709628488582140, 1.000000000000000000),
 ( 1.000000000000000000, 0.4561823831828598630, 1.000000000000000000),
 ( 1.000000000000000000, 0.4039565156453471806, 1.000000000000000000),
 ( 1.000000000000000000, 0.3848936348732069912, 1.000000000000000000),
 ( 1.000000000000000000, 0.3826834323650904479, 1.000000000000000000) ) ) 
 REPRESENTATION_ITEM ( '' )  SURFACE ( )  );
#36750=CARTESIAN_POINT ( 'NONE',  ( -0.07933194154489606187, -9.900000000000005684, -9.499668754385620417 ) ) ;
#36759=CARTESIAN_POINT ( 'NONE',  ( 0.4694063952341813728, -6.893137084989856334, 10.98997987423603995 ) ) ;
#36775=CARTESIAN_POINT ( 'NONE',  ( -10.91804383151481339, -8.407420853759283830, 0.1905751639681794174 ) ) ;
#36783=CYLINDRICAL_SURFACE ( 'NONE', #151542, 11.49999999999998934 ) ;
#36819=SURFACE_STYLE_FILL_AREA ( #3236 ) ;
#36856=PLANE ( 'NONE',  #95737 ) ;
#36867=CARTESIAN_POINT ( 'NONE',  ( 9.827407719474571479, -6.362962251424049143, -0.4359508081058064421 ) ) ;
#36895=CARTESIAN_POINT ( 'NONE',  ( -6.818239715405332468, -6.631671885544856870, 6.594971855056608767 ) ) ;
#36914=AXIS2_PLACEMENT_3D ( 'NONE', #38645, #155599, #138291 ) ;
#36941=AXIS2_PLACEMENT_3D ( 'NONE', #63243, #146660, #95773 ) ;
#36942=CARTESIAN_POINT ( 'NONE',  ( -2.331034670843834533E-15, -8.526088927971001041, -10.80093815994595730 ) ) ;
#36953=CARTESIAN_POINT ( 'NONE',  ( -0.4655551865852154414, -8.176568542494919711, -9.512045263456256450 ) ) ;
#36956=CARTESIAN_POINT ( 'NONE',  ( 9.622374086701777074, -9.063146643177445227, -0.5328106107931120938 ) ) ;
#36959=CARTESIAN_POINT ( 'NONE',  ( 9.469892045836674654, -6.532648833121171172, -0.4294077647110511320 ) ) ;
#36973=DIRECTION ( 'NONE',  ( 0.000000000000000000, 1.000000000000000000, 0.000000000000000000 ) ) ;
#37010=VERTEX_POINT ( 'NONE', #153750 ) ;
#37026=CARTESIAN_POINT ( 'NONE',  ( 0.3591838038534900801, -8.233137084989865073, 9.493791972417897185 ) ) ;
#37031=CARTESIAN_POINT ( 'NONE',  ( -0.08000000000000367928, -7.473374494045017968, 9.579665964948883783 ) ) ;
#37046=DIRECTION ( 'NONE',  ( 0.000000000000000000, 0.000000000000000000, 1.000000000000000000 ) ) ;
#37055=CARTESIAN_POINT ( 'NONE',  ( 6.500815856195029774, -6.554751173179699464, 6.901817412891874781 ) ) ;
#37059=ORIENTED_EDGE ( 'NONE', *, *, #85823, .T. ) ;
#37063=CARTESIAN_POINT ( 'NONE',  ( 10.99946651476068205, -9.910601012391426323, -0.1083346235443097966 ) ) ;
#37067=CARTESIAN_POINT ( 'NONE',  ( 7.055786748302883993, -6.583711766989194913, -6.534012848837080334 ) ) ;
#37072=( GEOMETRIC_REPRESENTATION_CONTEXT ( 3 ) GLOBAL_UNCERTAINTY_ASSIGNED_CONTEXT ( ( #42268 ) ) GLOBAL_UNIT_ASSIGNED_CONTEXT ( ( #55053, #57186, #58252 ) ) REPRESENTATION_CONTEXT ( 'NONE', 'WORKASPACE' ) );
#37081=LINE ( 'NONE', #169221, #18309 ) ;
#37096=ADVANCED_FACE ( 'NONE', ( #2129 ), #68204, .F. ) ;
#37105=CARTESIAN_POINT ( 'NONE',  ( 0.06263693352612137444, -7.008128100062071653, -9.499802063084663573 ) ) ;
#37106=B_SPLINE_CURVE_WITH_KNOTS ( 'NONE', 3,
 ( #85789, #151870, #38112, #201640, #69511, #53288, #152922, #119421 ),
 .UNSPECIFIED., .F., .F.,
 ( 4, 2, 2, 4 ),
 ( 0.000000000000000000, 0.0004365159022975865317, 0.0006547738534463801770, 0.0008730318045951738224 ),
 .UNSPECIFIED. ) ;
#37148=EDGE_CURVE ( 'NONE', #193127, #195818, #89717, .T. ) ;
#37195=ADVANCED_FACE ( 'NONE', ( #185158 ), #36783, .T. ) ;
#37223=CYLINDRICAL_SURFACE ( 'NONE', #150023, 11.99999999999999112 ) ;
#37232=CARTESIAN_POINT ( 'NONE',  ( 7.681709917290610257, -6.443545996361870642, 7.726139724254744046 ) ) ;
#37277=CARTESIAN_POINT ( 'NONE',  ( 0.4359507092142514972, -8.863025497814007281, -9.827344407697072626 ) ) ;
#37305=ORIENTED_EDGE ( 'NONE', *, *, #213004, .F. ) ;
#37317=CARTESIAN_POINT ( 'NONE',  ( -6.645879322773616593, -6.896483513897168294, -6.785280070212523107 ) ) ;
#37326=CARTESIAN_POINT ( 'NONE',  ( 0.000000000000000000, 0.000000000000000000, 9.579665964948883783 ) ) ;
#37333=CONICAL_SURFACE ( 'NONE', #9653, 11.53746066217573762, 0.1181278931043537039 ) ;
#37376=FILL_AREA_STYLE_COLOUR ( '', #11471 ) ;
#37468=CARTESIAN_POINT ( 'NONE',  ( -10.38614328979765489, 3.507114751586604129, -5.996442624206661520 ) ) ;
#37492=AXIS2_PLACEMENT_3D ( 'NONE', #114066, #28467, #160601 ) ;
#37499=CARTESIAN_POINT ( 'NONE',  ( 0.000000000000000000, -1.000000000000000888, 0.000000000000000000 ) ) ;
#37501=DIRECTION ( 'NONE',  ( -0.7071067811865489050, 0.000000000000000000, -0.7071067811865462405 ) ) ;
#37516=CARTESIAN_POINT ( 'NONE',  ( -0.4645879757425588341, -7.605490376146412324, -10.08385597498927488 ) ) ;
#37539=CARTESIAN_POINT ( 'NONE',  ( -10.39230484541323563, 3.038454817776168770, 6.000000000000048850 ) ) ;
#37589=CARTESIAN_POINT ( 'NONE',  ( 0.000000000000000000, 0.000000000000000000, 0.000000000000000000 ) ) ;
#37624=CARTESIAN_POINT ( 'NONE',  ( -7.045261094876551944, -5.790678129197933899, -7.662794434365294727 ) ) ;
#37646=CARTESIAN_POINT ( 'NONE',  ( -10.91804381884000641, -9.954640477432109336, 0.1905751637469953186 ) ) ;
#37701=DIRECTION ( 'NONE',  ( 0.000000000000000000, 0.000000000000000000, 1.000000000000000000 ) ) ;
#37719=ORIENTED_EDGE ( 'NONE', *, *, #52063, .T. ) ;
#37726=ORIENTED_EDGE ( 'NONE', *, *, #140961, .F. ) ;
#37731=FILL_AREA_STYLE ('',( #188236 ) ) ;
#37739=B_SPLINE_CURVE_WITH_KNOTS ( 'NONE', 3,
 ( #29192, #63816, #13977, #144053, #163464, #77932, #210048, #113711 ),
 .UNSPECIFIED., .F., .F.,
 ( 4, 2, 2, 4 ),
 ( 1.734723475976852932E-18, 0.0002034531274099198050, 0.0004069062548198378753, 0.0008138125096396721728 ),
 .UNSPECIFIED. ) ;
#37760=CARTESIAN_POINT ( 'NONE',  ( -0.3912817730721762643, -6.709848117146501423, -9.483257663144962990 ) ) ;
#37792=DIRECTION ( 'NONE',  ( 0.000000000000000000, 0.000000000000000000, -1.000000000000000000 ) ) ;
#37795=ORIENTED_EDGE ( 'NONE', *, *, #117997, .F. ) ;
#37822=CARTESIAN_POINT ( 'NONE',  ( 0.000000000000000000, 1.000000000000000888, 0.000000000000000000 ) ) ;
#37827=EDGE_CURVE ( 'NONE', #86684, #68781, #193058, .T. ) ;
#37829=CARTESIAN_POINT ( 'NONE',  ( 7.927630635717423324, -6.615717645446945738, -7.626802973668249663 ) ) ;
#37840=CARTESIAN_POINT ( 'NONE',  ( 0.2118258318327995438, -6.614835951978765394, 10.99866081003794527 ) ) ;
#37862=EDGE_CURVE ( 'NONE', #33092, #114840, #57347, .T. ) ;
#37863=DIRECTION ( 'NONE',  ( 0.000000000000000000, -1.000000000000000000, 0.000000000000000000 ) ) ;
#37896=AXIS2_PLACEMENT_3D ( 'NONE', #95902, #145736, #127395 ) ;
#37911=DIRECTION ( 'NONE',  ( 0.9990890794760038940, 0.000000000000000000, -0.04267330865764931702 ) ) ;
#37920=DIRECTION ( 'NONE',  ( -1.224646799147355426E-16, 0.000000000000000000, -1.000000000000000000 ) ) ;
#37940=EDGE_LOOP ( 'NONE', ( #105698, #162490, #131327, #117046, #123551 ) ) ;
#37941=DIRECTION ( 'NONE',  ( 0.000000000000000000, 1.000000000000000000, 0.000000000000000000 ) ) ;
#37952=CARTESIAN_POINT ( 'NONE',  ( 10.14529669463207640, -6.681160345271552892, 9.269928574751062911E-15 ) ) ;
#37977=CARTESIAN_POINT ( 'NONE',  ( -6.956254272497635505, -6.713678229394818509, 6.457408393014306469 ) ) ;
#37979=CARTESIAN_POINT ( 'NONE',  ( -8.724804694929160327E-15, -6.594478602028689629, -10.23203630735469893 ) ) ;
#38016=DIRECTION ( 'NONE',  ( -0.05727394217551152328, -1.062425134715125641E-15, -0.9983585005135562351 ) ) ;
#38018=ORIENTED_EDGE ( 'NONE', *, *, #31446, .F. ) ;
#38023=CARTESIAN_POINT ( 'NONE',  ( -7.860745937262166194, -5.389939693150854971, 7.694877102302390526 ) ) ;
#38040=CARTESIAN_POINT ( 'NONE',  ( -2.493461049780994365, 3.507114751586604129, 11.73081193161140590 ) ) ;
#38061=AXIS2_PLACEMENT_3D ( 'NONE', #788, #32270, #49578 ) ;
#38065=EDGE_CURVE ( 'NONE', #35700, #54210, #124420, .T. ) ;
#38069=CARTESIAN_POINT ( 'NONE',  ( -7.505515594164280380, -6.699677480913956096, -8.042162931142907922 ) ) ;
#38086=B_SPLINE_CURVE_WITH_KNOTS ( 'NONE', 3,
 ( #1328, #118371, #35981, #38130, #121593, #102062, #186499 ),
 .UNSPECIFIED., .F., .F.,
 ( 4, 3, 4 ),
 ( 0.0001126021369344445543, 0.001503110988946918273, 0.002006790696425510192 ),
 .UNSPECIFIED. ) ;
#38102=CARTESIAN_POINT ( 'NONE',  ( 2.093037498677865482, 1.000000000000000888, -11.70868840297833025 ) ) ;
#38103=CARTESIAN_POINT ( 'NONE',  ( -2.331034670843834533E-15, -5.530538574611992608, 11.29689844398642684 ) ) ;
#38105=ORIENTED_EDGE ( 'NONE', *, *, #91274, .T. ) ;
#38112=CARTESIAN_POINT ( 'NONE',  ( -6.729185404178093854, -6.864242587301021103, -6.701130199342132165 ) ) ;
#38130=CARTESIAN_POINT ( 'NONE',  ( 10.56178662260467682, -8.763419982614969683, -0.1843566712554992049 ) ) ;
#38139=CARTESIAN_POINT ( 'NONE',  ( 6.645879322773626363, -6.896483513897670115, 6.785280070212115433 ) ) ;
#38171=CARTESIAN_POINT ( 'NONE',  ( -0.001932266794912151702, -9.922538451904662438, -9.579662758527177857 ) ) ;
#38224=CARTESIAN_POINT ( 'NONE',  ( 0.08058962652511190983, -9.910877166163974294, 10.99970478295254850 ) ) ;
#38231=FACE_OUTER_BOUND ( 'NONE', #138444, .T. ) ;
#38236=FACE_OUTER_BOUND ( 'NONE', #195230, .T. ) ;
#38249=ADVANCED_FACE ( 'NONE', ( #135531 ), #213062, .T. ) ;
#38260=LINE ( 'NONE', #171458, #165598 ) ;
#38300=CARTESIAN_POINT ( 'NONE',  ( -6.781144757626070607, -7.161464053357452286, 6.776370306708066060 ) ) ;
#38304=EDGE_CURVE ( 'NONE', #98224, #81410, #33100, .T. ) ;
#38314=AXIS2_PLACEMENT_3D ( 'NONE', #100026, #3557, #54477 ) ;
#38336=B_SPLINE_CURVE_WITH_KNOTS ( 'NONE', 3,
 ( #212304, #100696, #133236, #49820, #33565, #183010 ),
 .UNSPECIFIED., .F., .F.,
 ( 4, 2, 4 ),
 ( 0.000000000000000000, 0.001225895755212360379, 0.002451791510424721193 ),
 .UNSPECIFIED. ) ;
#38342=CARTESIAN_POINT ( 'NONE',  ( 10.91962425643211709, -9.999999999999998224, -0.09058751758337030280 ) ) ;
#38347=ORIENTED_EDGE ( 'NONE', *, *, #164350, .F. ) ;
#38360=ORIENTED_EDGE ( 'NONE', *, *, #4172, .T. ) ;
#38388=CARTESIAN_POINT ( 'NONE',  ( -6.531918710724228916, -6.583723166013396799, -7.057683771862738986 ) ) ;
#38398=CARTESIAN_POINT ( 'NONE',  ( 0.03636482241361622264, -7.019129742887146861, 9.500587730661987251 ) ) ;
#38423=EDGE_CURVE ( 'NONE', #61589, #74349, #206106, .T. ) ;
#38436=FACE_OUTER_BOUND ( 'NONE', #3197, .T. ) ;
#38458=CARTESIAN_POINT ( 'NONE',  ( -11.00039779440762899, -6.304807775344881904, 0.01400375819670464893 ) ) ;
#38511=CIRCLE ( 'NONE', #149198, 10.97656854249491687 ) ;
#38552=CARTESIAN_POINT ( 'NONE',  ( 10.99943592145024951, -8.241816521215563185, -0.1113975309864851937 ) ) ;
#38553=AXIS2_PLACEMENT_3D ( 'NONE', #43203, #142844, #174271 ) ;
#38569=CARTESIAN_POINT ( 'NONE',  ( 6.396834479292349052, -8.176568542494905500, 7.055228938194280985 ) ) ;
#38571=B_SPLINE_CURVE_WITH_KNOTS ( 'NONE', 3,
 ( #169452, #53571, #168390, #40540, #202997, #19986, #104468, #23177 ),
 .UNSPECIFIED., .F., .F.,
 ( 4, 2, 2, 4 ),
 ( 0.000000000000000000, 0.0004970278158210180916, 0.0007455417237315293058, 0.0009940556316420405200 ),
 .UNSPECIFIED. ) ;
#38609=ORIENTED_EDGE ( 'NONE', *, *, #70817, .F. ) ;
#38611=ORIENTED_EDGE ( 'NONE', *, *, #109273, .F. ) ;
#38645=CARTESIAN_POINT ( 'NONE',  ( -0.08000000000000194456, -9.900000000000005684, -10.91970695577494865 ) ) ;
#38656=CARTESIAN_POINT ( 'NONE',  ( -9.481437597266051398, -6.708819892820502950, 0.4299312922663448555 ) ) ;
#38710=ORIENTED_EDGE ( 'NONE', *, *, #76837, .T. ) ;
#38720=FACE_OUTER_BOUND ( 'NONE', #117786, .T. ) ;
#38751=AXIS2_PLACEMENT_3D ( 'NONE', #143897, #74592, #140695 ) ;
#38788=ORIENTED_EDGE ( 'NONE', *, *, #29409, .T. ) ;
#38800=CARTESIAN_POINT ( 'NONE',  ( 10.91962425643199985, -9.999999999999994671, -0.09058751758333170867 ) ) ;
#38816=CARTESIAN_POINT ( 'NONE',  ( -0.4359479416626658721, -6.334709917115479705, -9.855659161987901484 ) ) ;
#38817=B_SPLINE_CURVE_WITH_KNOTS ( 'NONE', 3,
 ( #53665, #52595, #88307, #187916 ),
 .UNSPECIFIED., .F., .F.,
 ( 4, 4 ),
 ( 1.113895019748840813E-15, 8.505390839970735750E-05 ),
 .UNSPECIFIED. ) ;
#38828=CARTESIAN_POINT ( 'NONE',  ( -0.03636482241158912887, -7.019129742886503820, -9.500587730666937958 ) ) ;
#38841=CARTESIAN_POINT ( 'NONE',  ( -0.3532572990641859034, -7.666862990898835051, 10.99465531782957939 ) ) ;
#38898=CARTESIAN_POINT ( 'NONE',  ( 7.749822179018763357, -6.479141885268237644, -7.806953216197509704 ) ) ;
#38908=B_SPLINE_CURVE_WITH_KNOTS ( 'NONE', 3,
 ( #12906, #124639, #109440, #112633 ),
 .UNSPECIFIED., .F., .F.,
 ( 4, 4 ),
 ( 0.000000000000000000, 8.505390838610257180E-05 ),
 .UNSPECIFIED. ) ;
#38922=CARTESIAN_POINT ( 'NONE',  ( -9.486581398170532253, -9.006862915010220405, 0.5116190538792247944 ) ) ;
#38951=CARTESIAN_POINT ( 'NONE',  ( 10.96964784646768010, -7.712340523144908921, -0.6288774950739197678 ) ) ;
#38980=VERTEX_POINT ( 'NONE', #201294 ) ;
#38981=CARTESIAN_POINT ( 'NONE',  ( -10.56178662260468393, -8.763419982614969683, 0.1843566712555078646 ) ) ;
#38991=ORIENTED_EDGE ( 'NONE', *, *, #78185, .T. ) ;
#39000=CARTESIAN_POINT ( 'NONE',  ( -9.716492259128738596, -7.972382850425317358, 0.4652101495396395170 ) ) ;
#39010=( NAMED_UNIT ( * ) PLANE_ANGLE_UNIT ( ) SI_UNIT ( $, .RADIAN. ) );
#39071=ADVANCED_FACE ( 'NONE', ( #154718 ), #138452, .T. ) ;
#39077=AXIS2_PLACEMENT_3D ( 'NONE', #13500, #178156, #144621 ) ;
#39129=DIRECTION ( 'NONE',  ( 0.000000000000000000, 0.000000000000000000, -1.000000000000000000 ) ) ;
#39142=ORIENTED_EDGE ( 'NONE', *, *, #107850, .F. ) ;
#39160=CARTESIAN_POINT ( 'NONE',  ( 0.07999999999999327094, -9.746166700180788567, 9.579665964948873125 ) ) ;
#39199=CARTESIAN_POINT ( 'NONE',  ( 6.392587740394325202, -6.532648833121162291, 6.999862025037000279 ) ) ;
#39236=ORIENTED_EDGE ( 'NONE', *, *, #49632, .T. ) ;
#39238=CIRCLE ( 'NONE', #4566, 0.08000000000000020983 ) ;
#39239=ORIENTED_EDGE ( 'NONE', *, *, #50950, .T. ) ;
#39263=VERTEX_POINT ( 'NONE', #61475 ) ;
#39291=( LENGTH_UNIT ( ) NAMED_UNIT ( * ) SI_UNIT ( .MILLI., .METRE. ) );
#39292=CARTESIAN_POINT ( 'NONE',  ( -11.41267819554183127, 4.000000000000003553, 3.708203932499423150 ) ) ;
#39297=FILL_AREA_STYLE_COLOUR ( '', #167127 ) ;
#39301=CARTESIAN_POINT ( 'NONE',  ( 1.972527975918452161E-16, -7.473374494045017968, -9.500331257164628340 ) ) ;
#39325=CARTESIAN_POINT ( 'NONE',  ( -9.499668754385629299, -7.215597533182398493, -0.07933194154558173561 ) ) ;
#39327=VECTOR ( 'NONE', #62489, 1000.000000000000000 ) ;
#39368=CARTESIAN_POINT ( 'NONE',  ( 7.591565991045856165, -6.646943093534003033, 7.792125355486806626 ) ) ;
#39388=CARTESIAN_POINT ( 'NONE',  ( 0.000000000000000000, 3.079999999999999183, 0.000000000000000000 ) ) ;
#39400=B_SPLINE_CURVE_WITH_KNOTS ( 'NONE', 3,
 ( #171032, #204576, #122387, #89817, #200318, #51969 ),
 .UNSPECIFIED., .F., .F.,
 ( 4, 2, 4 ),
 ( 0.000000000000000000, 0.0002835903134653135075, 0.0005671806269306270149 ),
 .UNSPECIFIED. ) ;
#39414=ORIENTED_EDGE ( 'NONE', *, *, #19442, .F. ) ;
#39425=DIRECTION ( 'NONE',  ( 0.000000000000000000, 0.000000000000000000, 1.000000000000000000 ) ) ;
#39441=ORIENTED_EDGE ( 'NONE', *, *, #131051, .F. ) ;
#39450=CARTESIAN_POINT ( 'NONE',  ( 7.808923410443484592, -5.575271019048062549, 7.747753938335146806 ) ) ;
#39454=DIRECTION ( 'NONE',  ( 0.000000000000000000, 1.000000000000000000, 0.000000000000000000 ) ) ;
#39457=EDGE_CURVE ( 'NONE', #37010, #148901, #206648, .T. ) ;
#39463=CARTESIAN_POINT ( 'NONE',  ( 7.720982897393566802, -6.134628647623485698, -7.834948825496929281 ) ) ;
#39500=DIRECTION ( 'NONE',  ( -0.7431448254774005724, 0.000000000000000000, -0.6691306063588511321 ) ) ;
#39506=ORIENTED_EDGE ( 'NONE', *, *, #189032, .T. ) ;
#39511=ADVANCED_FACE ( 'NONE', ( #145961 ), #199985, .T. ) ;
#39521=CARTESIAN_POINT ( 'NONE',  ( -10.98997987423604172, -6.893137084989856334, 0.4694063952341883672 ) ) ;
#39578=TOROIDAL_SURFACE ( 'NONE', #150146, 10.92000000000000171, 0.08000000000000000167 ) ;
#39652=CARTESIAN_POINT ( 'NONE',  ( -10.54982673430220608, -8.131911363926706215, 0.6210660986541721718 ) ) ;
#39699=EDGE_LOOP ( 'NONE', ( #172075, #28360, #69322, #173038 ) ) ;
#39717=TOROIDAL_SURFACE ( 'NONE', #157400, 9.559451093910102060, 0.08000000000000000167 ) ;
#39723=ORIENTED_EDGE ( 'NONE', *, *, #89254, .F. ) ;
#39728=STYLED_ITEM ( 'NONE', ( #151478 ), #86557 ) ;
#39753=CARTESIAN_POINT ( 'NONE',  ( 11.25751254300906723, -6.452016313277396442, 9.269928574751062911E-15 ) ) ;
#39776=CARTESIAN_POINT ( 'NONE',  ( 0.000000000000000000, 0.03624871340549007392, -6.329999999999995630 ) ) ;
#39875=CARTESIAN_POINT ( 'NONE',  ( 10.91850271852025500, -9.971093637360025852, -0.1617895344457838669 ) ) ;
#39890=CARTESIAN_POINT ( 'NONE',  ( -6.818239719371408825, -6.631671897293992757, 6.594971851908693061 ) ) ;
#39905=CARTESIAN_POINT ( 'NONE',  ( -0.1588444833727709893, -6.630981389236889179, -9.484513307599968357 ) ) ;
#39920=EDGE_CURVE ( 'NONE', #196061, #149524, #130973, .T. ) ;
#39944=ORIENTED_EDGE ( 'NONE', *, *, #111631, .T. ) ;
#39965=B_SPLINE_CURVE_WITH_KNOTS ( 'NONE', 3,
 ( #163786, #145439, #115086, #31652, #110819, #16429, #111898, #79322 ),
 .UNSPECIFIED., .F., .F.,
 ( 4, 2, 2, 4 ),
 ( 0.000000000000000000, 0.0002567066673176287726, 0.0005134133346352575452, 0.001026826669270511404 ),
 .UNSPECIFIED. ) ;
#39983=CARTESIAN_POINT ( 'NONE',  ( 0.1531059978909261043, -6.764708007038248816, 10.99917004716958857 ) ) ;
#39986=ORIENTED_EDGE ( 'NONE', *, *, #49632, .F. ) ;
#40097=EDGE_CURVE ( 'NONE', #163559, #16492, #43093, .T. ) ;
#40127=ORIENTED_EDGE ( 'NONE', *, *, #160637, .T. ) ;
#40132=VERTEX_POINT ( 'NONE', #73184 ) ;
#40139=CARTESIAN_POINT ( 'NONE',  ( 0.000000000000000000, 3.000000000000000888, -6.329999999999995630 ) ) ;
#40175=DIRECTION ( 'NONE',  ( -0.007014632059889177630, 0.000000000000000000, -0.9999753971658824625 ) ) ;
#40200=CARTESIAN_POINT ( 'NONE',  ( -6.549078289569701283, -6.948428148671524696, 6.549078289569724376 ) ) ;
#40201=CARTESIAN_POINT ( 'NONE',  ( 9.579665964948882007, -7.473374494045003757, 1.734723475976807094E-15 ) ) ;
#40236=CARTESIAN_POINT ( 'NONE',  ( 6.825099317097807372, -8.105676417795693922, -6.608557002163611749 ) ) ;
#40238=CARTESIAN_POINT ( 'NONE',  ( 2.020417662918754687, 3.956598013261175772, -11.36521191596581737 ) ) ;
#40243=EDGE_LOOP ( 'NONE', ( #103237, #49351, #15970, #64840 ) ) ;
#40258=DIRECTION ( 'NONE',  ( 0.000000000000000000, 0.7071067811865432429, 0.7071067811865517916 ) ) ;
#40262=CARTESIAN_POINT ( 'NONE',  ( 6.661184041420940005, -7.215597533173327527, -6.773376349083132908 ) ) ;
#40278=CARTESIAN_POINT ( 'NONE',  ( 0.008219159353561588180, -7.627132808484223148, 9.567202289542827032 ) ) ;
#40289=DIRECTION ( 'NONE',  ( 0.000000000000000000, 0.000000000000000000, 1.000000000000000000 ) ) ;
#40316=CARTESIAN_POINT ( 'NONE',  ( -0.07804408512528809849, -9.997559919034475939, -9.579522898042005963 ) ) ;
#40322=ORIENTED_EDGE ( 'NONE', *, *, #49463, .F. ) ;
#40352=ADVANCED_FACE ( 'NONE', ( #53757 ), #72113, .F. ) ;
#40383=VERTEX_POINT ( 'NONE', #114053 ) ;
#40446=EDGE_LOOP ( 'NONE', ( #45438, #21366, #70838, #62490, #74152, #186619 ) ) ;
#40466=CARTESIAN_POINT ( 'NONE',  ( -0.005636871015592820333, -9.933099847254503345, -10.91969863820289177 ) ) ;
#40467=COLOUR_RGB ( '', 0.72549020, 0.75294118, 0.79215686) ;
#40474=FACE_OUTER_BOUND ( 'NONE', #163144, .T. ) ;
#40497=CARTESIAN_POINT ( 'NONE',  ( -2.331034670843834533E-15, -9.181223591647247773, -10.14523337821909976 ) ) ;
#40534=ORIENTED_EDGE ( 'NONE', *, *, #115776, .F. ) ;
#40540=CARTESIAN_POINT ( 'NONE',  ( 10.99663476780025206, -7.859187537802522883, -0.2753234695294711765 ) ) ;
#40562=CARTESIAN_POINT ( 'NONE',  ( -0.4638907948587486785, -7.079050064870612502, -10.61081979358357330 ) ) ;
#40611=CARTESIAN_POINT ( 'NONE',  ( -2.474997580123502683, 0.9706168436483498807, 11.64394813633530390 ) ) ;
#40635=UNCERTAINTY_MEASURE_WITH_UNIT (LENGTH_MEASURE( 1.000000000000000082E-05 ), #90258, 'distance_accuracy_value', 'NONE');
#40666=CARTESIAN_POINT ( 'NONE',  ( -0.09411116651288103929, -9.919020924439822195, -10.99959762541856811 ) ) ;
#40670=EDGE_LOOP ( 'NONE', ( #207171, #33600, #48500 ) ) ;
#40684=CARTESIAN_POINT ( 'NONE',  ( -10.33323920393391582, 4.021557182957058885, 5.965898435992110116 ) ) ;
#40687=EDGE_LOOP ( 'NONE', ( #50652, #83734, #109849, #9808, #18876 ) ) ;
#40743=DIRECTION ( 'NONE',  ( -0.000000000000000000, -1.000000000000000000, -0.000000000000000000 ) ) ;
#40750=FILL_AREA_STYLE ('',( #171799 ) ) ;
#40762=ADVANCED_FACE ( 'NONE', ( #50039 ), #65376, .T. ) ;
#40766=VECTOR ( 'NONE', #63424, 1000.000000000000000 ) ;
#40768=DIRECTION ( 'NONE',  ( 0.000000000000000000, -1.000000000000000000, 0.000000000000000000 ) ) ;
#40773=CARTESIAN_POINT ( 'NONE',  ( 2.493461049780987260, 3.507114751586604129, -11.73081193161139169 ) ) ;
#40783=ORIENTED_EDGE ( 'NONE', *, *, #202457, .T. ) ;
#40810=CARTESIAN_POINT ( 'NONE',  ( 9.578206935422374002, -9.900000000000074962, -0.1671882239537531845 ) ) ;
#40813=SURFACE_STYLE_FILL_AREA ( #190229 ) ;
#40826=EDGE_CURVE ( 'NONE', #107467, #1301, #96523, .T. ) ;
#40836=CARTESIAN_POINT ( 'NONE',  ( -8.081892667527538876, -5.166862915010145052, 7.462104991928527831 ) ) ;
#40921=EDGE_CURVE ( 'NONE', #98224, #54631, #50717, .T. ) ;
#40925=COLOUR_RGB ( '', 0.40784314, 0.44705882, 0.49803922) ;
#40955=DIRECTION ( 'NONE',  ( 0.000000000000000000, 0.000000000000000000, 1.000000000000000000 ) ) ;
#40997=CARTESIAN_POINT ( 'NONE',  ( -0.1747071867222168284, -7.850481869465710361, 10.96497182194659104 ) ) ;
#41042=FACE_OUTER_BOUND ( 'NONE', #78205, .T. ) ;
#41050=CARTESIAN_POINT ( 'NONE',  ( 7.845789747616911392, -6.699703214240884996, -7.710100441483645817 ) ) ;
#41066=CARTESIAN_POINT ( 'NONE',  ( -1.858365260435290220E-15, -9.595263517168275413, -9.591985693222424558 ) ) ;
#41067=CARTESIAN_POINT ( 'NONE',  ( -7.487360338304386964, -6.465328379374276402, 7.487360338304412721 ) ) ;
#41080=( NAMED_UNIT ( * ) PLANE_ANGLE_UNIT ( ) SI_UNIT ( $, .RADIAN. ) );
#41100=VERTEX_POINT ( 'NONE', #87262 ) ;
#41101=AXIS2_PLACEMENT_3D ( 'NONE', #83534, #149616, #67261 ) ;
#41114=CARTESIAN_POINT ( 'NONE',  ( 9.561191386655707447, -9.006862915010142245, -0.6000160562356342542 ) ) ;
#41161=EDGE_LOOP ( 'NONE', ( #72180, #135788, #186607, #128139 ) ) ;
#41172=LINE ( 'NONE', #58467, #12737 ) ;
#41200=ORIENTED_EDGE ( 'NONE', *, *, #166038, .T. ) ;
#41229=CARTESIAN_POINT ( 'NONE',  ( -0.002323312721275774470, -7.217450603046129842, -9.500350659417616583 ) ) ;
#41240=CARTESIAN_POINT ( 'NONE',  ( -7.967649405165836640, -5.251137252134745914, 7.547231044119360632 ) ) ;
#41254=CARTESIAN_POINT ( 'NONE',  ( 10.99126615174920651, -5.166862915010145052, -0.4382560683119322009 ) ) ;
#41257=CARTESIAN_POINT ( 'NONE',  ( 9.579764304849151202, -9.919999999999998153, -0.06720017513373727214 ) ) ;
#41284=AXIS2_PLACEMENT_3D ( 'NONE', #100931, #128471, #18612 ) ;
#41285=CARTESIAN_POINT ( 'NONE',  ( 0.000000000000000000, -6.527411821100059797, 0.000000000000000000 ) ) ;
#41288=DIRECTION ( 'NONE',  ( 1.000000000000000000, -0.000000000000000000, 1.224646799147353207E-16 ) ) ;
#41295=CARTESIAN_POINT ( 'NONE',  ( -0.4330238300980990274, -6.527411821100045586, -9.549638505170015890 ) ) ;
#41310=CIRCLE ( 'NONE', #51655, 0.07999999999999982125 ) ;
#41314=EDGE_LOOP ( 'NONE', ( #191409, #50507, #123813, #154683, #116305 ) ) ;
#41319=CARTESIAN_POINT ( 'NONE',  ( 2.033424464989775249, 3.426985321572571852, -11.42673966862522583 ) ) ;
#41321=DIRECTION ( 'NONE',  ( 0.000000000000000000, 1.000000000000000000, 0.000000000000000000 ) ) ;
#41329=( GEOMETRIC_REPRESENTATION_CONTEXT ( 3 ) GLOBAL_UNCERTAINTY_ASSIGNED_CONTEXT ( ( #19012 ) ) GLOBAL_UNIT_ASSIGNED_CONTEXT ( ( #20529, #120253, #138574 ) ) REPRESENTATION_CONTEXT ( 'NONE', 'WORKASPACE' ) );
#41330=CARTESIAN_POINT ( 'NONE',  ( -10.99440753328290121, -7.824706741106413510, 0.3572413387872626633 ) ) ;
#41333=CIRCLE ( 'NONE', #131353, 11.49999999999998934 ) ;
#41340=CARTESIAN_POINT ( 'NONE',  ( 6.277139874739040337, -0.02379966007286238305, 9.660711923649619224E-16 ) ) ;
#41341=CARTESIAN_POINT ( 'NONE',  ( -10.99946651476068560, -9.910601012391426323, 0.1083346235443097966 ) ) ;
#41342=DIRECTION ( 'NONE',  ( 0.000000000000000000, 0.000000000000000000, 1.000000000000000000 ) ) ;
#41374=CARTESIAN_POINT ( 'NONE',  ( 0.000000000000000000, -6.893137084989842123, 0.000000000000000000 ) ) ;
#41390=CARTESIAN_POINT ( 'NONE',  ( -8.912450614902597934, 3.507114751586604129, -8.024806578263023127 ) ) ;
#41392=CARTESIAN_POINT ( 'NONE',  ( 8.002408263930250953, -6.836568542494980250, -7.346809171966436125 ) ) ;
#41516=SURFACE_STYLE_USAGE ( .BOTH. , #189874 ) ;
#41517=VERTEX_POINT ( 'NONE', #90480 ) ;
#41532=EDGE_CURVE ( 'NONE', #41837, #129023, #35372, .T. ) ;
#41549=CARTESIAN_POINT ( 'NONE',  ( 10.43625799253549857, 3.019799309333581316, 6.025376361322622998 ) ) ;
#41555=CARTESIAN_POINT ( 'NONE',  ( -10.93220419382131325, -5.754340240174524723, 1.121760655089042704E-14 ) ) ;
#41577=DIRECTION ( 'NONE',  ( 0.000000000000000000, 1.000000000000000000, 0.000000000000000000 ) ) ;
#41606=EDGE_LOOP ( 'NONE', ( #118169, #85260, #119661, #14728 ) ) ;
#41628=FACE_OUTER_BOUND ( 'NONE', #139788, .T. ) ;
#41664=MECHANICAL_DESIGN_GEOMETRIC_PRESENTATION_REPRESENTATION('',(#159145),#69287);
#41681=EDGE_CURVE ( 'NONE', #150870, #108531, #92958, .T. ) ;
#41687=CARTESIAN_POINT ( 'NONE',  ( -10.90688615205346856, -6.291672674598600246, 8.483881999699072196E-15 ) ) ;
#41702=CARTESIAN_POINT ( 'NONE',  ( 0.000000000000000000, 3.000000000000002665, 0.000000000000000000 ) ) ;
#41759=CARTESIAN_POINT ( 'NONE',  ( -10.64229060209977540, 1.016282880930358790, 6.144329343916601793 ) ) ;
#41832=CIRCLE ( 'NONE', #90360, 0.08000000000000020983 ) ;
#41837=VERTEX_POINT ( 'NONE', #50247 ) ;
#41848=CARTESIAN_POINT ( 'NONE',  ( 2.391594655221662258, 3.742896273583267597, -11.51132696612780748 ) ) ;
#41872=CARTESIAN_POINT ( 'NONE',  ( -10.91804383151480451, 0.000000000000000000, 0.1905751639681829146 ) ) ;
#41885=CARTESIAN_POINT ( 'NONE',  ( -3.459282556586562585E-15, 3.603753425775780617, 11.89624657422421627 ) ) ;
#41964=FACE_OUTER_BOUND ( 'NONE', #187378, .T. ) ;
#41987=UNCERTAINTY_MEASURE_WITH_UNIT (LENGTH_MEASURE( 1.000000000000000082E-05 ), #14906, 'distance_accuracy_value', 'NONE');
#41997=EDGE_CURVE ( 'NONE', #206526, #174410, #72182, .T. ) ;
#42020=CARTESIAN_POINT ( 'NONE',  ( -10.98194350564911659, -7.666862915010147717, 0.6300133639306291222 ) ) ;
#42034=CARTESIAN_POINT ( 'NONE',  ( -6.658747417465793461, -6.682123388833676181, -6.935047222998397487 ) ) ;
#42077=EDGE_CURVE ( 'NONE', #86477, #113056, #38260, .T. ) ;
#42087=CIRCLE ( 'NONE', #201123, 9.479622692290801567 ) ;
#42111=B_SPLINE_CURVE_WITH_KNOTS ( 'NONE', 3,
 ( #106912, #129589, #111188, #164144, #196637, #16788, #46142, #28807, #148949, #112256 ),
 .UNSPECIFIED., .F., .F.,
 ( 4, 2, 2, 2, 4 ),
 ( 0.000000000000000000, 0.0002299353307164190533, 0.0004598706614328381065, 0.0006898059921492572140, 0.0009197413228656762130 ),
 .UNSPECIFIED. ) ;
#42112=CARTESIAN_POINT ( 'NONE',  ( 0.000000000000000000, -13.99999999999999822, 0.000000000000000000 ) ) ;
#42127=AXIS2_PLACEMENT_3D ( 'NONE', #22930, #26151, #159358 ) ;
#42135=CARTESIAN_POINT ( 'NONE',  ( -0.04277205541327071259, -9.414847940711862151, -9.500256024741366545 ) ) ;
#42181=CARTESIAN_POINT ( 'NONE',  ( 0.000000000000000000, 0.000000000000000000, 9.579665964948883783 ) ) ;
#42192=ORIENTED_EDGE ( 'NONE', *, *, #47373, .F. ) ;
#42199=DIRECTION ( 'NONE',  ( 0.04267330865764933784, 4.780913106218958965E-15, 0.9990890794760041160 ) ) ;
#42200=CARTESIAN_POINT ( 'NONE',  ( -9.578206935409053102, -9.746166700193986898, 0.1671882239534360770 ) ) ;
#42225=ORIENTED_EDGE ( 'NONE', *, *, #22536, .T. ) ;
#42234=EDGE_CURVE ( 'NONE', #182554, #210172, #73727, .T. ) ;
#42237=ADVANCED_FACE ( 'NONE', ( #88077 ), #75029, .T. ) ;
#42268=UNCERTAINTY_MEASURE_WITH_UNIT (LENGTH_MEASURE( 1.000000000000000082E-05 ), #55053, 'distance_accuracy_value', 'NONE');
#42282=MECHANICAL_DESIGN_GEOMETRIC_PRESENTATION_REPRESENTATION('',(#156377),#153115);
#42315=CARTESIAN_POINT ( 'NONE',  ( 0.05503291520805564385, -6.406027784105803313, -11.00000000000011902 ) ) ;
#42319=FACE_OUTER_BOUND ( 'NONE', #55148, .T. ) ;
#42343=ORIENTED_EDGE ( 'NONE', *, *, #191143, .F. ) ;
#42349=CARTESIAN_POINT ( 'NONE',  ( -7.173763318588814109, -6.681223591462385869, 7.173763318588837201 ) ) ;
#42390=DIRECTION ( 'NONE',  ( 0.000000000000000000, 1.000000000000000000, 0.000000000000000000 ) ) ;
#42391=ORIENTED_EDGE ( 'NONE', *, *, #54338, .T. ) ;
#42410=CARTESIAN_POINT ( 'NONE',  ( 7.721398836998391246, 0.000000000000000000, 7.721398836998372595 ) ) ;
#42494=B_SPLINE_CURVE_WITH_KNOTS ( 'NONE', 3,
 ( #186169, #19402, #199207, #50854, #86552, #100664 ),
 .UNSPECIFIED., .F., .F.,
 ( 4, 2, 4 ),
 ( 0.000000000000000000, 0.001225895755212360596, 0.002451791510424720759 ),
 .UNSPECIFIED. ) ;
#42521=SURFACE_SIDE_STYLE ('',( #204968 ) ) ;
#42522=AXIS2_PLACEMENT_3D ( 'NONE', #31549, #213455, #65079 ) ;
#42526=CARTESIAN_POINT ( 'NONE',  ( 0.000000000000000000, 4.000000000000003553, 0.000000000000000000 ) ) ;
#42572=DIRECTION ( 'NONE',  ( 0.000000000000000000, 1.000000000000000000, 0.000000000000000000 ) ) ;
#42610=CARTESIAN_POINT ( 'NONE',  ( -0.1000000000000080685, -9.999999999999994671, -10.91954211494235238 ) ) ;
#42619=PRESENTATION_STYLE_ASSIGNMENT (( #176865 ) ) ;
#42637=AXIS2_PLACEMENT_3D ( 'NONE', #145810, #111207, #211817 ) ;
#42639=CYLINDRICAL_SURFACE ( 'NONE', #150746, 0.08000000000000020983 ) ;
#42680=CARTESIAN_POINT ( 'NONE',  ( 7.100579091572746471, -6.583980363594995389, -6.484567079770767961 ) ) ;
#42758=CARTESIAN_POINT ( 'NONE',  ( -10.99970480911017745, -6.304485801116145538, -0.08058605610350685899 ) ) ;
#42834=ORIENTED_EDGE ( 'NONE', *, *, #85714, .F. ) ;
#42863=CARTESIAN_POINT ( 'NONE',  ( 11.16489891154632907, 3.742896273583259159, -3.684481756086981363 ) ) ;
#42895=CARTESIAN_POINT ( 'NONE',  ( 0.4373225248172890045, -5.223431457505089526, 10.96785329849812385 ) ) ;
#42923=ORIENTED_EDGE ( 'NONE', *, *, #37862, .T. ) ;
#42938=CARTESIAN_POINT ( 'NONE',  ( -0.1969747848977146110, -6.717152734873772069, -10.87166355890665415 ) ) ;
#42950=VERTEX_POINT ( 'NONE', #14269 ) ;
#42951=LINE ( 'NONE', #30960, #190334 ) ;
#42952=CARTESIAN_POINT ( 'NONE',  ( -9.516228778038660963, -8.176227079964615285, 0.3870642018030935882 ) ) ;
#42999=EDGE_CURVE ( 'NONE', #100951, #212186, #86273, .T. ) ;
#43011=AXIS2_PLACEMENT_3D ( 'NONE', #139792, #120392, #203670 ) ;
#43052=ORIENTED_EDGE ( 'NONE', *, *, #63645, .T. ) ;
#43062=FACE_BOUND ( 'NONE', #146284, .T. ) ;
#43078=EDGE_CURVE ( 'NONE', #172976, #82895, #41310, .T. ) ;
#43093=B_SPLINE_CURVE_WITH_KNOTS ( 'NONE', 3,
 ( #105744, #167505, #104651, #168565, #87322, #36426, #118812, #136081 ),
 .UNSPECIFIED., .F., .F.,
 ( 4, 2, 2, 4 ),
 ( 1.069992374519254186E-15, 0.0004443203323512401174, 0.0006664804985263230895, 0.0008886406647014061157 ),
 .UNSPECIFIED. ) ;
#43100=CARTESIAN_POINT ( 'NONE',  ( -6.381095703207996905, -8.233137084989849086, -7.037870247915946287 ) ) ;
#43106=CARTESIAN_POINT ( 'NONE',  ( -10.93005900490891413, -6.124285369217943753, 1.138412281109779656E-15 ) ) ;
#43133=CARTESIAN_POINT ( 'NONE',  ( -9.617101990990361671, -9.241291349679078948, 0.3048231516917374040 ) ) ;
#43135=( BOUNDED_SURFACE ( )  B_SPLINE_SURFACE ( 3, 2, ( 
 ( #3207, #168936, #121340 ),
 ( #86621, #105026, #171064 ),
 ( #4271, #22661, #88772 ),
 ( #6414, #26937, #156972 ) ),
 .UNSPECIFIED., .F., .F., .T. ) 
 B_SPLINE_SURFACE_WITH_KNOTS ( ( 4, 4 ),
 ( 3, 3 ),
 ( 0.01133669335851671123, 0.01377857026255084258 ),
 ( 0.000000000000000000, 1.000000000000000000 ),
 .UNSPECIFIED. ) 
 GEOMETRIC_REPRESENTATION_ITEM ( )  RATIONAL_B_SPLINE_SURFACE ( (
 ( 1.000000000000000000, 0.7169883299103944063, 1.000000000000000000),
 ( 1.000000000000000000, 0.7174882367753923074, 1.000000000000000000),
 ( 1.000000000000000000, 0.7180609655871059704, 1.000000000000000000),
 ( 1.000000000000000000, 0.7187540731122940008, 1.000000000000000000) ) ) 
 REPRESENTATION_ITEM ( '' )  SURFACE ( )  );
#43154=CONICAL_SURFACE ( 'NONE', #47013, 6.249999999999995559, 0.7853981633974548293 ) ;
#43188=CARTESIAN_POINT ( 'NONE',  ( 7.712222144931855539, -6.293595771081261780, -7.712222144931889289 ) ) ;
#43202=CARTESIAN_POINT ( 'NONE',  ( 10.99126615174920651, -5.166862915010145052, -0.4382560683119322009 ) ) ;
#43203=CARTESIAN_POINT ( 'NONE',  ( 0.000000000000000000, 0.000000000000000000, 0.000000000000000000 ) ) ;
#43216=SURFACE_STYLE_USAGE ( .BOTH. , #29075 ) ;
#43242=DIRECTION ( 'NONE',  ( 0.000000000000000000, 0.000000000000000000, -1.000000000000000000 ) ) ;
#43284=CARTESIAN_POINT ( 'NONE',  ( -10.85353573482952072, -6.836568542495036205, 0.4635785636673775967 ) ) ;
#43307=CONICAL_SURFACE ( 'NONE', #164347, 6.249999999999995559, 0.7853981633974548293 ) ;
#43332=PLANE ( 'NONE',  #30120 ) ;
#43345=ORIENTED_EDGE ( 'NONE', *, *, #81818, .F. ) ;
#43358=CARTESIAN_POINT ( 'NONE',  ( -9.093502852636577316, 1.000000000000000888, -7.666967846417613863 ) ) ;
#43386=CARTESIAN_POINT ( 'NONE',  ( -0.3866937364864243554, 3.956598013261175772, 11.53692321988874170 ) ) ;
#43417=AXIS2_PLACEMENT_3D ( 'NONE', #73869, #176701, #26170 ) ;
#43447=CARTESIAN_POINT ( 'NONE',  ( 7.439168848973789494, -6.700000000000001954, 8.103009739378206788 ) ) ;
#43450=EDGE_LOOP ( 'NONE', ( #169588, #199582, #95288, #23578 ) ) ;
#43451=CARTESIAN_POINT ( 'NONE',  ( -5.204170427930421283E-15, -2.000000000000001776, -12.26547674076639716 ) ) ;
#43452=ORIENTED_EDGE ( 'NONE', *, *, #103866, .T. ) ;
#43457=ORIENTED_EDGE ( 'NONE', *, *, #117446, .F. ) ;
#43461=CARTESIAN_POINT ( 'NONE',  ( -10.99529341469513355, -7.794776013890357014, 0.3288329489800617123 ) ) ;
#43465=ADVANCED_FACE ( 'NONE', ( #16939, #79831 ), #30029, .T. ) ;
#43473=DIRECTION ( 'NONE',  ( -0.9980789807931677027, 0.06195440338564740107, 0.000000000000000000 ) ) ;
#43478=CARTESIAN_POINT ( 'NONE',  ( -9.500331257164621235, -7.246166700193446886, -1.011626589619743066E-12 ) ) ;
#43490=VERTEX_POINT ( 'NONE', #195728 ) ;
#43529=EDGE_CURVE ( 'NONE', #71781, #142721, #102111, .T. ) ;
#43535=DIRECTION ( 'NONE',  ( 0.000000000000000000, 1.000000000000000000, 0.000000000000000000 ) ) ;
#43574=EDGE_CURVE ( 'NONE', #14256, #18033, #34961, .T. ) ;
#43581=ADVANCED_FACE ( 'NONE', ( #128680 ), #79326, .T. ) ;
#43600=ORIENTED_EDGE ( 'NONE', *, *, #5319, .F. ) ;
#43617=DIRECTION ( 'NONE',  ( -0.9962287396576089415, 0.08676576675286083729, 0.000000000000000000 ) ) ;
#43654=FILL_AREA_STYLE_COLOUR ( '', #73011 ) ;
#43674=CARTESIAN_POINT ( 'NONE',  ( -0.009341426467593692828, -9.943661027227911120, -10.91969313363969007 ) ) ;
#43682=CARTESIAN_POINT ( 'NONE',  ( 7.552496594302675170, -5.254973434576991842, 7.962224162659105708 ) ) ;
#43701=CARTESIAN_POINT ( 'NONE',  ( -6.713552092916992287, -7.189371949512880278, -6.722000117220233051 ) ) ;
#43744=CARTESIAN_POINT ( 'NONE',  ( 7.015831072854086692, -6.604036961759984337, -6.576431128233156009 ) ) ;
#43748=DIRECTION ( 'NONE',  ( 0.000000000000000000, 0.000000000000000000, 1.000000000000000000 ) ) ;
#43762=VECTOR ( 'NONE', #160000, 1000.000000000000000 ) ;
#43766=CARTESIAN_POINT ( 'NONE',  ( 6.956180625286545904, -6.372104534814153176, -6.956180625285512065 ) ) ;
#43773=CARTESIAN_POINT ( 'NONE',  ( 0.09411116651286953461, -9.919020924439822195, 10.99959762541857877 ) ) ;
#43782=AXIS2_PLACEMENT_3D ( 'NONE', #138653, #55258, #24871 ) ;
#43801=LINE ( 'NONE', #173802, #99959 ) ;
#43834=FACE_OUTER_BOUND ( 'NONE', #120025, .T. ) ;
#43843=AXIS2_PLACEMENT_3D ( 'NONE', #129296, #195271, #146549 ) ;
#43858=SURFACE_STYLE_USAGE ( .BOTH. , #190072 ) ;
#43873=CARTESIAN_POINT ( 'NONE',  ( -0.08172171391244466288, -9.906619969460795261, -10.99969643042365419 ) ) ;
#43946=CARTESIAN_POINT ( 'NONE',  ( 0.008494835128459769791, -5.601932402265091149, 11.00038526257045390 ) ) ;
#43963=ORIENTED_EDGE ( 'NONE', *, *, #23354, .F. ) ;
#43965=ORIENTED_EDGE ( 'NONE', *, *, #3532, .F. ) ;
#43966=EDGE_CURVE ( 'NONE', #9078, #24478, #204434, .T. ) ;
#44004=CARTESIAN_POINT ( 'NONE',  ( 9.617648866954018771, -9.063431457505044975, -0.6035590660249217088 ) ) ;
#44036=CARTESIAN_POINT ( 'NONE',  ( 10.67552548858665418, -7.034525073436789455, 9.912773128239630417E-13 ) ) ;
#44043=ORIENTED_EDGE ( 'NONE', *, *, #188975, .F. ) ;
#44068=CARTESIAN_POINT ( 'NONE',  ( 0.000000000000000000, -9.900000000000005684, 10.91970695577495931 ) ) ;
#44093=CARTESIAN_POINT ( 'NONE',  ( -0.07538891330675576152, -7.154544010627095219, 9.499700864329900796 ) ) ;
#44159=ORIENTED_EDGE ( 'NONE', *, *, #189732, .F. ) ;
#44187=CARTESIAN_POINT ( 'NONE',  ( -9.497898427948538114, -9.431315562283163700, 0.2398643602166746491 ) ) ;
#44212=AXIS2_PLACEMENT_3D ( 'NONE', #61780, #176600, #10871 ) ;
#44228=FILL_AREA_STYLE ('',( #192573 ) ) ;
#44242=CARTESIAN_POINT ( 'NONE',  ( 7.834474503270790535, -6.459788825448837812, -7.722692672890167032 ) ) ;
#44250=ADVANCED_FACE ( 'NONE', ( #91330 ), #34676, .F. ) ;
#44255=CARTESIAN_POINT ( 'NONE',  ( 0.000000000000000000, 0.000000000000000000, 0.000000000000000000 ) ) ;
#44269=SURFACE_STYLE_FILL_AREA ( #191549 ) ;
#44272=EDGE_CURVE ( 'NONE', #97798, #105253, #39965, .T. ) ;
#44324=DIRECTION ( 'NONE',  ( 0.000000000000000000, 1.000000000000000000, 0.000000000000000000 ) ) ;
#44338=EDGE_CURVE ( 'NONE', #18903, #80718, #28440, .T. ) ;
#44367=CARTESIAN_POINT ( 'NONE',  ( -0.008494835128554827433, -5.601932402265138222, -11.00038526257045390 ) ) ;
#44380=SURFACE_SIDE_STYLE ('',( #192726 ) ) ;
#44388=FACE_OUTER_BOUND ( 'NONE', #193933, .T. ) ;
#44392=ORIENTED_EDGE ( 'NONE', *, *, #38423, .F. ) ;
#44433=CARTESIAN_POINT ( 'NONE',  ( -0.3046331935817688241, -6.606549254264993287, -9.611339018008544954 ) ) ;
#44456=DIRECTION ( 'NONE',  ( 0.000000000000000000, 0.000000000000000000, 1.000000000000000000 ) ) ;
#44472=ORIENTED_EDGE ( 'NONE', *, *, #76253, .T. ) ;
#44482=ORIENTED_EDGE ( 'NONE', *, *, #67908, .F. ) ;
#44489=CARTESIAN_POINT ( 'NONE',  ( 0.000000000000000000, 0.000000000000000000, 0.000000000000000000 ) ) ;
#44508=ORIENTED_EDGE ( 'NONE', *, *, #118916, .F. ) ;
#44512=CARTESIAN_POINT ( 'NONE',  ( 7.470306724221089212, -6.701288531903148993, 8.074422843255659288 ) ) ;
#44513=CARTESIAN_POINT ( 'NONE',  ( 0.000000000000000000, -9.746166700180788567, 9.579665964948883783 ) ) ;
#44516=DIRECTION ( 'NONE',  ( -1.776356839400250465E-15, 0.000000000000000000, 1.000000000000000000 ) ) ;
#44530=DIRECTION ( 'NONE',  ( 0.000000000000000000, 1.000000000000000000, 0.000000000000000000 ) ) ;
#44573=AXIS2_PLACEMENT_3D ( 'NONE', #140911, #8729, #156061 ) ;
#44619=CARTESIAN_POINT ( 'NONE',  ( 6.451695228974854146, -8.176248043968833201, 7.005920419302530178 ) ) ;
#44666=VERTEX_POINT ( 'NONE', #36959 ) ;
#44667=ORIENTED_EDGE ( 'NONE', *, *, #34950, .T. ) ;
#44682=EDGE_CURVE ( 'NONE', #83007, #34393, #29608, .T. ) ;
#44712=CARTESIAN_POINT ( 'NONE',  ( 10.96384816988413924, 2.972657967447023708, -3.969100948793135686 ) ) ;
#44741=CYLINDRICAL_SURFACE ( 'NONE', #37492, 8.049999999999993605 ) ;
#44752=CARTESIAN_POINT ( 'NONE',  ( 10.10343170205820407, 2.974000657017351390, 5.833219012922953972 ) ) ;
#44861=DIRECTION ( 'NONE',  ( 0.000000000000000000, 0.000000000000000000, 1.000000000000000000 ) ) ;
#44881=AXIS2_PLACEMENT_3D ( 'NONE', #134829, #36218, #114367 ) ;
#44939=EDGE_CURVE ( 'NONE', #192862, #74902, #86366, .T. ) ;
#44968=ORIENTED_EDGE ( 'NONE', *, *, #26377, .F. ) ;
#45042=CARTESIAN_POINT ( 'NONE',  ( 0.3869736770896747835, 1.794419290072776896, -11.79366332131311523 ) ) ;
#45047=EDGE_CURVE ( 'NONE', #148930, #60029, #132816, .T. ) ;
#45056=VERTEX_POINT ( 'NONE', #210108 ) ;
#45071=CARTESIAN_POINT ( 'NONE',  ( -0.4694063952341876456, -6.700000000000002842, -10.98997987423603107 ) ) ;
#45106=VERTEX_POINT ( 'NONE', #176569 ) ;
#45114=CARTESIAN_POINT ( 'NONE',  ( -10.30923643716948490, 0.9706168436483916251, -5.952040432139263260 ) ) ;
#45142=ORIENTED_EDGE ( 'NONE', *, *, #5562, .T. ) ;
#45219=CARTESIAN_POINT ( 'NONE',  ( 7.767011945534265216, -7.169578370797519362, -7.110792111438882124 ) ) ;
#45230=CARTESIAN_POINT ( 'NONE',  ( -6.484567079770452658, -6.583980363594976737, -7.100579091573040458 ) ) ;
#45284=EDGE_CURVE ( 'NONE', #100589, #144319, #135687, .T. ) ;
#45304=ORIENTED_EDGE ( 'NONE', *, *, #116636, .T. ) ;
#45316=FACE_OUTER_BOUND ( 'NONE', #104982, .T. ) ;
#45319=CIRCLE ( 'NONE', #152609, 0.08000000000000050127 ) ;
#45420=VERTEX_POINT ( 'NONE', #118422 ) ;
#45424=CARTESIAN_POINT ( 'NONE',  ( 7.765925996254661179, -5.615420858948578342, -7.710915694720370084 ) ) ;
#45438=ORIENTED_EDGE ( 'NONE', *, *, #163321, .T. ) ;
#45450=CARTESIAN_POINT ( 'NONE',  ( -1.409462824231155764E-15, 1.016282880930355459, 12.28865868783309701 ) ) ;
#45516=CARTESIAN_POINT ( 'NONE',  ( 0.000000000000000000, -6.532648833121171172, 0.000000000000000000 ) ) ;
#45525=CARTESIAN_POINT ( 'NONE',  ( -0.07302493934789386354, 1.405922845961228962, 11.99988463978226250 ) ) ;
#45532=AXIS2_PLACEMENT_3D ( 'NONE', #37031, #200583, #169174 ) ;
#45555=DIRECTION ( 'NONE',  ( 0.04529798058948776573, 0.000000000000000000, 0.9989735196462988798 ) ) ;
#45577=CARTESIAN_POINT ( 'NONE',  ( 7.455003611050232237, -6.808400134080644150, 7.905503641038496454 ) ) ;
#45587=VERTEX_POINT ( 'NONE', #34453 ) ;
#45592=ORIENTED_EDGE ( 'NONE', *, *, #136104, .T. ) ;
#45627=CARTESIAN_POINT ( 'NONE',  ( 11.00039779440667154, -6.304807775344823284, -0.01400375819716699437 ) ) ;
#45640=EDGE_CURVE ( 'NONE', #15455, #172181, #65613, .T. ) ;
#45653=CARTESIAN_POINT ( 'NONE',  ( 0.000000000000000000, -5.199999999999996625, 0.000000000000000000 ) ) ;
#45686=VERTEX_POINT ( 'NONE', #53917 ) ;
#45687=DIRECTION ( 'NONE',  ( 0.000000000000000000, 1.000000000000000000, 0.000000000000000000 ) ) ;
#45755=ORIENTED_EDGE ( 'NONE', *, *, #101405, .F. ) ;
#45780=B_SPLINE_CURVE_WITH_KNOTS ( 'NONE', 3,
 ( #214398, #150533, #198183, #3163, #68168, #134300, #120223, #200307, #181931, #66027, #184067, #118081, #35687, #185125, #101763, #36750 ),
 .UNSPECIFIED., .F., .F.,
 ( 4, 3, 3, 3, 3, 4 ),
 ( 0.000000000000000000, 4.381999914579121551E-06, 1.110488615493335718E-05, 1.784390311306779410E-05, 2.460054645147216775E-05, 3.136851507421684792E-05 ),
 .UNSPECIFIED. ) ;
#45810=ORIENTED_EDGE ( 'NONE', *, *, #201793, .T. ) ;
#45816=CARTESIAN_POINT ( 'NONE',  ( 7.501945787865619941, -5.223163706540480788, 8.013579835756337033 ) ) ;
#45834=CARTESIAN_POINT ( 'NONE',  ( -6.776370306708066060, -7.161464053357566861, -6.781144757626042185 ) ) ;
#45888=DIRECTION ( 'NONE',  ( 0.000000000000000000, -1.000000000000000000, 0.000000000000000000 ) ) ;
#45894=CARTESIAN_POINT ( 'NONE',  ( 8.072398248062480519, -5.212532583863434432, -7.453913518772576019 ) ) ;
#45963=( NAMED_UNIT ( * ) PLANE_ANGLE_UNIT ( ) SI_UNIT ( $, .RADIAN. ) );
#45976=EDGE_LOOP ( 'NONE', ( #134278, #10291, #26384, #153107 ) ) ;
#45989=CARTESIAN_POINT ( 'NONE',  ( 10.91944002402979130, -8.407420853759269619, -0.1105873483556608222 ) ) ;
#46022=ORIENTED_EDGE ( 'NONE', *, *, #173466, .T. ) ;
#46101=EDGE_LOOP ( 'NONE', ( #28500, #204462, #196158, #179455 ) ) ;
#46120=ORIENTED_EDGE ( 'NONE', *, *, #185379, .F. ) ;
#46124=ORIENTED_EDGE ( 'NONE', *, *, #45047, .T. ) ;
#46141=AXIS2_PLACEMENT_3D ( 'NONE', #9860, #211250, #158271 ) ;
#46142=CARTESIAN_POINT ( 'NONE',  ( 0.1888596022590748325, -6.708723052947950904, 10.87247189006428272 ) ) ;
#46178=CARTESIAN_POINT ( 'NONE',  ( -7.727873494160017565, -5.742104877864247392, 7.828177403543863377 ) ) ;
#46183=CARTESIAN_POINT ( 'NONE',  ( -3.469446951953614189E-15, 3.487142912321096855, 11.99525683304595702 ) ) ;
#46191=ORIENTED_EDGE ( 'NONE', *, *, #135617, .F. ) ;
#46199=VECTOR ( 'NONE', #121503, 1000.000000000000000 ) ;
#46207=CARTESIAN_POINT ( 'NONE',  ( 6.434831245971852631, -8.233137084989849086, 7.097136523687869847 ) ) ;
#46209=AXIS2_PLACEMENT_3D ( 'NONE', #131267, #148526, #146417 ) ;
#46210=DIRECTION ( 'NONE',  ( 0.000000000000000000, 0.000000000000000000, 1.000000000000000000 ) ) ;
#46250=CARTESIAN_POINT ( 'NONE',  ( 11.18654035131437219, 1.000000000000000888, -4.041720556560823852 ) ) ;
#46252=DIRECTION ( 'NONE',  ( 0.000000000000000000, 0.000000000000000000, 1.000000000000000000 ) ) ;
#46263=ORIENTED_EDGE ( 'NONE', *, *, #33969, .T. ) ;
#46272=( BOUNDED_SURFACE ( )  B_SPLINE_SURFACE ( 3, 2, ( 
 ( #168335, #19929, #86016 ),
 ( #7166, #105800, #21271 ),
 ( #190196, #71092, #188060 ),
 ( #169683, #138272, #206446 ) ),
 .UNSPECIFIED., .F., .F., .T. ) 
 B_SPLINE_SURFACE_WITH_KNOTS ( ( 4, 4 ),
 ( 3, 3 ),
 ( 0.004991389062828482590, 0.008017777006561210146 ),
 ( 0.000000000000000000, 1.000000000000000000 ),
 .UNSPECIFIED. ) 
 GEOMETRIC_REPRESENTATION_ITEM ( )  RATIONAL_B_SPLINE_SURFACE ( (
 ( 1.000000000000000000, 0.7184380228464066764, 1.000000000000000000),
 ( 1.000000000000000000, 0.7185467277397524777, 1.000000000000000000),
 ( 1.000000000000000000, 0.7186585579881034080, 1.000000000000000000),
 ( 1.000000000000000000, 0.7187737999613694750, 1.000000000000000000) ) ) 
 REPRESENTATION_ITEM ( '' )  SURFACE ( )  );
#46303=DIRECTION ( 'NONE',  ( 0.000000000000000000, 0.000000000000000000, 1.000000000000000000 ) ) ;
#46377=CARTESIAN_POINT ( 'NONE',  ( 9.500479199177245704, -7.792108994756139495, -0.01138762994422098072 ) ) ;
#46381=FILL_AREA_STYLE ('',( #112499 ) ) ;
#46421=CARTESIAN_POINT ( 'NONE',  ( 0.1360919303235845756, -7.795524846228436999, -10.99936842639231571 ) ) ;
#46472=CARTESIAN_POINT ( 'NONE',  ( 0.4635785636673654952, -6.836568542495036205, 10.85353573482952250 ) ) ;
#46501=VECTOR ( 'NONE', #140994, 1000.000000000000000 ) ;
#46509=EDGE_CURVE ( 'NONE', #190376, #146171, #58158, .T. ) ;
#46528=CARTESIAN_POINT ( 'NONE',  ( -0.03919461954072858689, -7.818966704647663413, 9.500338091956020747 ) ) ;
#46637=CARTESIAN_POINT ( 'NONE',  ( 7.401194801146942837, -6.836289462023670715, 7.952857047016752112 ) ) ;
#46640=ORIENTED_EDGE ( 'NONE', *, *, #165017, .F. ) ;
#46654=ORIENTED_EDGE ( 'NONE', *, *, #14059, .F. ) ;
#46701=AXIS2_PLACEMENT_3D ( 'NONE', #13813, #113534, #114598 ) ;
#46711=EDGE_CURVE ( 'NONE', #118245, #53554, #205282, .T. ) ;
#46721=CARTESIAN_POINT ( 'NONE',  ( -7.583532603600728450, -5.197284395437328897, -7.968353659517138254 ) ) ;
#46724=ORIENTED_EDGE ( 'NONE', *, *, #166817, .T. ) ;
#46726=CARTESIAN_POINT ( 'NONE',  ( 0.07933194154487849259, -9.746166700180788567, 9.499668754385625746 ) ) ;
#46748=( BOUNDED_SURFACE ( )  B_SPLINE_SURFACE ( 3, 2, ( 
 ( #100173, #150002, #67633 ),
 ( #82851, #51433, #198715 ),
 ( #183547, #2639, #54622 ),
 ( #152131, #52488, #165173 ),
 ( #1572, #69776, #166238 ),
 ( #66568, #169438, #117553 ),
 ( #50361, #167313, #18900 ),
 ( #17828, #21022, #135884 ) ),
 .UNSPECIFIED., .F., .F., .T. ) 
 B_SPLINE_SURFACE_WITH_KNOTS ( ( 4, 2, 2, 4 ),
 ( 3, 3 ),
 ( 0.000000000000000000, 0.0002204160392919248825, 0.0004408320785838497650, 0.0008816641571676995300 ),
 ( 0.000000000000000000, 1.000000000000000000 ),
 .UNSPECIFIED. ) 
 GEOMETRIC_REPRESENTATION_ITEM ( )  RATIONAL_B_SPLINE_SURFACE ( (
 ( 1.000000000000000000, 0.4127341956165090364, 1.000000000000000000),
 ( 1.000000000000000000, 0.4103180386329450813, 1.000000000000000000),
 ( 1.000000000000000000, 0.4223234233960728723, 1.000000000000000000),
 ( 1.000000000000000000, 0.4613847219396438604, 1.000000000000000000),
 ( 1.000000000000000000, 0.4878744032655865093, 1.000000000000000000),
 ( 1.000000000000000000, 0.5702658980234648345, 1.000000000000000000),
 ( 1.000000000000000000, 0.6280001242509933856, 1.000000000000000000),
 ( 1.000000000000000000, 0.6787756258918243857, 1.000000000000000000) ) ) 
 REPRESENTATION_ITEM ( '' )  SURFACE ( )  );
#46755=CYLINDRICAL_SURFACE ( 'NONE', #205408, 0.08000000000000020983 ) ;
#46789=FACE_OUTER_BOUND ( 'NONE', #41606, .T. ) ;
#46843=CARTESIAN_POINT ( 'NONE',  ( 6.534012848836709075, -6.583711766989043035, 7.055786748303249922 ) ) ;
#46849=CARTESIAN_POINT ( 'NONE',  ( -6.726765609221550868, -8.198316280115697907, 6.726765609221573960 ) ) ;
#46868=ORIENTED_EDGE ( 'NONE', *, *, #119448, .T. ) ;
#46876=VECTOR ( 'NONE', #59422, 1000.000000000000000 ) ;
#46905=CYLINDRICAL_SURFACE ( 'NONE', #26250, 0.08000000000000020983 ) ;
#46908=ORIENTED_EDGE ( 'NONE', *, *, #80448, .F. ) ;
#46911=CARTESIAN_POINT ( 'NONE',  ( 6.775478006741562531, -7.217909409563599610, -6.775478006741584736 ) ) ;
#46921=FACE_OUTER_BOUND ( 'NONE', #72671, .T. ) ;
#46974=CARTESIAN_POINT ( 'NONE',  ( -0.08000000000000367928, -7.246166700194011767, 9.579665964948883783 ) ) ;
#46993=CARTESIAN_POINT ( 'NONE',  ( 0.000000000000000000, -11.15905291171102931, 0.000000000000000000 ) ) ;
#47013=AXIS2_PLACEMENT_3D ( 'NONE', #143677, #127474, #209670 ) ;
#47043=ORIENTED_EDGE ( 'NONE', *, *, #42234, .T. ) ;
#47087=ORIENTED_EDGE ( 'NONE', *, *, #151210, .T. ) ;
#47094=CIRCLE ( 'NONE', #150981, 0.08000000000000020983 ) ;
#47095=B_SPLINE_CURVE_WITH_KNOTS ( 'NONE', 3,
 ( #179300, #30921, #147862, #96997, #146814, #196602, #48243, #114356 ),
 .UNSPECIFIED., .F., .F.,
 ( 4, 2, 2, 4 ),
 ( 0.000000000000000000, 0.0003954713701971457199, 0.0005932070552957175499, 0.0007909427403942893798 ),
 .UNSPECIFIED. ) ;
#47100=SURFACE_SIDE_STYLE ('',( #29770 ) ) ;
#47107=CARTESIAN_POINT ( 'NONE',  ( 10.91944002402978775, -9.999999999999994671, -0.1105873483556677611 ) ) ;
#47123=AXIS2_PLACEMENT_3D ( 'NONE', #45989, #61146, #15571 ) ;
#47177=CARTESIAN_POINT ( 'NONE',  ( 0.3868823266961737839, 2.515145635913770494, -11.70808416779823524 ) ) ;
#47189=CARTESIAN_POINT ( 'NONE',  ( 0.07933194154487524519, -7.246166700194011767, -9.499668754385622194 ) ) ;
#47197=DIRECTION ( 'NONE',  ( 0.000000000000000000, 1.000000000000000000, 0.000000000000000000 ) ) ;
#47246=CARTESIAN_POINT ( 'NONE',  ( -10.00050683067327384, 3.975933801733735784, -5.773795310721868468 ) ) ;
#47250=CARTESIAN_POINT ( 'NONE',  ( -7.777446446097295407, -5.502990254781792601, 7.779015489124650351 ) ) ;
#47280=DIRECTION ( 'NONE',  ( -0.6716942845482061220, 0.000000000000000000, -0.7408284471490504952 ) ) ;
#47283=CARTESIAN_POINT ( 'NONE',  ( -6.801849727212544217, -7.605490242344541407, -7.458876343101966455 ) ) ;
#47307=FACE_OUTER_BOUND ( 'NONE', #43450, .T. ) ;
#47325=PRESENTATION_STYLE_ASSIGNMENT (( #196749 ) ) ;
#47332=FACE_OUTER_BOUND ( 'NONE', #191007, .T. ) ;
#47339=DIRECTION ( 'NONE',  ( 0.000000000000000000, -3.252606517456504467E-14, -1.000000000000000000 ) ) ;
#47354=CARTESIAN_POINT ( 'NONE',  ( 7.055228938194279209, -8.176568542494891290, -6.396834479292358822 ) ) ;
#47364=CARTESIAN_POINT ( 'NONE',  ( 8.855744143575730476, 3.691791674785632082, 7.453352967675146878 ) ) ;
#47373=EDGE_CURVE ( 'NONE', #146105, #210172, #163036, .T. ) ;
#47386=CARTESIAN_POINT ( 'NONE',  ( -10.10176665042269839, 1.000000000000000888, -6.279211784079198999 ) ) ;
#47447=EDGE_LOOP ( 'NONE', ( #103654, #66947, #27231, #5380, #54859 ) ) ;
#47485=ORIENTED_EDGE ( 'NONE', *, *, #79889, .F. ) ;
#47548=UNCERTAINTY_MEASURE_WITH_UNIT (LENGTH_MEASURE( 1.000000000000000082E-05 ), #4115, 'distance_accuracy_value', 'NONE');
#47601=DIRECTION ( 'NONE',  ( -0.009157509157509154465, 0.000000000000000000, -0.9999580691339163829 ) ) ;
#47639=AXIS2_PLACEMENT_3D ( 'NONE', #210041, #75798, #80057 ) ;
#47715=CARTESIAN_POINT ( 'NONE',  ( 6.661184053807540195, -7.645781813054109755, -6.773376336901701045 ) ) ;
#47790=ORIENTED_EDGE ( 'NONE', *, *, #90996, .T. ) ;
#47827=CARTESIAN_POINT ( 'NONE',  ( -9.579253414572390213, -9.994362535427860905, 0.1002978391578569772 ) ) ;
#47842=ORIENTED_EDGE ( 'NONE', *, *, #73745, .F. ) ;
#47854=CARTESIAN_POINT ( 'NONE',  ( 6.717278222822382183, -7.473374494058216300, -6.830415307812249814 ) ) ;
#47864=CARTESIAN_POINT ( 'NONE',  ( -6.446420058208179427, -6.527411821100059797, -7.058808231563611812 ) ) ;
#47901=AXIS2_PLACEMENT_3D ( 'NONE', #207208, #126047, #139036 ) ;
#47922=CARTESIAN_POINT ( 'NONE',  ( -0.04536292375657846598, -10.00000000000003908, -10.91964218157423083 ) ) ;
#47934=LINE ( 'NONE', #84659, #83837 ) ;
#47949=( NAMED_UNIT ( * ) SI_UNIT ( $, .STERADIAN. ) SOLID_ANGLE_UNIT ( ) );
#47981=ORIENTED_EDGE ( 'NONE', *, *, #69925, .F. ) ;
#47985=EDGE_LOOP ( 'NONE', ( #116901, #64046, #50117, #65842 ) ) ;
#48016=CARTESIAN_POINT ( 'NONE',  ( -0.07933194018405020920, -7.215568602689852007, 9.499668754397001535 ) ) ;
#48038=CARTESIAN_POINT ( 'NONE',  ( 7.257245574617835260, -6.363025497629767990, -6.640718169119574910 ) ) ;
#48051=PLANE ( 'NONE',  #188096 ) ;
#48065=CARTESIAN_POINT ( 'NONE',  ( -10.85277107007939001, 3.956598013261175772, 3.932872935640539414 ) ) ;
#48138=AXIS2_PLACEMENT_3D ( 'NONE', #119440, #185427, #37046 ) ;
#48143=ADVANCED_FACE ( 'NONE', ( #195289, #46921 ), #114111, .T. ) ;
#48156=DIRECTION ( 'NONE',  ( -0.7071067811865489050, 0.000000000000000000, -0.7071067811865462405 ) ) ;
#48204=ADVANCED_FACE ( 'NONE', ( #152927 ), #144181, .T. ) ;
#48243=CARTESIAN_POINT ( 'NONE',  ( 9.609441814500813805, -6.583711573986998467, -0.3689019803512830764 ) ) ;
#48281=DIRECTION ( 'NONE',  ( -0.9990890794760040050, 5.454924750823445190E-15, 0.04267330865764876885 ) ) ;
#48296=EDGE_CURVE ( 'NONE', #194999, #68165, #66195, .T. ) ;
#48324=CARTESIAN_POINT ( 'NONE',  ( 6.717748655459607754, -7.246166700180828535, -6.717748655459624629 ) ) ;
#48325=EDGE_CURVE ( 'NONE', #197280, #148930, #187280, .T. ) ;
#48326=EDGE_LOOP ( 'NONE', ( #190846, #144179, #91428, #94946 ) ) ;
#48342=DIRECTION ( 'NONE',  ( -0.9510565162951500895, 0.000000000000000000, 0.3090169943749582759 ) ) ;
#48390=( LENGTH_UNIT ( ) NAMED_UNIT ( * ) SI_UNIT ( .MILLI., .METRE. ) );
#48392=AXIS2_PLACEMENT_3D ( 'NONE', #41702, #155423, #58992 ) ;
#48399=B_SPLINE_CURVE_WITH_KNOTS ( 'NONE', 3,
 ( #77257, #94607, #92479, #207253, #158520, #125036, #127172 ),
 .UNSPECIFIED., .F., .F.,
 ( 4, 3, 4 ),
 ( 0.000000000000000000, 0.0008000000000004422844, 0.002977368225425623249 ),
 .UNSPECIFIED. ) ;
#48407=ORIENTED_EDGE ( 'NONE', *, *, #102049, .F. ) ;
#48467=LINE ( 'NONE', #98271, #203056 ) ;
#48489=DIRECTION ( 'NONE',  ( 0.000000000000000000, 0.000000000000000000, 1.000000000000000000 ) ) ;
#48500=ORIENTED_EDGE ( 'NONE', *, *, #72198, .F. ) ;
#48528=CARTESIAN_POINT ( 'NONE',  ( 6.776370306708059843, -7.161464053357565973, 6.781144757626057284 ) ) ;
#48530=CARTESIAN_POINT ( 'NONE',  ( -2.173285075505815599E-15, -8.011313137147263674, 11.00000000000000178 ) ) ;
#48533=CARTESIAN_POINT ( 'NONE',  ( 10.40709887848268167, 1.794419290072776896, -5.561702625701125946 ) ) ;
#48561=CARTESIAN_POINT ( 'NONE',  ( 9.578446392664460518, -9.953004327042588528, -0.1519871474491476526 ) ) ;
#48571=TOROIDAL_SURFACE ( 'NONE', #34790, 10.92000000000000171, 0.08000000000000000167 ) ;
#48616=EDGE_LOOP ( 'NONE', ( #3313, #189788, #13039, #74092 ) ) ;
#48621=FACE_OUTER_BOUND ( 'NONE', #52117, .T. ) ;
#48631=CARTESIAN_POINT ( 'NONE',  ( -7.720982897393583677, -9.999999999999994671, 7.834948825496934610 ) ) ;
#48643=CARTESIAN_POINT ( 'NONE',  ( -0.4644097342743139234, -8.233137084989849086, -9.488641820551089623 ) ) ;
#48732=DIRECTION ( 'NONE',  ( 0.000000000000000000, 1.000000000000000000, 0.000000000000000000 ) ) ;
#48764=CARTESIAN_POINT ( 'NONE',  ( 0.09263630470259102967, -10.00000000000047251, 9.579493439010624556 ) ) ;
#48765=CARTESIAN_POINT ( 'NONE',  ( -0.3602790413719305640, -9.063128419003716019, 9.630430012830167641 ) ) ;
#48800=( BOUNDED_SURFACE ( )  B_SPLINE_SURFACE ( 3, 2, ( 
 ( #186430, #168066, #85743 ),
 ( #5521, #87880, #151827 ),
 ( #23926, #38069, #153953 ),
 ( #71601, #152878, #137710 ),
 ( #203732, #122609, #121533 ),
 ( #187503, #19666, #135575 ),
 ( #105215, #171253, #6602 ),
 ( #72683, #52183, #138778 ) ),
 .UNSPECIFIED., .F., .F., .T. ) 
 B_SPLINE_SURFACE_WITH_KNOTS ( ( 4, 2, 2, 4 ),
 ( 3, 3 ),
 ( 0.000000000000000000, 0.0002568729646053923097, 0.0005137459292107846194, 0.001027491858421569239 ),
 ( 0.000000000000000000, 1.000000000000000000 ),
 .UNSPECIFIED. ) 
 GEOMETRIC_REPRESENTATION_ITEM ( )  RATIONAL_B_SPLINE_SURFACE ( (
 ( 1.000000000000000000, 0.3826834323651035485, 1.000000000000000000),
 ( 1.000000000000000000, 0.3847114443836440745, 1.000000000000000000),
 ( 1.000000000000000000, 0.4039255759072567509, 1.000000000000000000),
 ( 1.000000000000000000, 0.4557194474498202919, 1.000000000000000000),
 ( 1.000000000000000000, 0.4874388927522833037, 1.000000000000000000),
 ( 1.000000000000000000, 0.5833547384518390500, 1.000000000000000000),
 ( 1.000000000000000000, 0.6470545345835431172, 1.000000000000000000),
 ( 1.000000000000000000, 0.7045118851637689472, 1.000000000000000000) ) ) 
 REPRESENTATION_ITEM ( '' )  SURFACE ( )  );
#48815=EDGE_CURVE ( 'NONE', #145242, #67222, #202157, .T. ) ;
#48816=CARTESIAN_POINT ( 'NONE',  ( 10.86152993230179220, -6.808378554901793223, -0.3183146091066044736 ) ) ;
#48830=EDGE_CURVE ( 'NONE', #191645, #138616, #21354, .T. ) ;
#48905=DIRECTION ( 'NONE',  ( 0.000000000000000000, 0.000000000000000000, 1.000000000000000000 ) ) ;
#48919=ORIENTED_EDGE ( 'NONE', *, *, #190705, .F. ) ;
#48920=ORIENTED_EDGE ( 'NONE', *, *, #212049, .T. ) ;
#48927=ORIENTED_EDGE ( 'NONE', *, *, #43966, .F. ) ;
#48931=AXIS2_PLACEMENT_3D ( 'NONE', #88179, #36207, #185657 ) ;
#48961=ORIENTED_EDGE ( 'NONE', *, *, #102136, .T. ) ;
#48966=CARTESIAN_POINT ( 'NONE',  ( 9.490381562237910629, -9.037089468803353398, -0.4325416218483115194 ) ) ;
#48970=CARTESIAN_POINT ( 'NONE',  ( -7.458876248283173638, -7.605490376493679427, 6.801849632071883534 ) ) ;
#49034=CARTESIAN_POINT ( 'NONE',  ( 6.937452841262695458, -7.242250812743807664, -6.937452841262718550 ) ) ;
#49037=CARTESIAN_POINT ( 'NONE',  ( 7.755938900619410603, -5.581885079358431589, -7.800371912476627756 ) ) ;
#49064=CARTESIAN_POINT ( 'NONE',  ( -0.07933194154488883154, -7.246166700194011767, 9.499668754385636404 ) ) ;
#49077=DIRECTION ( 'NONE',  ( 0.000000000000000000, 1.000000000000000000, 0.000000000000000000 ) ) ;
#49165=ORIENTED_EDGE ( 'NONE', *, *, #147708, .T. ) ;
#49210=ORIENTED_EDGE ( 'NONE', *, *, #50663, .T. ) ;
#49226=CARTESIAN_POINT ( 'NONE',  ( -6.770610912236888268, -7.154544010627095219, -6.663994888585867749 ) ) ;
#49230=AXIS2_PLACEMENT_3D ( 'NONE', #165850, #194072, #64090 ) ;
#49261=CARTESIAN_POINT ( 'NONE',  ( -10.99126615174920651, -5.199999999999992184, 0.4382560683119312572 ) ) ;
#49265=SURFACE_STYLE_USAGE ( .BOTH. , #66527 ) ;
#49289=ORIENTED_EDGE ( 'NONE', *, *, #7969, .F. ) ;
#49311=ORIENTED_EDGE ( 'NONE', *, *, #20338, .F. ) ;
#49326=CARTESIAN_POINT ( 'NONE',  ( -0.4360851681528791768, -8.730413173480725320, 9.960047168614407198 ) ) ;
#49351=ORIENTED_EDGE ( 'NONE', *, *, #67862, .T. ) ;
#49379=CARTESIAN_POINT ( 'NONE',  ( 0.09540182900466742666, -7.837949925775435922, -10.99983588129881618 ) ) ;
#49388=EDGE_CURVE ( 'NONE', #1801, #96623, #85964, .T. ) ;
#49390=CARTESIAN_POINT ( 'NONE',  ( -6.726765607527585011, -8.198316282514451103, -6.726765607527558366 ) ) ;
#49407=UNCERTAINTY_MEASURE_WITH_UNIT (LENGTH_MEASURE( 1.000000000000000082E-05 ), #31107, 'distance_accuracy_value', 'NONE');
#49433=CARTESIAN_POINT ( 'NONE',  ( -1.114695358586659246E-15, -9.448428148670501514, 9.261795338153662627 ) ) ;
#49439=TOROIDAL_SURFACE ( 'NONE', #125580, 6.330000000000000959, 0.08000000000000000167 ) ;
#49441=CARTESIAN_POINT ( 'NONE',  ( 10.35569247086020894, 1.405922845961228962, 6.063183772476113731 ) ) ;
#49463=EDGE_CURVE ( 'NONE', #53554, #168636, #145486, .T. ) ;
#49471=( NAMED_UNIT ( * ) PLANE_ANGLE_UNIT ( ) SI_UNIT ( $, .RADIAN. ) );
#49561=DIRECTION ( 'NONE',  ( 0.000000000000000000, -1.561251128379122346E-12, 1.000000000000000000 ) ) ;
#49578=DIRECTION ( 'NONE',  ( -1.000000000000000000, -1.561251128379122346E-12, 0.000000000000000000 ) ) ;
#49607=FACE_OUTER_BOUND ( 'NONE', #166501, .T. ) ;
#49632=EDGE_CURVE ( 'NONE', #70421, #31187, #111433, .T. ) ;
#49661=CIRCLE ( 'NONE', #4639, 10.99999999999999112 ) ;
#49694=CARTESIAN_POINT ( 'NONE',  ( 0.000000000000000000, -7.666862915010147717, 0.000000000000000000 ) ) ;
#49696=SURFACE_STYLE_USAGE ( .BOTH. , #102720 ) ;
#49736=AXIS2_PLACEMENT_3D ( 'NONE', #20872, #150925, #136801 ) ;
#49783=CARTESIAN_POINT ( 'NONE',  ( 9.579665964948882007, -7.473374494045003757, 1.734723475976807094E-15 ) ) ;
#49813=ADVANCED_FACE ( 'NONE', ( #92265 ), #190832, .T. ) ;
#49820=CARTESIAN_POINT ( 'NONE',  ( 8.923337013803674722, 2.630042260599927850, 8.023366178422937978 ) ) ;
#49828=CARTESIAN_POINT ( 'NONE',  ( 0.000000000000000000, -0.9200000000000041478, 0.000000000000000000 ) ) ;
#49837=SURFACE_STYLE_USAGE ( .BOTH. , #82327 ) ;
#49862=CARTESIAN_POINT ( 'NONE',  ( 9.030096778091543541, 1.000000000000000888, 7.742171412064401181 ) ) ;
#49868=VERTEX_POINT ( 'NONE', #59723 ) ;
#49886=CARTESIAN_POINT ( 'NONE',  ( 0.07999999999999327094, -9.900000000000005684, 10.91970695577496286 ) ) ;
#49949=MECHANICAL_DESIGN_GEOMETRIC_PRESENTATION_REPRESENTATION('',(#108926),#177984);
#49963=CARTESIAN_POINT ( 'NONE',  ( -7.721398836998405457, -6.134628647623499909, -7.721398836998363713 ) ) ;
#50012=VERTEX_POINT ( 'NONE', #212558 ) ;
#50018=CARTESIAN_POINT ( 'NONE',  ( 10.10516068267231127, -6.085430761754773599, -0.4362825330288160330 ) ) ;
#50032=DIRECTION ( 'NONE',  ( -0.6123724356957922499, 0.7071067811865537900, -0.3535533905932651266 ) ) ;
#50039=FACE_OUTER_BOUND ( 'NONE', #21725, .T. ) ;
#50049=AXIS2_PLACEMENT_3D ( 'NONE', #157499, #45888, #92515 ) ;
#50062=ORIENTED_EDGE ( 'NONE', *, *, #186853, .T. ) ;
#50087=VERTEX_POINT ( 'NONE', #150785 ) ;
#50094=DIRECTION ( 'NONE',  ( 0.000000000000000000, 1.000000000000000000, 0.000000000000000000 ) ) ;
#50102=CARTESIAN_POINT ( 'NONE',  ( -6.381095703207960490, -8.200000000000001066, -7.037870247915966715 ) ) ;
#50117=ORIENTED_EDGE ( 'NONE', *, *, #77763, .F. ) ;
#50130=CARTESIAN_POINT ( 'NONE',  ( 0.09264309395030836947, -9.919020119916163836, 9.499548513212900502 ) ) ;
#50138=B_SPLINE_CURVE_WITH_KNOTS ( 'NONE', 3,
 ( #206693, #58321, #92976, #208810 ),
 .UNSPECIFIED., .F., .F.,
 ( 4, 4 ),
 ( 0.000000000000000000, 6.033646489354581229E-05 ),
 .UNSPECIFIED. ) ;
#50247=CARTESIAN_POINT ( 'NONE',  ( -0.08058608058609216529, -9.900000000000005684, -10.99970480893080271 ) ) ;
#50250=COLOUR_RGB ( '', 0.72549020, 0.75294118, 0.79215686) ;
#50251=B_SPLINE_CURVE_WITH_KNOTS ( 'NONE', 3,
 ( #164965, #182267, #198509, #69570, #97857, #149794, #98913, #19767, #16557, #163920 ),
 .UNSPECIFIED., .F., .F.,
 ( 4, 2, 2, 2, 4 ),
 ( 0.000000000000000000, 0.0002554020510936943849, 0.0005108041021873887698, 0.0007662061532810831004, 0.001021608204374777540 ),
 .UNSPECIFIED. ) ;
#50278=ORIENTED_EDGE ( 'NONE', *, *, #78480, .T. ) ;
#50321=CARTESIAN_POINT ( 'NONE',  ( 0.000000000000000000, 0.03624871340549007392, 0.000000000000000000 ) ) ;
#50348=AXIS2_PLACEMENT_3D ( 'NONE', #26717, #89614, #191337 ) ;
#50361=CARTESIAN_POINT ( 'NONE',  ( 9.597801448743146224, -7.025535116234753907, -0.01424860406303069330 ) ) ;
#50387=LINE ( 'NONE', #37326, #51116 ) ;
#50401=EDGE_CURVE ( 'NONE', #94234, #78199, #152966, .T. ) ;
#50406=ORIENTED_EDGE ( 'NONE', *, *, #182418, .F. ) ;
#50416=CARTESIAN_POINT ( 'NONE',  ( 10.97067990664313264, -5.250949308401987814, -0.2977236940312545377 ) ) ;
#50430=ORIENTED_EDGE ( 'NONE', *, *, #43529, .T. ) ;
#50481=( BOUNDED_SURFACE ( )  B_SPLINE_SURFACE ( 3, 2, ( 
 ( #96341, #111566, #146160 ),
 ( #207919, #77927, #210043 ),
 ( #76853, #127851, #125700 ),
 ( #45450, #177574, #29187 ) ),
 .UNSPECIFIED., .F., .F., .F. ) 
 B_SPLINE_SURFACE_WITH_KNOTS ( ( 4, 4 ),
 ( 3, 3 ),
 ( 0.005025772024296196530, 0.008052159968022380709 ),
 ( 0.000000000000000000, 1.000000000000000000 ),
 .UNSPECIFIED. ) 
 GEOMETRIC_REPRESENTATION_ITEM ( )  RATIONAL_B_SPLINE_SURFACE ( (
 ( 1.000000000000000000, 0.7187737999613678097, 1.000000000000000000),
 ( 1.000000000000000000, 0.7186585579881044072, 1.000000000000000000),
 ( 1.000000000000000000, 0.7185467277397536989, 1.000000000000000000),
 ( 1.000000000000000000, 0.7184380228464064544, 1.000000000000000000) ) ) 
 REPRESENTATION_ITEM ( '' )  SURFACE ( )  );
#50507=ORIENTED_EDGE ( 'NONE', *, *, #54338, .F. ) ;
#50516=ORIENTED_EDGE ( 'NONE', *, *, #143132, .F. ) ;
#50594=CARTESIAN_POINT ( 'NONE',  ( 0.000000000000000000, -6.527411821100059797, 0.000000000000000000 ) ) ;
#50598=CARTESIAN_POINT ( 'NONE',  ( 10.91970695577495043, -5.907420853759282053, 8.673617379884035472E-15 ) ) ;
#50606=B_SPLINE_CURVE_WITH_KNOTS ( 'NONE', 3,
 ( #213463, #31558, #148501, #47827, #29425, #163690, #13152, #131243, #82412, #66133, #15272, #78156, #128080, #95516, #113939, #197230 ),
 .UNSPECIFIED., .F., .F.,
 ( 4, 3, 3, 3, 3, 4 ),
 ( 0.000000000000000000, 3.357822776042505863E-05, 6.715700932737113144E-05, 0.0001007352753633138738, 0.0001343124815392893027, 0.0001562160020015778686 ),
 .UNSPECIFIED. ) ;
#50626=CARTESIAN_POINT ( 'NONE',  ( 8.081892667527529994, -5.166862915010145052, -7.462104991928515396 ) ) ;
#50636=VECTOR ( 'NONE', #119490, 1000.000000000000000 ) ;
#50646=CARTESIAN_POINT ( 'NONE',  ( 10.18461545817735470, 3.956598013261175772, -5.433575010662928584 ) ) ;
#50652=ORIENTED_EDGE ( 'NONE', *, *, #212049, .F. ) ;
#50663=EDGE_CURVE ( 'NONE', #109724, #24478, #201765, .T. ) ;
#50671=CARTESIAN_POINT ( 'NONE',  ( -6.724721492623500829, -6.244189044378177122, -7.341412881700118298 ) ) ;
#50677=CARTESIAN_POINT ( 'NONE',  ( 9.578659721986364062, -9.971093151297267809, -0.1384029864567958568 ) ) ;
#50682=ORIENTED_EDGE ( 'NONE', *, *, #89522, .F. ) ;
#50717=B_SPLINE_CURVE_WITH_KNOTS ( 'NONE', 3,
 ( #51103, #132395, #169110, #147551, #213573, #117228, #183226, #150753, #85729, #2315 ),
 .UNSPECIFIED., .F., .F.,
 ( 4, 2, 2, 2, 4 ),
 ( 0.000000000000000000, 0.0002216178067634642641, 0.0004432356135269285282, 0.0006648534202903928466, 0.0008864712270538553218 ),
 .UNSPECIFIED. ) ;
#50767=DIRECTION ( 'NONE',  ( 0.000000000000000000, 0.000000000000000000, 1.000000000000000000 ) ) ;
#50797=STYLED_ITEM ( 'NONE', ( #148191 ), #197936 ) ;
#50825=CARTESIAN_POINT ( 'NONE',  ( 1.396097351027982424E-15, 0.000000000000000000, -11.29999999999999893 ) ) ;
#50845=VERTEX_POINT ( 'NONE', #24530 ) ;
#50853=FACE_OUTER_BOUND ( 'NONE', #163849, .T. ) ;
#50854=CARTESIAN_POINT ( 'NONE',  ( 2.486770427477404954, 2.630042260599927850, -11.73951962969540119 ) ) ;
#50884=DIRECTION ( 'NONE',  ( -0.000000000000000000, 1.000000000000000000, -0.000000000000000000 ) ) ;
#50925=CIRCLE ( 'NONE', #185715, 0.07999999999999993228 ) ;
#50937=CARTESIAN_POINT ( 'NONE',  ( 2.493461049780987260, 3.507114751586604129, -11.73081193161139169 ) ) ;
#50950=EDGE_CURVE ( 'NONE', #173465, #197280, #165743, .T. ) ;
#50953=CYLINDRICAL_SURFACE ( 'NONE', #163581, 10.99999999999999112 ) ;
#50963=SURFACE_STYLE_FILL_AREA ( #86655 ) ;
#50966=ADVANCED_FACE ( 'NONE', ( #185601 ), #174524, .T. ) ;
#50968=DIRECTION ( 'NONE',  ( -0.000000000000000000, -1.000000000000000000, -0.000000000000000000 ) ) ;
#51005=DIRECTION ( 'NONE',  ( 8.881784197001252323E-16, 0.000000000000000000, -1.000000000000000000 ) ) ;
#51032=CARTESIAN_POINT ( 'NONE',  ( -7.591565991045862383, -6.646943093533998592, -7.792125355486802185 ) ) ;
#51087=CARTESIAN_POINT ( 'NONE',  ( 9.578206935421269108, -9.746166700192988586, -0.1671882239536438552 ) ) ;
#51089=CARTESIAN_POINT ( 'NONE',  ( -2.315885204923618268, 3.829536045110814690, 11.43841291973005703 ) ) ;
#51103=CARTESIAN_POINT ( 'NONE',  ( -1.734723475976807094E-15, -8.407420853759283830, -10.91970695577494332 ) ) ;
#51106=ORIENTED_EDGE ( 'NONE', *, *, #108140, .F. ) ;
#51116=VECTOR ( 'NONE', #85011, 1000.000000000000000 ) ;
#51127=EDGE_CURVE ( 'NONE', #35700, #49868, #111732, .T. ) ;
#51152=VECTOR ( 'NONE', #211698, 1000.000000000000000 ) ;
#51164=VECTOR ( 'NONE', #16224, 1000.000000000000000 ) ;
#51169=CARTESIAN_POINT ( 'NONE',  ( 9.499701791763563108, -9.918130724412307586, -0.07530116296179023561 ) ) ;
#51191=VERTEX_POINT ( 'NONE', #105465 ) ;
#51202=DIRECTION ( 'NONE',  ( 0.000000000000000000, 0.000000000000000000, 1.000000000000000000 ) ) ;
#51221=CARTESIAN_POINT ( 'NONE',  ( 0.000000000000000000, 0.000000000000000000, 11.29999999999998828 ) ) ;
#51235=CARTESIAN_POINT ( 'NONE',  ( 9.579603127937247109, -9.746166700193986898, -0.08720040834114990702 ) ) ;
#51279=( LENGTH_UNIT ( ) NAMED_UNIT ( * ) SI_UNIT ( .MILLI., .METRE. ) );
#51433=CARTESIAN_POINT ( 'NONE',  ( 9.483257663144033955, -6.709848117146358426, -0.3912817730722052412 ) ) ;
#51450=CARTESIAN_POINT ( 'NONE',  ( -6.576431128232853141, -6.604036961759847557, -7.015831072854298078 ) ) ;
#51497=CARTESIAN_POINT ( 'NONE',  ( 0.000000000000000000, -9.746166700180788567, 9.579665964948883783 ) ) ;
#51500=CIRCLE ( 'NONE', #6485, 9.616019636405015447 ) ;
#51512=ORIENTED_EDGE ( 'NONE', *, *, #55286, .F. ) ;
#51538=SHAPE_DEFINITION_REPRESENTATION ( #124996, #63688 ) ;
#51596=FACE_OUTER_BOUND ( 'NONE', #169447, .T. ) ;
#51613=DIRECTION ( 'NONE',  ( -7.610300982150707428E-15, -1.000000000000000000, 7.722633184682877167E-15 ) ) ;
#51624=CARTESIAN_POINT ( 'NONE',  ( -7.555533889508359024E-14, -9.900000000000005684, 9.500331257164617682 ) ) ;
#51645=CARTESIAN_POINT ( 'NONE',  ( -7.749822179018673651, -6.479141885268356660, 7.806953216197599410 ) ) ;
#51649=CARTESIAN_POINT ( 'NONE',  ( 0.000000000000000000, 7.849261790823902629, 9.499999999999992895 ) ) ;
#51655=AXIS2_PLACEMENT_3D ( 'NONE', #138, #116115, #53190 ) ;
#51670=ADVANCED_FACE ( 'NONE', ( #60951 ), #105548, .F. ) ;
#51675=CARTESIAN_POINT ( 'NONE',  ( -7.004500933659051576, -6.920331743269724889, 7.004500933659075557 ) ) ;
#51705=VERTEX_POINT ( 'NONE', #112973 ) ;
#51716=CARTESIAN_POINT ( 'NONE',  ( -9.484899655072714708, -6.713792789267452932, 0.3525790917593041307 ) ) ;
#51759=( NAMED_UNIT ( * ) PLANE_ANGLE_UNIT ( ) SI_UNIT ( $, .RADIAN. ) );
#51769=EDGE_CURVE ( 'NONE', #5447, #54210, #67494, .T. ) ;
#51777=CARTESIAN_POINT ( 'NONE',  ( 0.09263662810811511272, -9.999999999999994671, 10.91955560153697746 ) ) ;
#51827=CIRCLE ( 'NONE', #44881, 0.08000000000000009881 ) ;
#51850=CARTESIAN_POINT ( 'NONE',  ( -9.554207839743737551, -7.792803924024828355, 0.03436587256740113172 ) ) ;
#51873=CARTESIAN_POINT ( 'NONE',  ( -1.040834085586084257E-14, -7.473374494045017968, -9.579665964948867796 ) ) ;
#51899=EDGE_CURVE ( 'NONE', #76877, #184758, #47934, .T. ) ;
#51969=CARTESIAN_POINT ( 'NONE',  ( -9.495347311156809411, -6.857257212219918685, 3.422217897015904270E-15 ) ) ;
#52012=DIRECTION ( 'NONE',  ( 0.000000000000000000, -1.000000000000000000, 0.000000000000000000 ) ) ;
#52027=ORIENTED_EDGE ( 'NONE', *, *, #10396, .T. ) ;
#52034=EDGE_CURVE ( 'NONE', #74902, #127875, #204886, .T. ) ;
#52063=EDGE_CURVE ( 'NONE', #108531, #194102, #106329, .T. ) ;
#52077=ADVANCED_FACE ( 'NONE', ( #8166 ), #154432, .T. ) ;
#52097=CARTESIAN_POINT ( 'NONE',  ( 11.37385970535889257, 1.000000000000000888, -3.825613075418463627 ) ) ;
#52113=ORIENTED_EDGE ( 'NONE', *, *, #78852, .F. ) ;
#52117=EDGE_LOOP ( 'NONE', ( #164459, #73595, #35737, #193383 ) ) ;
#52135=CARTESIAN_POINT ( 'NONE',  ( 9.586610838029415049, -7.161464053357574855, -0.003376046620562692113 ) ) ;
#52181=CARTESIAN_POINT ( 'NONE',  ( 11.18654035131437219, 1.000000000000000888, -4.041720556560823852 ) ) ;
#52183=CARTESIAN_POINT ( 'NONE',  ( -7.778383330260382422, -6.134628647623486586, -7.778383330260335349 ) ) ;
#52191=ORIENTED_EDGE ( 'NONE', *, *, #172200, .F. ) ;
#52215=ORIENTED_EDGE ( 'NONE', *, *, #94831, .T. ) ;
#52219=ORIENTED_EDGE ( 'NONE', *, *, #138625, .T. ) ;
#52233=MECHANICAL_DESIGN_GEOMETRIC_PRESENTATION_REPRESENTATION('',(#121419),#79883);
#52234=CARTESIAN_POINT ( 'NONE',  ( -10.99950989413231106, -9.915617157791128733, 0.1038368378055241209 ) ) ;
#52251=CARTESIAN_POINT ( 'NONE',  ( 0.4655551865852050608, -8.176568542494919711, 9.512045263456268884 ) ) ;
#52257=VECTOR ( 'NONE', #86295, 999.9999999999998863 ) ;
#52264=CARTESIAN_POINT ( 'NONE',  ( 6.764690511086886823E-16, -5.511313137147262786, 11.00000000000000178 ) ) ;
#52270=STYLED_ITEM ( 'NONE', ( #28255 ), #165584 ) ;
#52337=CARTESIAN_POINT ( 'NONE',  ( -2.450243370979069635, 1.813773193624685254, 11.74719778151168192 ) ) ;
#52365=ORIENTED_EDGE ( 'NONE', *, *, #187963, .T. ) ;
#52396=ORIENTED_EDGE ( 'NONE', *, *, #54844, .F. ) ;
#52451=( NAMED_UNIT ( * ) PLANE_ANGLE_UNIT ( ) SI_UNIT ( $, .RADIAN. ) );
#52488=CARTESIAN_POINT ( 'NONE',  ( 9.488968570712872364, -6.747343053191950268, -0.2633404184770131717 ) ) ;
#52491=ORIENTED_EDGE ( 'NONE', *, *, #43078, .T. ) ;
#52494=CARTESIAN_POINT ( 'NONE',  ( 6.908358566921232402, -6.724344753046858081, -6.684387857553371504 ) ) ;
#52503=CARTESIAN_POINT ( 'NONE',  ( 0.3931996164520941694, -9.201308816822022507, -9.491928691057864853 ) ) ;
#52504=CARTESIAN_POINT ( 'NONE',  ( -6.776370306708066060, -7.161464053357566861, -6.781144757626042185 ) ) ;
#52512=CARTESIAN_POINT ( 'NONE',  ( 0.3561222683123154709, -6.532648913094854848, 9.473215147174819606 ) ) ;
#52541=AXIS2_PLACEMENT_3D ( 'NONE', #60853, #80303, #64057 ) ;
#52595=CARTESIAN_POINT ( 'NONE',  ( 9.581972888692709134, -7.217909409572547119, 3.990133149647489978E-13 ) ) ;
#52650=EDGE_LOOP ( 'NONE', ( #207522, #27860, #186889, #15606 ) ) ;
#52656=B_SPLINE_CURVE_WITH_KNOTS ( 'NONE', 3,
 ( #80183, #48765, #214399, #146288, #13037, #98575, #95406, #144177, #114880, #44513 ),
 .UNSPECIFIED., .F., .F.,
 ( 4, 2, 2, 2, 4 ),
 ( 7.099868766331327897E-18, 0.0002236660844579363818, 0.0004473321689158656620, 0.0006709982533737948339, 0.0008946643378317241683 ),
 .UNSPECIFIED. ) ;
#52658=AXIS2_PLACEMENT_3D ( 'NONE', #10630, #58338, #174249 ) ;
#52682=DIRECTION ( 'NONE',  ( -0.7071067811865462405, 0.000000000000000000, 0.7071067811865489050 ) ) ;
#52687=ORIENTED_EDGE ( 'NONE', *, *, #123001, .T. ) ;
#52696=DIRECTION ( 'NONE',  ( -2.664535259100375697E-15, 0.000000000000000000, -1.000000000000000000 ) ) ;
#52727=DIRECTION ( 'NONE',  ( -0.6716942845482062330, -1.762391939599642519E-12, -0.7408284471490506062 ) ) ;
#52747=CARTESIAN_POINT ( 'NONE',  ( 9.499606442108964544, -9.746166700193986898, -0.08647222121513538362 ) ) ;
#52755=VECTOR ( 'NONE', #202096, 1000.000000000000000 ) ;
#52852=B_SPLINE_CURVE_WITH_KNOTS ( 'NONE', 3,
 ( #102042, #203777, #72727, #135620, #37026, #103110 ),
 .UNSPECIFIED., .F., .F.,
 ( 4, 2, 4 ),
 ( 0.0004037790303856251119, 0.0007126936173802011359, 0.001021608204374777106 ),
 .UNSPECIFIED. ) ;
#52856=CIRCLE ( 'NONE', #32150, 10.99999999999999112 ) ;
#52870=DIRECTION ( 'NONE',  ( -0.000000000000000000, 1.000000000000000000, -0.000000000000000000 ) ) ;
#52892=( LENGTH_UNIT ( ) NAMED_UNIT ( * ) SI_UNIT ( .MILLI., .METRE. ) );
#52900=CARTESIAN_POINT ( 'NONE',  ( -9.500331257164631893, -7.473374494045002869, 1.019891195965221523E-14 ) ) ;
#52904=ORIENTED_EDGE ( 'NONE', *, *, #131239, .T. ) ;
#52943=CARTESIAN_POINT ( 'NONE',  ( 8.743186976631660556, 3.870433085555829766, 7.668514896535032932 ) ) ;
#52970=ADVANCED_FACE ( 'NONE', ( #148871 ), #90979, .T. ) ;
#52974=AXIS2_PLACEMENT_3D ( 'NONE', #164250, #65644, #46252 ) ;
#53033=CARTESIAN_POINT ( 'NONE',  ( -10.18461545817740088, 3.956598013261175772, 5.433575010662861082 ) ) ;
#53050=CARTESIAN_POINT ( 'NONE',  ( -7.777967379493323286, -6.134628647623485698, -7.664830294503433450 ) ) ;
#53057=LINE ( 'NONE', #88779, #150419 ) ;
#53060=AXIS2_PLACEMENT_3D ( 'NONE', #127579, #211912, #195687 ) ;
#53086=( NAMED_UNIT ( * ) PLANE_ANGLE_UNIT ( ) SI_UNIT ( $, .RADIAN. ) );
#53099=EDGE_CURVE ( 'NONE', #75305, #186393, #36441, .T. ) ;
#53128=CIRCLE ( 'NONE', #136171, 0.07999999999999940492 ) ;
#53175=CARTESIAN_POINT ( 'NONE',  ( 10.04733898909039702, 1.529612873802630224, 6.247711339170956890 ) ) ;
#53190=DIRECTION ( 'NONE',  ( -0.6743504407188151140, 0.000000000000000000, -0.7384114592165670343 ) ) ;
#53201=CARTESIAN_POINT ( 'NONE',  ( -7.784592198500340565, -5.601927612791713251, 7.772296586883744141 ) ) ;
#53215=CARTESIAN_POINT ( 'NONE',  ( 9.498884310698278099, -9.746166700192997467, -0.1658036423878402332 ) ) ;
#53217=CARTESIAN_POINT ( 'NONE',  ( -2.483409115735836892, 3.555461883994699868, 11.68352130004407030 ) ) ;
#53233=CARTESIAN_POINT ( 'NONE',  ( 0.000000000000000000, -6.893137084989842123, 0.000000000000000000 ) ) ;
#53238=DIRECTION ( 'NONE',  ( -0.05727394217551268901, 3.884134901109067902E-16, -0.9983585005135560131 ) ) ;
#53275=DIRECTION ( 'NONE',  ( 0.000000000000000000, 1.000000000000000000, 0.000000000000000000 ) ) ;
#53288=CARTESIAN_POINT ( 'NONE',  ( -6.500815859342971237, -6.554751161430533379, -6.901817408925770891 ) ) ;
#53294=CARTESIAN_POINT ( 'NONE',  ( -6.625366561259609988, -8.010031549403139550, -6.808607288253771372 ) ) ;
#53315=CARTESIAN_POINT ( 'NONE',  ( 6.576431128232845147, -6.604036961759876867, 7.015831072854276762 ) ) ;
#53351=ORIENTED_EDGE ( 'NONE', *, *, #94831, .F. ) ;
#53411=CARTESIAN_POINT ( 'NONE',  ( 0.000000000000000000, 0.9200000000000041478, 0.000000000000000000 ) ) ;
#53448=VERTEX_POINT ( 'NONE', #163824 ) ;
#53451=CARTESIAN_POINT ( 'NONE',  ( 7.721398836998401904, -6.134628647623499909, 7.721398836998376147 ) ) ;
#53454=CARTESIAN_POINT ( 'NONE',  ( 0.07933194154555710254, -7.215597533182092960, -9.499668754385616865 ) ) ;
#53455=B_SPLINE_CURVE_WITH_KNOTS ( 'NONE', 3,
 ( #26047, #73742, #157147, #124718, #175527, #24984 ),
 .UNSPECIFIED., .F., .F.,
 ( 4, 2, 4 ),
 ( 0.000000000000000000, 0.001226111284895916101, 0.002452222569791831768 ),
 .UNSPECIFIED. ) ;
#53473=ORIENTED_EDGE ( 'NONE', *, *, #36152, .T. ) ;
#53479=CARTESIAN_POINT ( 'NONE',  ( 7.712474369503348193, -6.289226506789209914, 7.712474369503325100 ) ) ;
#53487=EDGE_CURVE ( 'NONE', #69637, #19069, #77036, .T. ) ;
#53495=MECHANICAL_DESIGN_GEOMETRIC_PRESENTATION_REPRESENTATION('',(#39728),#181641);
#53503=EDGE_CURVE ( 'NONE', #187284, #175139, #133478, .T. ) ;
#53533=CARTESIAN_POINT ( 'NONE',  ( -1.734723475976807094E-15, -6.134628647623513231, -10.91970695577494332 ) ) ;
#53547=EDGE_CURVE ( 'NONE', #163622, #163559, #97765, .T. ) ;
#53554=VERTEX_POINT ( 'NONE', #147570 ) ;
#53561=CARTESIAN_POINT ( 'NONE',  ( 6.864213375409820905, -6.776276029125531508, -6.558483974470185274 ) ) ;
#53571=CARTESIAN_POINT ( 'NONE',  ( 10.99943592164172479, -8.240513804456435665, -0.1113975120798833818 ) ) ;
#53640=CARTESIAN_POINT ( 'NONE',  ( 9.579665964935223599, -7.246166700194470067, 5.204170427930421283E-15 ) ) ;
#53665=CARTESIAN_POINT ( 'NONE',  ( 9.579665964935223599, -7.246166700194470067, 5.204170427930421283E-15 ) ) ;
#53699=DIRECTION ( 'NONE',  ( 0.000000000000000000, 1.000000000000000000, 0.000000000000000000 ) ) ;
#53718=CARTESIAN_POINT ( 'NONE',  ( -10.38894090356600231, 1.970899860167847795, 5.551243578534467815 ) ) ;
#53757=FACE_OUTER_BOUND ( 'NONE', #52650, .T. ) ;
#53762=ORIENTED_EDGE ( 'NONE', *, *, #2635, .T. ) ;
#53773=CARTESIAN_POINT ( 'NONE',  ( 0.000000000000000000, 4.000000000000003553, -11.50000000000000000 ) ) ;
#53779=LINE ( 'NONE', #106849, #151305 ) ;
#53787=AXIS2_PLACEMENT_3D ( 'NONE', #195317, #141269, #43748 ) ;
#53796=CARTESIAN_POINT ( 'NONE',  ( -10.91808280586644564, -9.921948886890824326, 0.1881369732364187586 ) ) ;
#53822=ORIENTED_EDGE ( 'NONE', *, *, #37827, .T. ) ;
#53827=ORIENTED_EDGE ( 'NONE', *, *, #3571, .F. ) ;
#53829=DIRECTION ( 'NONE',  ( -0.9781476007338056888, 0.000000000000000000, -0.2079116908177593703 ) ) ;
#53838=DIRECTION ( 'NONE',  ( 0.000000000000000000, -1.000000000000000000, 0.000000000000000000 ) ) ;
#53854=DIRECTION ( 'NONE',  ( 0.000000000000000000, -1.000000000000000000, 0.000000000000000000 ) ) ;
#53881=CARTESIAN_POINT ( 'NONE',  ( -6.844806938814769204, -6.074287852078585459, -7.461813752226478691 ) ) ;
#53917=CARTESIAN_POINT ( 'NONE',  ( 0.000000000000000000, -2.079999999999998295, 10.99999999999999112 ) ) ;
#53965=AXIS2_PLACEMENT_3D ( 'NONE', #120525, #204865, #8826 ) ;
#53968=CARTESIAN_POINT ( 'NONE',  ( 1.355252715606880543E-15, 3.019799309333501824, -12.05075272264721242 ) ) ;
#54010=CARTESIAN_POINT ( 'NONE',  ( -0.4299312922663480752, -6.708819892820486963, -9.481437597266031858 ) ) ;
#54046=CARTESIAN_POINT ( 'NONE',  ( 8.914213045750530640, 3.487142912321096855, 8.026393478126198744 ) ) ;
#54068=EDGE_CURVE ( 'NONE', #29554, #66830, #108344, .T. ) ;
#54086=CARTESIAN_POINT ( 'NONE',  ( 8.002408263929950749, -6.836568542494916301, -7.346809171966858010 ) ) ;
#54087=LINE ( 'NONE', #151596, #3073 ) ;
#54095=CARTESIAN_POINT ( 'NONE',  ( 0.09510031644101717141, -6.698521824825868443, 10.99968117833243042 ) ) ;
#54122=ORIENTED_EDGE ( 'NONE', *, *, #86771, .T. ) ;
#54137=CARTESIAN_POINT ( 'NONE',  ( 0.000000000000000000, 0.000000000000000000, 0.000000000000000000 ) ) ;
#54141=CARTESIAN_POINT ( 'NONE',  ( -10.32992389895503393, 1.000000000000000888, -6.106772653521458594 ) ) ;
#54157=EDGE_LOOP ( 'NONE', ( #201472, #22586 ) ) ;
#54162=SURFACE_SIDE_STYLE ('',( #50963 ) ) ;
#54180=CARTESIAN_POINT ( 'NONE',  ( -0.08000000000000367928, -9.746166700180788567, -9.579665964948867796 ) ) ;
#54202=AXIS2_PLACEMENT_3D ( 'NONE', #90986, #158114, #75782 ) ;
#54210=VERTEX_POINT ( 'NONE', #125805 ) ;
#54222=ADVANCED_FACE ( 'NONE', ( #59647 ), #192831, .T. ) ;
#54236=CARTESIAN_POINT ( 'NONE',  ( -6.781144757626059061, -7.161464053357560644, 6.776370306708066948 ) ) ;
#54245=ORIENTED_EDGE ( 'NONE', *, *, #124333, .T. ) ;
#54246=ORIENTED_EDGE ( 'NONE', *, *, #66712, .F. ) ;
#54288=LINE ( 'NONE', #104106, #73538 ) ;
#54294=CARTESIAN_POINT ( 'NONE',  ( -10.85717823004580040, -6.836271227032190367, 0.3852658704378439936 ) ) ;
#54297=( BOUNDED_SURFACE ( )  B_SPLINE_SURFACE ( 3, 2, ( 
 ( #123462, #155868, #138560 ),
 ( #41066, #173200, #206733 ),
 ( #26909, #58363, #42135 ),
 ( #108247, #207792, #59420 ),
 ( #125576, #93016, #159059 ),
 ( #10655, #76728, #83929 ),
 ( #66584, #52503, #163082 ),
 ( #130641, #14663, #151092 ) ),
 .UNSPECIFIED., .F., .F., .T. ) 
 B_SPLINE_SURFACE_WITH_KNOTS ( ( 4, 2, 2, 4 ),
 ( 3, 3 ),
 ( 0.000000000000000000, 0.0004912655988793406025, 0.0007368983983190109579, 0.0009825311977586812049 ),
 ( 0.000000000000000000, 1.000000000000000000 ),
 .UNSPECIFIED. ) 
 GEOMETRIC_REPRESENTATION_ITEM ( )  RATIONAL_B_SPLINE_SURFACE ( (
 ( 1.000000000000000000, 0.7100530722026748842, 1.000000000000000000),
 ( 1.000000000000000000, 0.6561915434212005627, 1.000000000000000000),
 ( 1.000000000000000000, 0.5915413786749507130, 1.000000000000000000),
 ( 1.000000000000000000, 0.4908282809844877748, 1.000000000000000000),
 ( 1.000000000000000000, 0.4560392263211181518, 1.000000000000000000),
 ( 1.000000000000000000, 0.3997350557756911282, 1.000000000000000000),
 ( 1.000000000000000000, 0.3799210206805033185, 1.000000000000000000),
 ( 1.000000000000000000, 0.3826834323650902259, 1.000000000000000000) ) ) 
 REPRESENTATION_ITEM ( '' )  SURFACE ( )  );
#54326=EDGE_CURVE ( 'NONE', #74349, #116385, #28806, .T. ) ;
#54328=ORIENTED_EDGE ( 'NONE', *, *, #95057, .F. ) ;
#54338=EDGE_CURVE ( 'NONE', #130349, #182554, #212375, .T. ) ;
#54340=CARTESIAN_POINT ( 'NONE',  ( 10.23127510237375937, 3.700502905159951172, -5.878152162067817876 ) ) ;
#54346=VERTEX_POINT ( 'NONE', #143079 ) ;
#54363=CARTESIAN_POINT ( 'NONE',  ( 0.1523027874134948167, -6.731960136058440902, 9.611344009005483358 ) ) ;
#54391=CARTESIAN_POINT ( 'NONE',  ( 6.692370362268437844, -7.020359948791616844, 6.743487189264702586 ) ) ;
#54403=CARTESIAN_POINT ( 'NONE',  ( 6.781144757626058173, -7.161464053357574855, -6.776370306708051849 ) ) ;
#54423=CARTESIAN_POINT ( 'NONE',  ( 7.900729602272468455, -6.805008568744117525, -7.460470246983064158 ) ) ;
#54433=CARTESIAN_POINT ( 'NONE',  ( 0.4659925305415726360, -6.893137084989842123, 10.91005274787796608 ) ) ;
#54437=CARTESIAN_POINT ( 'NONE',  ( 0.01979919457416898926, -6.863887352872461989, -9.496663240426190811 ) ) ;
#54475=CARTESIAN_POINT ( 'NONE',  ( 0.1588445005388132991, -6.630981418884858591, 9.484513308955760280 ) ) ;
#54477=DIRECTION ( 'NONE',  ( 0.000000000000000000, 0.000000000000000000, 1.000000000000000000 ) ) ;
#54518=CARTESIAN_POINT ( 'NONE',  ( -7.453913518772577795, -5.212532583863431768, -8.072398248062480519 ) ) ;
#54527=PLANE ( 'NONE',  #130360 ) ;
#54543=SURFACE_STYLE_FILL_AREA ( #153112 ) ;
#54572=( NAMED_UNIT ( * ) SI_UNIT ( $, .STERADIAN. ) SOLID_ANGLE_UNIT ( ) );
#54610=CARTESIAN_POINT ( 'NONE',  ( -11.00009153390426597, -6.553298220693309695, 0.005414006223999826353 ) ) ;
#54621=ORIENTED_EDGE ( 'NONE', *, *, #37827, .F. ) ;
#54622=CARTESIAN_POINT ( 'NONE',  ( 9.477100695693454924, -6.554910290221281244, -0.2834499523633078333 ) ) ;
#54631=VERTEX_POINT ( 'NONE', #202712 ) ;
#54646=CARTESIAN_POINT ( 'NONE',  ( 0.01083140255524605265, -7.162053774861989908, 9.500385102287577155 ) ) ;
#54652=AXIS2_PLACEMENT_3D ( 'NONE', #43, #19508, #66107 ) ;
#54672=DIRECTION ( 'NONE',  ( 0.000000000000000000, 0.000000000000000000, -1.000000000000000000 ) ) ;
#54696=EDGE_CURVE ( 'NONE', #100951, #29554, #23625, .T. ) ;
#54787=ORIENTED_EDGE ( 'NONE', *, *, #1928, .F. ) ;
#54802=DIRECTION ( 'NONE',  ( 0.000000000000000000, 0.000000000000000000, -1.000000000000000000 ) ) ;
#54816=CARTESIAN_POINT ( 'NONE',  ( 0.07933543236773606122, -9.910877263631659773, 9.499668725233687994 ) ) ;
#54830=ORIENTED_EDGE ( 'NONE', *, *, #64219, .F. ) ;
#54836=CARTESIAN_POINT ( 'NONE',  ( 0.000000000000000000, -9.999999999999994671, 10.99999999999999112 ) ) ;
#54840=CARTESIAN_POINT ( 'NONE',  ( -0.4637852190931971985, -7.024005807102851051, -10.66594404249593531 ) ) ;
#54844=EDGE_CURVE ( 'NONE', #91101, #116385, #108504, .T. ) ;
#54859=ORIENTED_EDGE ( 'NONE', *, *, #138938, .F. ) ;
#54867=CARTESIAN_POINT ( 'NONE',  ( 0.4373225248172890045, -5.223431457505089526, 10.96785329849812385 ) ) ;
#54886=EDGE_LOOP ( 'NONE', ( #93422, #189119, #106476, #115247 ) ) ;
#54893=CARTESIAN_POINT ( 'NONE',  ( 0.000000000000000000, -9.919999999999998153, 0.000000000000000000 ) ) ;
#54928=EDGE_LOOP ( 'NONE', ( #190275, #95401, #153719, #46724 ) ) ;
#54969=CIRCLE ( 'NONE', #34238, 0.08000000000000020983 ) ;
#54970=CARTESIAN_POINT ( 'NONE',  ( -10.99943594186085605, -9.910930717204488261, 0.1113955156350721065 ) ) ;
#54983=EDGE_CURVE ( 'NONE', #28024, #121080, #164648, .T. ) ;
#55004=MECHANICAL_DESIGN_GEOMETRIC_PRESENTATION_REPRESENTATION('',(#61809),#210527);
#55023=AXIS2_PLACEMENT_3D ( 'NONE', #167253, #18839, #35095 ) ;
#55041=VERTEX_POINT ( 'NONE', #12677 ) ;
#55048=ORIENTED_EDGE ( 'NONE', *, *, #62840, .T. ) ;
#55053=( LENGTH_UNIT ( ) NAMED_UNIT ( * ) SI_UNIT ( .MILLI., .METRE. ) );
#55068=TOROIDAL_SURFACE ( 'NONE', #183232, 6.330000000000000959, 0.08000000000000000167 ) ;
#55148=EDGE_LOOP ( 'NONE', ( #67836, #66824, #103105, #88537, #46654 ) ) ;
#55150=CARTESIAN_POINT ( 'NONE',  ( 8.103009739377982967, -6.893137084989842123, -7.439168848974014203 ) ) ;
#55151=AXIS2_PLACEMENT_3D ( 'NONE', #7899, #57739, #169348 ) ;
#55231=CARTESIAN_POINT ( 'NONE',  ( -10.91804383151481339, -8.407420853759283830, 0.1905751639681794174 ) ) ;
#55258=DIRECTION ( 'NONE',  ( -0.000000000000000000, 1.000000000000000000, -0.000000000000000000 ) ) ;
#55275=ORIENTED_EDGE ( 'NONE', *, *, #178012, .F. ) ;
#55286=EDGE_CURVE ( 'NONE', #45686, #133641, #146497, .T. ) ;
#55292=DIRECTION ( 'NONE',  ( 0.04888523518676889112, 8.339466111204228823E-16, 0.9988044021632737079 ) ) ;
#55294=CARTESIAN_POINT ( 'NONE',  ( 7.968353659517096510, -5.197284395437338667, -7.583532603600771083 ) ) ;
#55309=( GEOMETRIC_REPRESENTATION_CONTEXT ( 3 ) GLOBAL_UNCERTAINTY_ASSIGNED_CONTEXT ( ( #129681 ) ) GLOBAL_UNIT_ASSIGNED_CONTEXT ( ( #107100, #142776, #123384 ) ) REPRESENTATION_CONTEXT ( 'NONE', 'WORKASPACE' ) );
#55336=CARTESIAN_POINT ( 'NONE',  ( -7.836017471263608591, -5.361065518611685121, 7.720011280421910094 ) ) ;
#55353=DIRECTION ( 'NONE',  ( 0.000000000000000000, 1.000000000000000000, 0.000000000000000000 ) ) ;
#55403=ORIENTED_EDGE ( 'NONE', *, *, #94862, .F. ) ;
#55414=VERTEX_POINT ( 'NONE', #97173 ) ;
#55450=CARTESIAN_POINT ( 'NONE',  ( 6.761775799041450874, -7.009934032699937312, 6.672971353125840999 ) ) ;
#55456=DIRECTION ( 'NONE',  ( 0.000000000000000000, 0.000000000000000000, -1.000000000000000000 ) ) ;
#55498=CARTESIAN_POINT ( 'NONE',  ( -0.2834499351972725179, -6.554910260573307390, -9.477100694337659448 ) ) ;
#55544=DIRECTION ( 'NONE',  ( 0.000000000000000000, 1.000000000000000000, 0.000000000000000000 ) ) ;
#55609=SURFACE_STYLE_USAGE ( .BOTH. , #137941 ) ;
#55655=DIRECTION ( 'NONE',  ( 0.000000000000000000, 0.000000000000000000, 1.000000000000000000 ) ) ;
#55674=ORIENTED_EDGE ( 'NONE', *, *, #77512, .F. ) ;
#55691=CARTESIAN_POINT ( 'NONE',  ( 6.781144757626056396, -7.161464053357567749, -6.776370306708062508 ) ) ;
#55701=CARTESIAN_POINT ( 'NONE',  ( -0.08000000000000194456, -9.999999999999994671, -10.91970695577494865 ) ) ;
#55702=CARTESIAN_POINT ( 'NONE',  ( -6.770610912236891821, -7.154544010627095219, -6.663994888585869525 ) ) ;
#55712=CARTESIAN_POINT ( 'NONE',  ( 4.232369794311310053E-13, -9.350066838357705024, 9.500000000000001776 ) ) ;
#55754=ORIENTED_EDGE ( 'NONE', *, *, #98691, .F. ) ;
#55863=CARTESIAN_POINT ( 'NONE',  ( 10.94305301526625840, -8.100264386820958507, -0.2223449190352319027 ) ) ;
#55902=CARTESIAN_POINT ( 'NONE',  ( 0.000000000000000000, -0.02379966007286238305, 0.000000000000000000 ) ) ;
#55930=CARTESIAN_POINT ( 'NONE',  ( -10.91805698906626887, -9.914767083041231999, 0.1897524941850696201 ) ) ;
#55936=CARTESIAN_POINT ( 'NONE',  ( 2.467126471220339567, 3.603011019375355062, -11.63837686854860998 ) ) ;
#55952=ORIENTED_EDGE ( 'NONE', *, *, #119448, .F. ) ;
#55960=ORIENTED_EDGE ( 'NONE', *, *, #106666, .F. ) ;
#56052=CARTESIAN_POINT ( 'NONE',  ( -5.204170427930421283E-15, -5.907420853759282053, 10.91970695577496997 ) ) ;
#56103=CARTESIAN_POINT ( 'NONE',  ( 1.409462824231155764E-15, 2.018041202053853400, -12.16970660573436014 ) ) ;
#56127=SURFACE_SIDE_STYLE ('',( #5201 ) ) ;
#56134=DIRECTION ( 'NONE',  ( 0.000000000000000000, 0.000000000000000000, 1.000000000000000000 ) ) ;
#56146=CARTESIAN_POINT ( 'NONE',  ( -0.01424860406280193531, -7.025535116234850719, -9.597801448745755692 ) ) ;
#56164=CARTESIAN_POINT ( 'NONE',  ( 0.000000000000000000, -7.154544010627095219, 0.000000000000000000 ) ) ;
#56168=( BOUNDED_SURFACE ( )  B_SPLINE_SURFACE ( 3, 2, ( 
 ( #181549, #96077, #16901 ),
 ( #113439, #180500, #210854 ),
 ( #149055, #193549, #111306 ),
 ( #32117, #49433, #162130 ) ),
 .UNSPECIFIED., .F., .F., .T. ) 
 B_SPLINE_SURFACE_WITH_KNOTS ( ( 4, 4 ),
 ( 3, 3 ),
 ( 0.06089844177390838637, 0.06334004522945697879 ),
 ( 0.000000000000000000, 1.000000000000000000 ),
 .UNSPECIFIED. ) 
 GEOMETRIC_REPRESENTATION_ITEM ( )  RATIONAL_B_SPLINE_SURFACE ( (
 ( 1.000000000000000000, 0.7169884966214687960, 1.000000000000000000),
 ( 1.000000000000000000, 0.7174883642159475272, 1.000000000000000000),
 ( 1.000000000000000000, 0.7180610417775422638, 1.000000000000000000),
 ( 1.000000000000000000, 0.7187540717311187155, 1.000000000000000000) ) ) 
 REPRESENTATION_ITEM ( '' )  SURFACE ( )  );
#56186=VERTEX_POINT ( 'NONE', #162980 ) ;
#56201=SURFACE_STYLE_FILL_AREA ( #124488 ) ;
#56207=CARTESIAN_POINT ( 'NONE',  ( -0.04536344973642384565, -10.00000000000004796, -9.579592128873146706 ) ) ;
#56213=VERTEX_POINT ( 'NONE', #49226 ) ;
#56217=VECTOR ( 'NONE', #173740, 1000.000000000000000 ) ;
#56225=CARTESIAN_POINT ( 'NONE',  ( -0.04006801626467436372, -6.479296433800352695, 11.00029612940780410 ) ) ;
#56248=CARTESIAN_POINT ( 'NONE',  ( 0.000000000000000000, 15.50000000000019362, 0.000000000000000000 ) ) ;
#56274=CARTESIAN_POINT ( 'NONE',  ( 6.724721492623498165, -6.244189044378178011, 7.341412881700131621 ) ) ;
#56276=CARTESIAN_POINT ( 'NONE',  ( -3.239364772909965661E-16, -5.511313137147274333, -11.00000000000000178 ) ) ;
#56326=CARTESIAN_POINT ( 'NONE',  ( 1.255262969126037044E-15, -1.000000000000000888, -10.24999999999999822 ) ) ;
#56328=VECTOR ( 'NONE', #148632, 1000.000000000000000 ) ;
#56446=CARTESIAN_POINT ( 'NONE',  ( -7.769310276573702545, -5.221243112839676570, 7.769310276573728302 ) ) ;
#56447=CARTESIAN_POINT ( 'NONE',  ( 9.695354081530210166, -7.357813805514500594, 9.269928574751062911E-15 ) ) ;
#56480=EDGE_CURVE ( 'NONE', #29860, #156791, #18650, .T. ) ;
#56485=CARTESIAN_POINT ( 'NONE',  ( 0.4366904681730480742, -5.787668213791780758, 10.40319425600974235 ) ) ;
#56489=ORIENTED_EDGE ( 'NONE', *, *, #10791, .T. ) ;
#56503=CARTESIAN_POINT ( 'NONE',  ( 6.720112740279237329, -7.154544010627095219, -6.827626583076776612 ) ) ;
#56506=ADVANCED_FACE ( 'NONE', ( #3621 ), #200763, .F. ) ;
#56524=CARTESIAN_POINT ( 'NONE',  ( 6.558483974469879740, -6.776276029125230416, 6.864213375410075813 ) ) ;
#56525=CARTESIAN_POINT ( 'NONE',  ( -7.834948825496938163, -5.823938088759704534, -7.720982897393569466 ) ) ;
#56535=CARTESIAN_POINT ( 'NONE',  ( 0.4350687514514690046, -5.166862915010145052, 10.91132967064558024 ) ) ;
#56559=CARTESIAN_POINT ( 'NONE',  ( -0.06712503953322571104, -9.995102581657556939, -9.579544693637531694 ) ) ;
#56664=CARTESIAN_POINT ( 'NONE',  ( 6.937452841262716774, -7.242250812743806776, 6.937452841262695458 ) ) ;
#56733=CARTESIAN_POINT ( 'NONE',  ( -2.253107639696438902E-15, -7.721243112841103873, -10.98746396341378251 ) ) ;
#56747=AXIS2_PLACEMENT_3D ( 'NONE', #112620, #11834, #95262 ) ;
#56750=ORIENTED_EDGE ( 'NONE', *, *, #183643, .F. ) ;
#56751=ADVANCED_FACE ( 'NONE', ( #205038 ), #37223, .T. ) ;
#56783=CARTESIAN_POINT ( 'NONE',  ( -6.999862025036992286, -6.532648833121171172, 6.392587740394332307 ) ) ;
#56827=ORIENTED_EDGE ( 'NONE', *, *, #48815, .T. ) ;
#56845=SURFACE_STYLE_USAGE ( .BOTH. , #172742 ) ;
#56893=ADVANCED_FACE ( 'NONE', ( #57747 ), #162880, .T. ) ;
#56896=CARTESIAN_POINT ( 'NONE',  ( -0.08641082498352903318, -9.914243671626374876, -10.99966068378000728 ) ) ;
#56899=CARTESIAN_POINT ( 'NONE',  ( -11.00023875073173762, -5.574346042903139953, -0.04317804960739271558 ) ) ;
#56910=DIRECTION ( 'NONE',  ( 0.06086575749407437119, 0.9962285034897238045, -0.06183953750876716726 ) ) ;
#56998=DIRECTION ( 'NONE',  ( 0.000000000000000000, -1.000000000000000000, 0.000000000000000000 ) ) ;
#57000=AXIS2_PLACEMENT_3D ( 'NONE', #204789, #53238, #104131 ) ;
#57019=EDGE_CURVE ( 'NONE', #14247, #159583, #41832, .T. ) ;
#57039=DIRECTION ( 'NONE',  ( 0.000000000000000000, 0.000000000000000000, 1.000000000000000000 ) ) ;
#57048=AXIS2_PLACEMENT_3D ( 'NONE', #157325, #8917, #124896 ) ;
#57064=ORIENTED_EDGE ( 'NONE', *, *, #130804, .T. ) ;
#57102=ORIENTED_EDGE ( 'NONE', *, *, #35615, .T. ) ;
#57138=ADVANCED_FACE ( 'NONE', ( #198122 ), #168831, .T. ) ;
#57152=AXIS2_PLACEMENT_3D ( 'NONE', #14948, #36550, #34418 ) ;
#57185=CARTESIAN_POINT ( 'NONE',  ( 10.91804383151480096, -9.900000000000005684, -0.1905751639681742271 ) ) ;
#57186=( NAMED_UNIT ( * ) PLANE_ANGLE_UNIT ( ) SI_UNIT ( $, .RADIAN. ) );
#57268=CARTESIAN_POINT ( 'NONE',  ( 7.719547554928809951, -5.360178282914182191, 7.836475020641952227 ) ) ;
#57276=CYLINDRICAL_SURFACE ( 'NONE', #52658, 0.08000000000000020983 ) ;
#57282=ORIENTED_EDGE ( 'NONE', *, *, #104201, .F. ) ;
#57294=ORIENTED_EDGE ( 'NONE', *, *, #25109, .F. ) ;
#57299=CARTESIAN_POINT ( 'NONE',  ( -6.773846765307970585, -7.473374494058216300, 6.773846765307992790 ) ) ;
#57316=CARTESIAN_POINT ( 'NONE',  ( -7.055228938193937260, -8.176568542494910830, 6.396834479292722975 ) ) ;
#57325=LINE ( 'NONE', #24807, #209622 ) ;
#57338=DIRECTION ( 'NONE',  ( 0.000000000000000000, 0.000000000000000000, 1.000000000000000000 ) ) ;
#57339=CIRCLE ( 'NONE', #178422, 0.2000000000000005107 ) ;
#57340=CARTESIAN_POINT ( 'NONE',  ( 0.08058608058606736568, -5.770897281092849163, -10.99970480893079738 ) ) ;
#57347=LINE ( 'NONE', #107228, #34321 ) ;
#57348=LINE ( 'NONE', #76780, #198151 ) ;
#57362=CARTESIAN_POINT ( 'NONE',  ( -10.96785329849812562, -5.223431457505089526, 0.4373225248172959434 ) ) ;
#57378=CARTESIAN_POINT ( 'NONE',  ( -9.512045263456270661, -8.176568542494905500, 0.4655551865852137206 ) ) ;
#57389=CARTESIAN_POINT ( 'NONE',  ( 0.000000000000000000, -9.900000000000005684, 10.91970695577495931 ) ) ;
#57415=ADVANCED_FACE ( 'NONE', ( #189352 ), #180179, .T. ) ;
#57418=DIRECTION ( 'NONE',  ( 0.000000000000000000, -1.000000000000000000, 0.000000000000000000 ) ) ;
#57429=B_SPLINE_CURVE_WITH_KNOTS ( 'NONE', 3,
 ( #54867, #135068, #198946, #116714, #18067, #104695, #70011 ),
 .UNSPECIFIED., .F., .F.,
 ( 4, 3, 4 ),
 ( 3.314949680324280829E-05, 0.0009000000012044579497, 0.001958074173707490418 ),
 .UNSPECIFIED. ) ;
#57447=ORIENTED_EDGE ( 'NONE', *, *, #109647, .F. ) ;
#57471=CARTESIAN_POINT ( 'NONE',  ( -0.01387835396683118061, -7.030163990561719700, -9.597420367780069128 ) ) ;
#57501=CARTESIAN_POINT ( 'NONE',  ( 9.499766273075866962, -9.919999999999998153, -0.06663900456893058488 ) ) ;
#57515=CARTESIAN_POINT ( 'NONE',  ( 0.3313999689851374608, -9.006862915010144022, -9.494725171580505219 ) ) ;
#57527=AXIS2_PLACEMENT_3D ( 'NONE', #211867, #196702, #48342 ) ;
#57548=CARTESIAN_POINT ( 'NONE',  ( 0.000000000000000000, 3.956598013261175772, 0.000000000000000000 ) ) ;
#57552=CARTESIAN_POINT ( 'NONE',  ( 9.495347311156807635, -6.857257212219900921, -1.861063089699362494E-15 ) ) ;
#57560=DIRECTION ( 'NONE',  ( 0.6783731810844091381, 3.929830605827845711E-15, 0.7347175152297782397 ) ) ;
#57570=CARTESIAN_POINT ( 'NONE',  ( -10.99947830037066865, -9.912501460265211506, 0.1071380031274376810 ) ) ;
#57571=CARTESIAN_POINT ( 'NONE',  ( 0.000000000000000000, -9.919999999999998153, 0.000000000000000000 ) ) ;
#57623=CARTESIAN_POINT ( 'NONE',  ( 6.773846765317306229, -7.246166700180828535, -6.773846765317331986 ) ) ;
#57668=B_SPLINE_CURVE_WITH_KNOTS ( 'NONE', 3,
 ( #194126, #31646, #130284, #213551, #197323, #32695, #163781, #147530, #80384, #13246 ),
 .UNSPECIFIED., .F., .F.,
 ( 4, 2, 2, 2, 4 ),
 ( 0.000000000000000000, 0.0002299353307164137407, 0.0004598706614328274813, 0.0006898059921492411678, 0.0009197413228656549627 ),
 .UNSPECIFIED. ) ;
#57699=VERTEX_POINT ( 'NONE', #113509 ) ;
#57739=DIRECTION ( 'NONE',  ( 0.000000000000000000, 1.000000000000000000, 0.000000000000000000 ) ) ;
#57747=FACE_OUTER_BOUND ( 'NONE', #35768, .T. ) ;
#57793=CARTESIAN_POINT ( 'NONE',  ( 10.99962150373186809, -9.919999999999998153, -0.09125116240079202135 ) ) ;
#57796=CIRCLE ( 'NONE', #130546, 0.07999999999999982125 ) ;
#57805=CARTESIAN_POINT ( 'NONE',  ( -0.3107038660269380026, -6.804704122739850369, -10.86205067566995375 ) ) ;
#57813=VECTOR ( 'NONE', #17365, 1000.000000000000000 ) ;
#57835=CARTESIAN_POINT ( 'NONE',  ( 7.681496476274699781, -5.295524846228401472, 7.873959529867727625 ) ) ;
#57847=CARTESIAN_POINT ( 'NONE',  ( 0.1589091098076318986, -6.723650695528626819, 9.611540586923185359 ) ) ;
#57885=DIRECTION ( 'NONE',  ( 1.000000000000000000, 0.000000000000000000, 0.000000000000000000 ) ) ;
#57915=ADVANCED_FACE ( 'NONE', ( #165378 ), #115094, .T. ) ;
#58040=CARTESIAN_POINT ( 'NONE',  ( -6.663994888585885512, -7.154544010627095219, 6.770610912236877610 ) ) ;
#58047=FACE_OUTER_BOUND ( 'NONE', #193438, .T. ) ;
#58049=CONICAL_SURFACE ( 'NONE', #92711, 10.99999999999999112, 0.7853981633974425058 ) ;
#58061=DIRECTION ( 'NONE',  ( 0.000000000000000000, 0.000000000000000000, -1.000000000000000000 ) ) ;
#58064=CIRCLE ( 'NONE', #33934, 0.08000000000000050127 ) ;
#58068=( LENGTH_UNIT ( ) NAMED_UNIT ( * ) SI_UNIT ( .MILLI., .METRE. ) );
#58091=ORIENTED_EDGE ( 'NONE', *, *, #186328, .F. ) ;
#58093=CARTESIAN_POINT ( 'NONE',  ( -0.3793797362570683895, -6.699757570937928008, -10.99387514841215641 ) ) ;
#58108=CARTESIAN_POINT ( 'NONE',  ( -9.532262708098283355, -8.048696291100942091, 0.1899713450103325540 ) ) ;
#58109=CARTESIAN_POINT ( 'NONE',  ( -0.1132184859782652403, 3.829867255648767621, 11.66962136008045192 ) ) ;
#58134=CARTESIAN_POINT ( 'NONE',  ( 9.513083153069256781, -8.198316282515564879, 9.269928574751062911E-15 ) ) ;
#58157=VERTEX_POINT ( 'NONE', #61645 ) ;
#58158=CIRCLE ( 'NONE', #85832, 6.249999999999995559 ) ;
#58233=CARTESIAN_POINT ( 'NONE',  ( 1.355252715606880543E-15, 4.021557182957056220, -11.93179687198411543 ) ) ;
#58252=( NAMED_UNIT ( * ) SI_UNIT ( $, .STERADIAN. ) SOLID_ANGLE_UNIT ( ) );
#58281=CARTESIAN_POINT ( 'NONE',  ( 0.08058608058606961388, -9.999999999999994671, -10.99970480893079738 ) ) ;
#58321=CARTESIAN_POINT ( 'NONE',  ( -2.494447209962484813, 3.467171072964057466, 11.73545145049398464 ) ) ;
#58331=CARTESIAN_POINT ( 'NONE',  ( 7.828177403543859825, -5.742104877864243839, 7.727873494160014900 ) ) ;
#58338=DIRECTION ( 'NONE',  ( 0.000000000000000000, 1.000000000000000000, 0.000000000000000000 ) ) ;
#58363=CARTESIAN_POINT ( 'NONE',  ( 0.07406709734308211668, -9.431556885384749123, -9.500634193481465317 ) ) ;
#58364=CARTESIAN_POINT ( 'NONE',  ( 10.39230484541330313, 4.000000000000003553, 5.999999999999906741 ) ) ;
#58379=ADVANCED_FACE ( 'NONE', ( #16064 ), #160213, .T. ) ;
#58381=CARTESIAN_POINT ( 'NONE',  ( -6.779954559072826292, -7.792646766725027874, 6.731761806397297931 ) ) ;
#58404=CARTESIAN_POINT ( 'NONE',  ( 0.1945363205450193478, 1.000000000000000888, -11.93115981699675743 ) ) ;
#58419=( NAMED_UNIT ( * ) SI_UNIT ( $, .STERADIAN. ) SOLID_ANGLE_UNIT ( ) );
#58422=ORIENTED_EDGE ( 'NONE', *, *, #158609, .T. ) ;
#58464=DIRECTION ( 'NONE',  ( 0.000000000000000000, 0.000000000000000000, 1.000000000000000000 ) ) ;
#58467=CARTESIAN_POINT ( 'NONE',  ( 10.91804383151480096, 0.000000000000000000, -0.1905751639681742271 ) ) ;
#58472=CARTESIAN_POINT ( 'NONE',  ( -0.2977236940312470992, -5.250949308401958504, -10.97067990664317350 ) ) ;
#58579=CARTESIAN_POINT ( 'NONE',  ( 7.214015694909405418, -7.024005795613374126, 7.869907041763756439 ) ) ;
#58580=ORIENTED_EDGE ( 'NONE', *, *, #35599, .F. ) ;
#58588=CARTESIAN_POINT ( 'NONE',  ( 0.000000000000000000, -6.836568542494925182, 0.000000000000000000 ) ) ;
#58594=CARTESIAN_POINT ( 'NONE',  ( 0.3636750363432239008, -6.893137084989843899, 10.99449589488468604 ) ) ;
#58602=MECHANICAL_DESIGN_GEOMETRIC_PRESENTATION_REPRESENTATION('',(#34312),#155378);
#58624=EDGE_CURVE ( 'NONE', #149119, #87461, #108869, .T. ) ;
#58633=CARTESIAN_POINT ( 'NONE',  ( -1.734723475976807094E-15, -8.327195405469542067, -10.91970695577494332 ) ) ;
#58658=CARTESIAN_POINT ( 'NONE',  ( 10.89423718502886906, -6.453216945989374231, -0.03415196713897916680 ) ) ;
#58685=CARTESIAN_POINT ( 'NONE',  ( -7.499070966595134280, -5.223177556212268868, -8.016215341155858098 ) ) ;
#58702=B_SPLINE_CURVE_WITH_KNOTS ( 'NONE', 3,
 ( #94139, #143975, #26961, #7506, #188403, #155923, #8585 ),
 .UNSPECIFIED., .F., .F.,
 ( 4, 3, 4 ),
 ( 0.0001932309589017161869, 0.0009000000022123051842, 0.002089081127711812057 ),
 .UNSPECIFIED. ) ;
#58730=EDGE_LOOP ( 'NONE', ( #55048, #17160, #111855, #113806 ) ) ;
#58775=ADVANCED_FACE ( 'NONE', ( #191538 ), #205661, .F. ) ;
#58795=VERTEX_POINT ( 'NONE', #113325 ) ;
#58811=DIRECTION ( 'NONE',  ( 0.000000000000000000, 0.000000000000000000, -1.000000000000000000 ) ) ;
#58812=VERTEX_POINT ( 'NONE', #30953 ) ;
#58845=B_SPLINE_CURVE_WITH_KNOTS ( 'NONE', 3,
 ( #19987, #167331, #169453, #151093, #138038, #88211, #69792, #67650 ),
 .UNSPECIFIED., .F., .F.,
 ( 4, 2, 2, 4 ),
 ( 1.064029803361153984E-15, 0.0004636157603174426438, 0.0006954236404756319748, 0.0009272315206338212516 ),
 .UNSPECIFIED. ) ;
#58848=CARTESIAN_POINT ( 'NONE',  ( -10.91962425643199808, -9.919999999999998153, 0.09058751758333691284 ) ) ;
#58859=CARTESIAN_POINT ( 'NONE',  ( 6.830415307812257808, -7.473374494058229622, 6.717278222822394618 ) ) ;
#58862=B_SPLINE_CURVE_WITH_KNOTS ( 'NONE', 3,
 ( #57362, #174334, #25912, #172189, #107244, #121377, #21616, #59486 ),
 .UNSPECIFIED., .F., .F.,
 ( 4, 2, 2, 4 ),
 ( 7.521151966117911075E-18, 0.0002224730689913869807, 0.0004449461379827664804, 0.0008898922759655229862 ),
 .UNSPECIFIED. ) ;
#58927=CARTESIAN_POINT ( 'NONE',  ( 0.08097581798159399213, -9.904508987438854106, 10.99970197202149969 ) ) ;
#58954=B_SPLINE_CURVE_WITH_KNOTS ( 'NONE', 3,
 ( #161999, #94871, #29861, #114370, #112238, #28788, #146827 ),
 .UNSPECIFIED., .F., .F.,
 ( 4, 3, 4 ),
 ( 0.000000000000000000, 0.0008000000000005096134, 0.002977368225425562967 ),
 .UNSPECIFIED. ) ;
#58978=CARTESIAN_POINT ( 'NONE',  ( -2.044581833100346469, 2.972657967446783456, 11.47952151275213240 ) ) ;
#58992=DIRECTION ( 'NONE',  ( 0.000000000000000000, 0.000000000000000000, 1.000000000000000000 ) ) ;
#59026=CARTESIAN_POINT ( 'NONE',  ( -0.08246874231332826377, -9.908734156519553693, -10.99969088041219401 ) ) ;
#59035=DIRECTION ( 'NONE',  ( 0.000000000000000000, 1.000000000000000000, 0.000000000000000000 ) ) ;
#59054=AXIS2_PLACEMENT_3D ( 'NONE', #13612, #48281, #98096 ) ;
#59059=CARTESIAN_POINT ( 'NONE',  ( -9.499606442108964544, -9.900000000000005684, 0.08647222121513538362 ) ) ;
#59060=CARTESIAN_POINT ( 'NONE',  ( 0.000000000000000000, 0.000000000000000000, 0.000000000000000000 ) ) ;
#59114=ORIENTED_EDGE ( 'NONE', *, *, #166016, .F. ) ;
#59121=ORIENTED_EDGE ( 'NONE', *, *, #13614, .T. ) ;
#59158=ADVANCED_FACE ( 'NONE', ( #124517 ), #54297, .T. ) ;
#59169=AXIS2_PLACEMENT_3D ( 'NONE', #138947, #55544, #76059 ) ;
#59179=B_SPLINE_CURVE_WITH_KNOTS ( 'NONE', 3,
 ( #5592, #105291, #122684, #188647, #75969, #157235, #159349, #172411, #92255, #192899 ),
 .UNSPECIFIED., .F., .F.,
 ( 4, 2, 2, 2, 4 ),
 ( 5.529431079675726716E-18, 0.0002236660844579351078, 0.0004473321689158646862, 0.0006709982533737942918, 0.0008946643378317238431 ),
 .UNSPECIFIED. ) ;
#59188=ORIENTED_EDGE ( 'NONE', *, *, #119616, .F. ) ;
#59213=ORIENTED_EDGE ( 'NONE', *, *, #64826, .T. ) ;
#59222=CARTESIAN_POINT ( 'NONE',  ( 0.000000000000000000, -9.911192131523236526, 10.91970695577495931 ) ) ;
#59281=( BOUNDED_SURFACE ( )  B_SPLINE_SURFACE ( 3, 2, ( 
 ( #25533, #92701, #158747 ),
 ( #93767, #208534, #202 ),
 ( #147576, #64189, #163829 ),
 ( #115128, #181123, #60170 ),
 ( #132420, #91641, #157694 ),
 ( #207483, #43946, #80431 ),
 ( #146531, #130330, #196319 ),
 ( #15407, #81498, #99881 ) ),
 .UNSPECIFIED., .F., .F., .T. ) 
 B_SPLINE_SURFACE_WITH_KNOTS ( ( 4, 2, 2, 4 ),
 ( 3, 3 ),
 ( 5.963111948670274387E-19, 0.0002475938981900011613, 0.0004951877963800016720, 0.0009903755927600026935 ),
 ( 0.000000000000000000, 1.000000000000000000 ),
 .UNSPECIFIED. ) 
 GEOMETRIC_REPRESENTATION_ITEM ( )  RATIONAL_B_SPLINE_SURFACE ( (
 ( 1.000000000000000000, 0.9238795325112872936, 1.000000000000000000),
 ( 1.000000000000000000, 0.9248499699753846004, 1.000000000000000000),
 ( 1.000000000000000000, 0.9171047238582999972, 1.000000000000000000),
 ( 1.000000000000000000, 0.8907236462369912955, 1.000000000000000000),
 ( 1.000000000000000000, 0.8725411758594774358, 1.000000000000000000),
 ( 1.000000000000000000, 0.8105159241142789739, 1.000000000000000000),
 ( 1.000000000000000000, 0.7599483315140537210, 1.000000000000000000),
 ( 1.000000000000000000, 0.7045118851637761637, 1.000000000000000000) ) ) 
 REPRESENTATION_ITEM ( '' )  SURFACE ( )  );
#59293=ORIENTED_EDGE ( 'NONE', *, *, #45047, .F. ) ;
#59298=( BOUNDED_SURFACE ( )  B_SPLINE_SURFACE ( 3, 2, ( 
 ( #162172, #178421, #157912 ),
 ( #177350, #127622, #175231 ),
 ( #206629, #27892, #12686 ),
 ( #9507, #75579, #43106 ) ),
 .UNSPECIFIED., .F., .F., .F. ) 
 B_SPLINE_SURFACE_WITH_KNOTS ( ( 4, 4 ),
 ( 3, 3 ),
 ( 0.01126995942960227343, 0.01373815140602661217 ),
 ( 0.000000000000000000, 1.000000000000000000 ),
 .UNSPECIFIED. ) 
 GEOMETRIC_REPRESENTATION_ITEM ( )  RATIONAL_B_SPLINE_SURFACE ( (
 ( 1.000000000000000000, 0.6947640035331654751, 1.000000000000000000),
 ( 1.000000000000000000, 0.6955505939616328792, 1.000000000000000000),
 ( 1.000000000000000000, 0.6961913616428423435, 1.000000000000000000),
 ( 1.000000000000000000, 0.6967468848049983565, 1.000000000000000000) ) ) 
 REPRESENTATION_ITEM ( '' )  SURFACE ( )  );
#59299=CARTESIAN_POINT ( 'NONE',  ( 9.093502852636627054, 1.000000000000000888, 7.666967846417570343 ) ) ;
#59309=CARTESIAN_POINT ( 'NONE',  ( 10.91944941500665855, -9.999999999999994671, -0.1017788107271373199 ) ) ;
#59315=( BOUNDED_SURFACE ( )  B_SPLINE_SURFACE ( 3, 2, ( 
 ( #113569, #194740, #77795 ),
 ( #14902, #97266, #142839 ),
 ( #112496, #46377, #143914 ),
 ( #125572, #95138, #212037 ),
 ( #60475, #177439, #209909 ),
 ( #13843, #178506, #163322 ),
 ( #61546, #162257, #141780 ),
 ( #126633, #191533, #193673 ) ),
 .UNSPECIFIED., .F., .F., .F. ) 
 B_SPLINE_SURFACE_WITH_KNOTS ( ( 4, 2, 2, 4 ),
 ( 3, 3 ),
 ( 5.421010862427522170E-20, 0.0005123566476021758223, 0.0007685349714032637877, 0.001024713295204351645 ),
 ( 0.000000000000000000, 1.000000000000000000 ),
 .UNSPECIFIED. ) 
 GEOMETRIC_REPRESENTATION_ITEM ( )  RATIONAL_B_SPLINE_SURFACE ( (
 ( 1.000000000000000000, 0.7100530722026823227, 1.000000000000000000),
 ( 1.000000000000000000, 0.7667719522827172174, 1.000000000000000000),
 ( 1.000000000000000000, 0.8160440554223276077, 1.000000000000000000),
 ( 1.000000000000000000, 0.8737249316769536422, 1.000000000000000000),
 ( 1.000000000000000000, 0.8903164784319999026, 1.000000000000000000),
 ( 1.000000000000000000, 0.9150853305241253288, 1.000000000000000000),
 ( 1.000000000000000000, 0.9227739504732664910, 1.000000000000000000),
 ( 1.000000000000000000, 0.9238795325112855172, 1.000000000000000000) ) ) 
 REPRESENTATION_ITEM ( '' )  SURFACE ( )  );
#59316=CARTESIAN_POINT ( 'NONE',  ( -10.58872653680447939, -6.465328379374283507, 1.138412281109779656E-15 ) ) ;
#59322=CARTESIAN_POINT ( 'NONE',  ( -11.37385970535894231, 1.000000000000000888, 3.825613075418397457 ) ) ;
#59332=EDGE_CURVE ( 'NONE', #206986, #166319, #74621, .T. ) ;
#59335=AXIS2_PLACEMENT_3D ( 'NONE', #23111, #70790, #5783 ) ;
#59352=CARTESIAN_POINT ( 'NONE',  ( -0.1645940602202590475, -7.825441678136469292, 10.99897937609845044 ) ) ;
#59377=CIRCLE ( 'NONE', #90478, 11.54340198673881979 ) ;
#59385=DIRECTION ( 'NONE',  ( 0.000000000000000000, 1.000000000000000000, 0.000000000000000000 ) ) ;
#59390=ADVANCED_FACE ( 'NONE', ( #165190 ), #187278, .T. ) ;
#59392=CARTESIAN_POINT ( 'NONE',  ( 7.523999700038789484, -5.166862915010145052, 8.024744567526242989 ) ) ;
#59398=DIRECTION ( 'NONE',  ( 0.000000000000000000, 0.000000000000000000, 1.000000000000000000 ) ) ;
#59420=CARTESIAN_POINT ( 'NONE',  ( 0.07995206772519822258, -9.200995477224008567, -9.499751636909056884 ) ) ;
#59422=DIRECTION ( 'NONE',  ( 0.000000000000000000, -1.000000000000000000, 0.000000000000000000 ) ) ;
#59440=CARTESIAN_POINT ( 'NONE',  ( -6.808607288253732293, -8.010031549403114681, 6.625366561259686371 ) ) ;
#59486=CARTESIAN_POINT ( 'NONE',  ( -10.91970695577496997, -5.907420853759282053, 5.204170427930421283E-15 ) ) ;
#59526=CARTESIAN_POINT ( 'NONE',  ( 0.04341786867403699124, -5.575210796978269379, -11.00023563321887643 ) ) ;
#59527=ORIENTED_EDGE ( 'NONE', *, *, #90996, .F. ) ;
#59579=EDGE_CURVE ( 'NONE', #58812, #80737, #38571, .T. ) ;
#59582=FACE_OUTER_BOUND ( 'NONE', #191759, .T. ) ;
#59589=CARTESIAN_POINT ( 'NONE',  ( 10.38819714233658686, 3.487142912321096855, -5.997628416523089534 ) ) ;
#59635=CARTESIAN_POINT ( 'NONE',  ( -7.580882385731715800, -6.105993949506102858, 7.580882385731741557 ) ) ;
#59636=CARTESIAN_POINT ( 'NONE',  ( 0.03866526371284223496, -9.261493551422342208, -9.500000000000152767 ) ) ;
#59647=FACE_OUTER_BOUND ( 'NONE', #78633, .T. ) ;
#59670=CARTESIAN_POINT ( 'NONE',  ( 7.346809171966843799, -6.836568542494916301, 8.002408263929979171 ) ) ;
#59681=CARTESIAN_POINT ( 'NONE',  ( -10.99574878476023976, -7.889012432655405860, 0.3098035853330368128 ) ) ;
#59689=CARTESIAN_POINT ( 'NONE',  ( 0.07999999999999327094, -9.999999999999994671, 10.99970695577496294 ) ) ;
#59720=FACE_OUTER_BOUND ( 'NONE', #45976, .T. ) ;
#59723=CARTESIAN_POINT ( 'NONE',  ( 7.721398836998401904, -6.134628647623499909, 7.721398836998376147 ) ) ;
#59775=ADVANCED_FACE ( 'NONE', ( #138037 ), #204050, .T. ) ;
#59880=AXIS2_PLACEMENT_3D ( 'NONE', #25007, #142006, #110607 ) ;
#59942=B_SPLINE_CURVE_WITH_KNOTS ( 'NONE', 3,
 ( #181314, #5468, #169067, #16665 ),
 .UNSPECIFIED., .F., .F.,
 ( 4, 4 ),
 ( 1.083473084032624673E-15, 8.505390839925406612E-05 ),
 .UNSPECIFIED. ) ;
#59944=EDGE_LOOP ( 'NONE', ( #60880, #207493, #176440, #157755, #73241 ) ) ;
#59963=CARTESIAN_POINT ( 'NONE',  ( 6.956254272497339741, -6.713678229395078745, -6.457408393014691050 ) ) ;
#59969=DIRECTION ( 'NONE',  ( 1.000000000000000000, -0.000000000000000000, 1.224646799147353207E-16 ) ) ;
#60019=( GEOMETRIC_REPRESENTATION_CONTEXT ( 3 ) GLOBAL_UNCERTAINTY_ASSIGNED_CONTEXT ( ( #210303 ) ) GLOBAL_UNIT_ASSIGNED_CONTEXT ( ( #71987, #184678, #200914 ) ) REPRESENTATION_CONTEXT ( 'NONE', 'WORKASPACE' ) );
#60029=VERTEX_POINT ( 'NONE', #97410 ) ;
#60043=PRESENTATION_STYLE_ASSIGNMENT (( #56845 ) ) ;
#60148=EDGE_CURVE ( 'NONE', #144331, #186972, #152653, .T. ) ;
#60170=CARTESIAN_POINT ( 'NONE',  ( 0.1833053738655651410, -5.341077028191773657, 10.96562622554680821 ) ) ;
#60187=ORIENTED_EDGE ( 'NONE', *, *, #176622, .F. ) ;
#60210=ORIENTED_EDGE ( 'NONE', *, *, #129019, .T. ) ;
#60219=EDGE_LOOP ( 'NONE', ( #125900, #13078, #16346, #55754 ) ) ;
#60221=CARTESIAN_POINT ( 'NONE',  ( -1.020505294851981049E-14, -6.134628647623514119, -10.91970695577493977 ) ) ;
#60250=EDGE_CURVE ( 'NONE', #27864, #189856, #136794, .T. ) ;
#60267=CARTESIAN_POINT ( 'NONE',  ( -8.923337013803626760, 2.630042260599928294, -8.023366178422991268 ) ) ;
#60293=ORIENTED_EDGE ( 'NONE', *, *, #27811, .T. ) ;
#60382=CARTESIAN_POINT ( 'NONE',  ( -6.758184431511294221, -6.900108348305955097, -6.825879202496253129 ) ) ;
#60442=COLOUR_RGB ( '', 0.08235294, 0.09019608, 0.10196078) ;
#60475=CARTESIAN_POINT ( 'NONE',  ( 9.531438498077132948, -8.057097448493882652, -0.1980946632348720704 ) ) ;
#60535=ADVANCED_FACE ( 'NONE', ( #149339 ), #66986, .T. ) ;
#60541=COLOUR_RGB ( '', 0.09019608, 0.27058824, 0.51372549) ;
#60583=CARTESIAN_POINT ( 'NONE',  ( 7.876942567271134621, -5.350481869465718354, -7.629869294364563181 ) ) ;
#60584=PRESENTATION_STYLE_ASSIGNMENT (( #194852 ) ) ;
#60594=CARTESIAN_POINT ( 'NONE',  ( -0.1178541238725513418, -5.389012432655349016, -10.99948089704805199 ) ) ;
#60609=PRESENTATION_STYLE_ASSIGNMENT (( #28114 ) ) ;
#60622=CARTESIAN_POINT ( 'NONE',  ( 0.1520312049661921572, -8.104757123234346494, 9.499050059654537748 ) ) ;
#60677=CARTESIAN_POINT ( 'NONE',  ( 0.000000000000000000, 4.000000000000003553, 0.000000000000000000 ) ) ;
#60680=CARTESIAN_POINT ( 'NONE',  ( -6.511381374296909996, -8.144978210217297843, -6.953912913643677030 ) ) ;
#60692=VERTEX_POINT ( 'NONE', #12092 ) ;
#60701=CARTESIAN_POINT ( 'NONE',  ( 6.801849727211993546, -7.605490242344523644, 7.458876343102490480 ) ) ;
#60732=CARTESIAN_POINT ( 'NONE',  ( 0.04698948850440434755, -9.984793193541563028, 9.579582872750577849 ) ) ;
#60733=CARTESIAN_POINT ( 'NONE',  ( 6.932145363377535396, -8.169775483750580491, -6.496114076516128932 ) ) ;
#60739=AXIS2_PLACEMENT_3D ( 'NONE', #94617, #210459, #74073 ) ;
#60747=SURFACE_STYLE_FILL_AREA ( #210183 ) ;
#60754=CYLINDRICAL_SURFACE ( 'NONE', #181795, 0.08000000000000020983 ) ;
#60813=CARTESIAN_POINT ( 'NONE',  ( -7.834948825496938163, -5.907420853759296264, -7.720982897393567690 ) ) ;
#60818=EDGE_CURVE ( 'NONE', #104249, #50012, #620, .T. ) ;
#60823=DIRECTION ( 'NONE',  ( 1.000000000000000000, 0.000000000000000000, -1.224646799147353207E-16 ) ) ;
#60853=CARTESIAN_POINT ( 'NONE',  ( 0.000000000000000000, 3.000000000000002665, 0.000000000000000000 ) ) ;
#60858=TOROIDAL_SURFACE ( 'NONE', #116269, 6.330000000000000959, 0.08000000000000000167 ) ;
#60870=CARTESIAN_POINT ( 'NONE',  ( 0.000000000000000000, -7.246166700194011767, 9.579665964935665912 ) ) ;
#60880=ORIENTED_EDGE ( 'NONE', *, *, #13865, .F. ) ;
#60903=CARTESIAN_POINT ( 'NONE',  ( -10.99976498415366954, -5.359187537802505119, 0.08336379702154585181 ) ) ;
#60922=AXIS2_PLACEMENT_3D ( 'NONE', #87947, #187569, #141011 ) ;
#60932=ORIENTED_EDGE ( 'NONE', *, *, #196420, .F. ) ;
#60951=FACE_OUTER_BOUND ( 'NONE', #7194, .T. ) ;
#60974=CARTESIAN_POINT ( 'NONE',  ( 7.446209719563365859, -5.223431457505076203, 8.064677165291195493 ) ) ;
#60985=( GEOMETRIC_REPRESENTATION_CONTEXT ( 3 ) GLOBAL_UNCERTAINTY_ASSIGNED_CONTEXT ( ( #127554 ) ) GLOBAL_UNIT_ASSIGNED_CONTEXT ( ( #74308, #157701, #205349 ) ) REPRESENTATION_CONTEXT ( 'NONE', 'WORKASPACE' ) );
#61042=CARTESIAN_POINT ( 'NONE',  ( -10.99943592164172834, -9.900000000000005684, 0.1113975120798846308 ) ) ;
#61051=CIRCLE ( 'NONE', #88742, 0.08000000000000009881 ) ;
#61056=CARTESIAN_POINT ( 'NONE',  ( 7.580882385732278905, -6.105993949506924423, -7.580882385732309103 ) ) ;
#61146=DIRECTION ( 'NONE',  ( 0.000000000000000000, 1.000000000000000000, 0.000000000000000000 ) ) ;
#61200=AXIS2_PLACEMENT_3D ( 'NONE', #54893, #72183, #118882 ) ;
#61262=CARTESIAN_POINT ( 'NONE',  ( 4.806723615010448736E-13, -7.868798029037617603, -9.500000000000001776 ) ) ;
#61276=DIRECTION ( 'NONE',  ( 0.000000000000000000, 0.000000000000000000, 1.000000000000000000 ) ) ;
#61287=CYLINDRICAL_SURFACE ( 'NONE', #182116, 0.08000000000000020983 ) ;
#61295=CARTESIAN_POINT ( 'NONE',  ( 0.08058605610391310348, -6.304485801116100241, -10.99970480911016146 ) ) ;
#61298=DIRECTION ( 'NONE',  ( 0.000000000000000000, -1.000000000000000000, 0.000000000000000000 ) ) ;
#61321=CARTESIAN_POINT ( 'NONE',  ( -2.331034670843834533E-15, -7.357813805514510364, 9.695354081530208390 ) ) ;
#61340=CARTESIAN_POINT ( 'NONE',  ( -10.64229060209982514, 1.016282880930358568, -6.144329343916520081 ) ) ;
#61393=CARTESIAN_POINT ( 'NONE',  ( 6.766604819867146681, -7.256397064628574256, 6.766604819867123588 ) ) ;
#61424=B_SPLINE_CURVE_WITH_KNOTS ( 'NONE', 3,
 ( #4615, #103227, #1422, #102156 ),
 .UNSPECIFIED., .F., .F.,
 ( 4, 4 ),
 ( 0.000000000000000000, 0.0002909236271752678894 ),
 .UNSPECIFIED. ) ;
#61430=ORIENTED_EDGE ( 'NONE', *, *, #190504, .T. ) ;
#61463=CARTESIAN_POINT ( 'NONE',  ( -0.07933194154488912297, -7.473374494045017968, 9.499668754385634628 ) ) ;
#61475=CARTESIAN_POINT ( 'NONE',  ( -10.39230484541323740, 3.499999999999989342, 6.000000000000048850 ) ) ;
#61484=CARTESIAN_POINT ( 'NONE',  ( -9.483599735403307918, -9.201296717416616033, 0.5591315121169729840 ) ) ;
#61507=AXIS2_PLACEMENT_3D ( 'NONE', #111697, #108499, #44516 ) ;
#61535=ORIENTED_EDGE ( 'NONE', *, *, #60818, .T. ) ;
#61546=CARTESIAN_POINT ( 'NONE',  ( 9.516020521606803229, -8.176244038172738371, -0.3909723190920387226 ) ) ;
#61573=CARTESIAN_POINT ( 'NONE',  ( -6.825099317097829577, -8.105676417795773858, 6.608557002163587768 ) ) ;
#61589=VERTEX_POINT ( 'NONE', #159156 ) ;
#61611=DIRECTION ( 'NONE',  ( -1.084202172485362439E-14, -1.000000000000000000, -3.260636891504970529E-14 ) ) ;
#61614=ORIENTED_EDGE ( 'NONE', *, *, #169387, .T. ) ;
#61645=CARTESIAN_POINT ( 'NONE',  ( 0.000000000000000000, 3.499999999999989342, 12.00000000000000178 ) ) ;
#61652=ORIENTED_EDGE ( 'NONE', *, *, #171517, .T. ) ;
#61656=CARTESIAN_POINT ( 'NONE',  ( 7.787098537122153274, -5.543994141378499663, -7.698131257602417676 ) ) ;
#61657=DIRECTION ( 'NONE',  ( 0.000000000000000000, 0.000000000000000000, 1.000000000000000000 ) ) ;
#61682=( NAMED_UNIT ( * ) SI_UNIT ( $, .STERADIAN. ) SOLID_ANGLE_UNIT ( ) );
#61689=CARTESIAN_POINT ( 'NONE',  ( -10.91944002402978775, -9.999999999999994671, 0.1105873483556694958 ) ) ;
#61711=EDGE_LOOP ( 'NONE', ( #185570, #164276, #139244, #77497 ) ) ;
#61717=CIRCLE ( 'NONE', #137950, 11.49999999999998934 ) ;
#61721=CARTESIAN_POINT ( 'NONE',  ( 2.168404344971008868E-16, -7.246166700193014343, -9.579665964947887247 ) ) ;
#61780=CARTESIAN_POINT ( 'NONE',  ( 0.000000000000000000, 3.499999999999989342, 0.000000000000000000 ) ) ;
#61808=CARTESIAN_POINT ( 'NONE',  ( 7.710100441483561440, -6.699703214240864568, 7.845789747616994880 ) ) ;
#61809=STYLED_ITEM ( 'NONE', ( #22521 ), #22111 ) ;
#61823=( NAMED_UNIT ( * ) SI_UNIT ( $, .STERADIAN. ) SOLID_ANGLE_UNIT ( ) );
#61861=( BOUNDED_SURFACE ( )  B_SPLINE_SURFACE ( 3, 2, ( 
 ( #10395, #76470, #60221 ),
 ( #61295, #176128, #142579 ),
 ( #124254, #208586, #126380 ),
 ( #192339, #11465, #27727 ),
 ( #207536, #74351, #42938 ),
 ( #93821, #58093, #12531 ),
 ( #78603, #159862, #127456 ),
 ( #177184, #45071, #9342 ) ),
 .UNSPECIFIED., .F., .F., .F. ) 
 B_SPLINE_SURFACE_WITH_KNOTS ( ( 4, 2, 2, 4 ),
 ( 3, 3 ),
 ( 0.000000000000000000, 0.0005109843281227174992, 0.0007664764921840762487, 0.001021968656245434998 ),
 ( 0.000000000000000000, 1.000000000000000000 ),
 .UNSPECIFIED. ) 
 GEOMETRIC_REPRESENTATION_ITEM ( )  RATIONAL_B_SPLINE_SURFACE ( (
 ( 1.000000000000000000, 0.7045118851637612867, 1.000000000000000000),
 ( 1.000000000000000000, 0.6478559580219772629, 1.000000000000000000),
 ( 1.000000000000000000, 0.5832506164449779984, 1.000000000000000000),
 ( 1.000000000000000000, 0.4879709628488522188, 1.000000000000000000),
 ( 1.000000000000000000, 0.4561823831824661224, 1.000000000000000000),
 ( 1.000000000000000000, 0.4039565156457392558, 1.000000000000000000),
 ( 1.000000000000000000, 0.3848936348729107282, 1.000000000000000000),
 ( 1.000000000000000000, 0.3826834323650832315, 1.000000000000000000) ) ) 
 REPRESENTATION_ITEM ( '' )  SURFACE ( )  );
#61920=CARTESIAN_POINT ( 'NONE',  ( 6.588752024304575627, -8.074889850123490476, 6.844216539294094126 ) ) ;
#61953=ORIENTED_EDGE ( 'NONE', *, *, #89270, .T. ) ;
#61968=ORIENTED_EDGE ( 'NONE', *, *, #64072, .F. ) ;
#62007=ORIENTED_EDGE ( 'NONE', *, *, #63875, .T. ) ;
#62014=DIRECTION ( 'NONE',  ( 0.9989735196462988798, 0.000000000000000000, -0.04529798058948708572 ) ) ;
#62018=ADVANCED_FACE ( 'NONE', ( #48621 ), #170268, .F. ) ;
#62055=ORIENTED_EDGE ( 'NONE', *, *, #23354, .T. ) ;
#62078=CYLINDRICAL_SURFACE ( 'NONE', #146576, 0.07999999999999993228 ) ;
#62114=CARTESIAN_POINT ( 'NONE',  ( -9.586610838029429260, -7.161464053357567749, 0.003376046620574604893 ) ) ;
#62137=DIRECTION ( 'NONE',  ( -2.168462536859579677E-14, -1.000000000000000000, -9.418999208338882750E-28 ) ) ;
#62142=DIRECTION ( 'NONE',  ( 0.000000000000000000, 0.000000000000000000, 1.000000000000000000 ) ) ;
#62178=CIRCLE ( 'NONE', #110643, 0.08000000000000001554 ) ;
#62261=SURFACE_STYLE_USAGE ( .BOTH. , #47100 ) ;
#62263=VECTOR ( 'NONE', #161126, 1000.000000000000000 ) ;
#62269=LINE ( 'NONE', #147798, #51152 ) ;
#62295=EDGE_CURVE ( 'NONE', #73749, #146898, #4750, .T. ) ;
#62307=CARTESIAN_POINT ( 'NONE',  ( 10.53927507717300216, 2.018041202054248195, -6.084853302869510649 ) ) ;
#62322=ORIENTED_EDGE ( 'NONE', *, *, #165017, .T. ) ;
#62352=ORIENTED_EDGE ( 'NONE', *, *, #68459, .T. ) ;
#62359=ORIENTED_EDGE ( 'NONE', *, *, #157678, .T. ) ;
#62369=DIRECTION ( 'NONE',  ( -0.000000000000000000, -1.000000000000000000, -0.000000000000000000 ) ) ;
#62396=B_SPLINE_CURVE_WITH_KNOTS ( 'NONE', 3,
 ( #186986, #1811, #134016, #87368, #734, #51675, #132940 ),
 .UNSPECIFIED., .F., .F.,
 ( 4, 3, 4 ),
 ( 0.0001135037246152888473, 0.0006245292469112881514, 0.002007692286193847424 ),
 .UNSPECIFIED. ) ;
#62398=CARTESIAN_POINT ( 'NONE',  ( 0.000000000000000000, -5.223431457505076203, 0.000000000000000000 ) ) ;
#62429=EDGE_LOOP ( 'NONE', ( #118493, #200815, #194477, #141120 ) ) ;
#62435=DIRECTION ( 'NONE',  ( 0.000000000000000000, 1.000000000000000000, 0.000000000000000000 ) ) ;
#62478=CARTESIAN_POINT ( 'NONE',  ( 10.94245301910277668, 3.162178953954597471, -3.962121973755224680 ) ) ;
#62480=AXIS2_PLACEMENT_3D ( 'NONE', #103712, #19234, #170833 ) ;
#62489=DIRECTION ( 'NONE',  ( -0.000000000000000000, -1.000000000000000000, -0.000000000000000000 ) ) ;
#62490=ORIENTED_EDGE ( 'NONE', *, *, #106413, .F. ) ;
#62515=SURFACE_STYLE_FILL_AREA ( #179485 ) ;
#62527=ADVANCED_FACE ( 'NONE', ( #186858 ), #87246, .T. ) ;
#62565=ORIENTED_EDGE ( 'NONE', *, *, #48830, .F. ) ;
#62591=ORIENTED_EDGE ( 'NONE', *, *, #184771, .T. ) ;
#62610=B_SPLINE_CURVE_WITH_KNOTS ( 'NONE', 3,
 ( #60870, #177836, #146421, #145375 ),
 .UNSPECIFIED., .F., .F.,
 ( 4, 4 ),
 ( 1.084337306069862702E-15, 8.505390839925406612E-05 ),
 .UNSPECIFIED. ) ;
#62637=EDGE_CURVE ( 'NONE', #71330, #212186, #76880, .T. ) ;
#62644=CARTESIAN_POINT ( 'NONE',  ( 0.1826339422288050240, -7.841768514962160097, -10.96557956857097160 ) ) ;
#62648=SURFACE_SIDE_STYLE ('',( #131967 ) ) ;
#62649=CARTESIAN_POINT ( 'NONE',  ( -10.38819714233668456, 3.487142912321096855, -5.997628416522944761 ) ) ;
#62712=CARTESIAN_POINT ( 'NONE',  ( -2.494940289813118994, 3.447199233515649386, 11.73777120880565583 ) ) ;
#62721=CARTESIAN_POINT ( 'NONE',  ( -9.029845422049838533, 1.720726420432414638, -7.609771484012884279 ) ) ;
#62733=CARTESIAN_POINT ( 'NONE',  ( -0.3080734816351294314, -8.169755926620753783, -9.495223711095173158 ) ) ;
#62745=DIRECTION ( 'NONE',  ( 0.000000000000000000, 0.000000000000000000, -1.000000000000000000 ) ) ;
#62749=FACE_OUTER_BOUND ( 'NONE', #208758, .T. ) ;
#62759=CARTESIAN_POINT ( 'NONE',  ( -6.396834479292370368, -8.176568542494905500, -7.055228938194266775 ) ) ;
#62772=CARTESIAN_POINT ( 'NONE',  ( 4.232369794311310053E-13, -9.350066838357705024, 9.500000000000001776 ) ) ;
#62810=CARTESIAN_POINT ( 'NONE',  ( -6.605500049835229426, -8.049367966558005349, -6.875062624577632064 ) ) ;
#62840=EDGE_CURVE ( 'NONE', #166319, #36647, #142637, .T. ) ;
#62862=CARTESIAN_POINT ( 'NONE',  ( 7.806953216197655365, -6.479141885268318468, 7.749822179018618584 ) ) ;
#62866=DIRECTION ( 'NONE',  ( -0.000000000000000000, -1.000000000000000000, -0.000000000000000000 ) ) ;
#62872=ORIENTED_EDGE ( 'NONE', *, *, #124338, .F. ) ;
#62938=ORIENTED_EDGE ( 'NONE', *, *, #58624, .T. ) ;
#62943=VERTEX_POINT ( 'NONE', #185279 ) ;
#62944=CARTESIAN_POINT ( 'NONE',  ( -11.37385970535894231, 1.000000000000000888, 3.825613075418397457 ) ) ;
#62972=CARTESIAN_POINT ( 'NONE',  ( 7.664830294503436114, -9.999999999999994671, -7.777967379493309075 ) ) ;
#62973=CARTESIAN_POINT ( 'NONE',  ( 1.438959988998140160E-15, 4.000000000000003553, 11.50000000000000000 ) ) ;
#62981=EDGE_CURVE ( 'NONE', #19391, #208229, #105319, .T. ) ;
#63011=DIRECTION ( 'NONE',  ( 0.000000000000000000, 0.000000000000000000, 1.000000000000000000 ) ) ;
#63016=ORIENTED_EDGE ( 'NONE', *, *, #153420, .F. ) ;
#63075=AXIS2_PLACEMENT_3D ( 'NONE', #66135, #83480, #163693 ) ;
#63083=CARTESIAN_POINT ( 'NONE',  ( 7.869907033621586834, -7.024005807131050716, -7.214015686748633804 ) ) ;
#63098=PRESENTATION_STYLE_ASSIGNMENT (( #194158 ) ) ;
#63100=( LENGTH_UNIT ( ) NAMED_UNIT ( * ) SI_UNIT ( .MILLI., .METRE. ) );
#63161=ORIENTED_EDGE ( 'NONE', *, *, #62637, .F. ) ;
#63165=ORIENTED_EDGE ( 'NONE', *, *, #64003, .T. ) ;
#63191=AXIS2_PLACEMENT_3D ( 'NONE', #87300, #54802, #2814 ) ;
#63235=CARTESIAN_POINT ( 'NONE',  ( 10.39649820107524825, 2.629643693813620509, -5.992760101887531832 ) ) ;
#63243=CARTESIAN_POINT ( 'NONE',  ( 0.000000000000000000, -8.233137084989849086, 0.000000000000000000 ) ) ;
#63254=DIRECTION ( 'NONE',  ( 0.000000000000000000, 1.000000000000000000, 0.000000000000000000 ) ) ;
#63282=ORIENTED_EDGE ( 'NONE', *, *, #158238, .F. ) ;
#63289=AXIS2_PLACEMENT_3D ( 'NONE', #39388, #89225, #188837 ) ;
#63311=EDGE_CURVE ( 'NONE', #162142, #78601, #133975, .T. ) ;
#63361=EDGE_CURVE ( 'NONE', #56186, #191954, #149552, .T. ) ;
#63384=CARTESIAN_POINT ( 'NONE',  ( 8.912450614902654777, 3.507114751586604129, 8.024806578262976942 ) ) ;
#63402=CARTESIAN_POINT ( 'NONE',  ( 0.3867890553498105066, 3.235871879154613051, -11.62250415223146938 ) ) ;
#63424=DIRECTION ( 'NONE',  ( 0.000000000000000000, -1.000000000000000000, 0.000000000000000000 ) ) ;
#63429=ORIENTED_EDGE ( 'NONE', *, *, #10155, .F. ) ;
#63462=ORIENTED_EDGE ( 'NONE', *, *, #188812, .T. ) ;
#63469=PRESENTATION_STYLE_ASSIGNMENT (( #12568 ) ) ;
#63509=CARTESIAN_POINT ( 'NONE',  ( -9.606148981167596190, -6.583980363595129504, 0.4355862708379978354 ) ) ;
#63516=EDGE_CURVE ( 'NONE', #135108, #19237, #208445, .T. ) ;
#63560=CARTESIAN_POINT ( 'NONE',  ( 10.99962150373185210, -9.919999999999998153, -0.09125116240077391083 ) ) ;
#63574=CARTESIAN_POINT ( 'NONE',  ( 7.777967379493318845, -6.134628647623485698, 7.664830294503448549 ) ) ;
#63588=( NAMED_UNIT ( * ) SI_UNIT ( $, .STERADIAN. ) SOLID_ANGLE_UNIT ( ) );
#63616=CARTESIAN_POINT ( 'NONE',  ( 11.37385970535889257, 1.000000000000000888, -3.825613075418463627 ) ) ;
#63645=EDGE_CURVE ( 'NONE', #176780, #199252, #163481, .T. ) ;
#63671=CARTESIAN_POINT ( 'NONE',  ( 7.788485247869523675, -6.306978362809961602, -7.768428355095886140 ) ) ;
#63688=SHAPE_REPRESENTATION ( 'air flow regulation', ( #200407 ), #83064 ) ;
#63689=( GEOMETRIC_REPRESENTATION_CONTEXT ( 3 ) GLOBAL_UNCERTAINTY_ASSIGNED_CONTEXT ( ( #161602 ) ) GLOBAL_UNIT_ASSIGNED_CONTEXT ( ( #201277, #170931, #105994 ) ) REPRESENTATION_CONTEXT ( 'NONE', 'WORKASPACE' ) );
#63783=SURFACE_SIDE_STYLE ('',( #178619 ) ) ;
#63784=FACE_OUTER_BOUND ( 'NONE', #95844, .T. ) ;
#63787=DIRECTION ( 'NONE',  ( 0.000000000000000000, -1.000000000000000000, 0.000000000000000000 ) ) ;
#63810=FILL_AREA_STYLE ('',( #142972 ) ) ;
#63816=CARTESIAN_POINT ( 'NONE',  ( -10.15205317230718407, 3.956598013261175772, 5.494609294606044081 ) ) ;
#63826=UNCERTAINTY_MEASURE_WITH_UNIT (LENGTH_MEASURE( 1.000000000000000082E-05 ), #58068, 'distance_accuracy_value', 'NONE');
#63827=CARTESIAN_POINT ( 'NONE',  ( 0.4655551865852024518, -8.176568542494939251, 9.512045263456274213 ) ) ;
#63875=EDGE_CURVE ( 'NONE', #164527, #54346, #173938, .T. ) ;
#63878=CARTESIAN_POINT ( 'NONE',  ( 9.579665964948885559, -7.246166700194470067, 0.07999999999999847511 ) ) ;
#63883=CARTESIAN_POINT ( 'NONE',  ( -0.1236583036082171405, 1.000000000000000888, 11.99936284241579898 ) ) ;
#63901=CARTESIAN_POINT ( 'NONE',  ( 6.663994888585877518, -7.154544010627095219, -6.770610912236881163 ) ) ;
#63903=EDGE_CURVE ( 'NONE', #90583, #147438, #70046, .T. ) ;
#63929=ORIENTED_EDGE ( 'NONE', *, *, #106815, .T. ) ;
#63976=CIRCLE ( 'NONE', #167259, 0.08000000000000044575 ) ;
#64003=EDGE_CURVE ( 'NONE', #130351, #157630, #35432, .T. ) ;
#64019=AXIS2_PLACEMENT_3D ( 'NONE', #152689, #100737, #184110 ) ;
#64020=CARTESIAN_POINT ( 'NONE',  ( -0.1363799957457066114, -9.242177669965698783, 9.620888806888750366 ) ) ;
#64046=ORIENTED_EDGE ( 'NONE', *, *, #109647, .T. ) ;
#64047=CARTESIAN_POINT ( 'NONE',  ( 6.396834479292727416, -8.176568542494925040, 7.055228938193930155 ) ) ;
#64057=DIRECTION ( 'NONE',  ( 0.000000000000000000, 0.000000000000000000, -1.000000000000000000 ) ) ;
#64072=EDGE_CURVE ( 'NONE', #189856, #90864, #194541, .T. ) ;
#64076=DIRECTION ( 'NONE',  ( -1.561558963378126405E-12, 1.000000000000000000, -1.535693738323023938E-12 ) ) ;
#64089=B_SPLINE_CURVE_WITH_KNOTS ( 'NONE', 3,
 ( #184918, #117872, #120011, #69027, #18145, #35476, #20289, #101554 ),
 .UNSPECIFIED., .F., .F.,
 ( 4, 2, 2, 4 ),
 ( 0.000000000000000000, 0.0002567066673176282847, 0.0005134133346352565694, 0.001026826669270514006 ),
 .UNSPECIFIED. ) ;
#64090=DIRECTION ( 'NONE',  ( -0.03984146075563027578, 0.000000000000000000, 0.9992060137953822085 ) ) ;
#64121=STYLED_ITEM ( 'NONE', ( #155445 ), #122337 ) ;
#64146=CARTESIAN_POINT ( 'NONE',  ( 11.32145367647655476, 0.9706168436483538775, -3.678563289475825560 ) ) ;
#64176=CARTESIAN_POINT ( 'NONE',  ( -0.001932293024938683355, -9.922538603026485049, -10.91970414279958135 ) ) ;
#64189=CARTESIAN_POINT ( 'NONE',  ( 0.2868663046952837914, -5.229832900979505261, 10.99643026930483636 ) ) ;
#64216=CARTESIAN_POINT ( 'NONE',  ( 7.720982897393566802, -5.907420853759296264, -7.834948825496929281 ) ) ;
#64219=EDGE_CURVE ( 'NONE', #80737, #109006, #125524, .T. ) ;
#64238=ORIENTED_EDGE ( 'NONE', *, *, #6325, .F. ) ;
#64242=FACE_OUTER_BOUND ( 'NONE', #89560, .T. ) ;
#64245=CARTESIAN_POINT ( 'NONE',  ( -9.611540586923190688, -6.723650695528641918, 0.1589091098076336750 ) ) ;
#64262=CARTESIAN_POINT ( 'NONE',  ( 7.769310276573696328, -5.221243112839685452, -7.769310276573722085 ) ) ;
#64264=VECTOR ( 'NONE', #83782, 1000.000000000000000 ) ;
#64436=CARTESIAN_POINT ( 'NONE',  ( -10.99976946526262900, -5.360092950639650411, 0.08269815893113317828 ) ) ;
#64440=( NAMED_UNIT ( * ) SI_UNIT ( $, .STERADIAN. ) SOLID_ANGLE_UNIT ( ) );
#64452=CARTESIAN_POINT ( 'NONE',  ( 0.000000000000000000, -5.223431457505076203, 0.000000000000000000 ) ) ;
#64489=FACE_OUTER_BOUND ( 'NONE', #54928, .T. ) ;
#64494=ORIENTED_EDGE ( 'NONE', *, *, #85988, .F. ) ;
#64497=CARTESIAN_POINT ( 'NONE',  ( -0.4694063952341946955, -6.893137084989842123, -10.98997987423602751 ) ) ;
#64505=CARTESIAN_POINT ( 'NONE',  ( -10.99970480893081870, -9.999999999999994671, -0.08058608058607828750 ) ) ;
#64527=ORIENTED_EDGE ( 'NONE', *, *, #181792, .T. ) ;
#64590=UNCERTAINTY_MEASURE_WITH_UNIT (LENGTH_MEASURE( 1.000000000000000082E-05 ), #63100, 'distance_accuracy_value', 'NONE');
#64603=AXIS2_PLACEMENT_3D ( 'NONE', #24764, #169953, #187272 ) ;
#64630=ORIENTED_EDGE ( 'NONE', *, *, #213004, .T. ) ;
#64639=ORIENTED_EDGE ( 'NONE', *, *, #85988, .T. ) ;
#64642=CARTESIAN_POINT ( 'NONE',  ( 7.649321060469609357, -7.336076765398686028, -6.992767129439135587 ) ) ;
#64742=STYLED_ITEM ( 'NONE', ( #206622 ), #149431 ) ;
#64746=CARTESIAN_POINT ( 'NONE',  ( -6.773376349083143566, -7.215597533173308875, -6.661184041420940005 ) ) ;
#64754=CARTESIAN_POINT ( 'NONE',  ( 6.776323679500987573, -7.189645481333916344, 6.777910281175898000 ) ) ;
#64759=CARTESIAN_POINT ( 'NONE',  ( 0.000000000000000000, 4.000000000000003553, 0.000000000000000000 ) ) ;
#64782=CARTESIAN_POINT ( 'NONE',  ( 0.008694310353105784428, -8.101927612791786970, -11.00038155431018438 ) ) ;
#64785=FILL_AREA_STYLE_COLOUR ( '', #144243 ) ;
#64787=( LENGTH_UNIT ( ) NAMED_UNIT ( * ) SI_UNIT ( .MILLI., .METRE. ) );
#64826=EDGE_CURVE ( 'NONE', #111346, #109058, #182762, .T. ) ;
#64834=CARTESIAN_POINT ( 'NONE',  ( 0.4655551865852050608, -8.176568542494919711, 9.512045263456268884 ) ) ;
#64840=ORIENTED_EDGE ( 'NONE', *, *, #188521, .T. ) ;
#64850=CARTESIAN_POINT ( 'NONE',  ( -9.499690612162398295, -9.919996481418280609, 0.07742489488620404869 ) ) ;
#64860=ORIENTED_EDGE ( 'NONE', *, *, #173047, .T. ) ;
#64883=ORIENTED_EDGE ( 'NONE', *, *, #194704, .F. ) ;
#64886=CARTESIAN_POINT ( 'NONE',  ( 0.3199376857464626411, -8.148349307653466767, 9.520891725236003467 ) ) ;
#64895=CIRCLE ( 'NONE', #151339, 9.479622692290801567 ) ;
#64904=CARTESIAN_POINT ( 'NONE',  ( 0.07933194154488537597, -7.246166700194011767, -9.499668754385634628 ) ) ;
#64947=ORIENTED_EDGE ( 'NONE', *, *, #89214, .F. ) ;
#64949=ADVANCED_FACE ( 'NONE', ( #129113 ), #132124, .T. ) ;
#64982=CARTESIAN_POINT ( 'NONE',  ( 0.001932266794894933271, -9.922538451904662438, 9.579662758527193844 ) ) ;
#64983=CARTESIAN_POINT ( 'NONE',  ( -7.721398836998405457, -6.134628647623499909, -7.721398836998363713 ) ) ;
#65003=CIRCLE ( 'NONE', #186070, 11.69999999999999041 ) ;
#65012=DIRECTION ( 'NONE',  ( 0.000000000000000000, 1.000000000000000000, 0.000000000000000000 ) ) ;
#65020=EDGE_LOOP ( 'NONE', ( #196952, #101812, #128124, #179062, #40783 ) ) ;
#65079=DIRECTION ( 'NONE',  ( 0.000000000000000000, 0.000000000000000000, 1.000000000000000000 ) ) ;
#65087=CARTESIAN_POINT ( 'NONE',  ( 6.496114076516082747, -8.169775483750532530, 6.932145363377579805 ) ) ;
#65129=VERTEX_POINT ( 'NONE', #5371 ) ;
#65237=CARTESIAN_POINT ( 'NONE',  ( -6.776323679501130570, -7.189645481333919896, -6.777910281175996587 ) ) ;
#65255=EDGE_CURVE ( 'NONE', #40132, #172181, #32782, .T. ) ;
#65325=DIRECTION ( 'NONE',  ( 0.000000000000000000, 0.000000000000000000, 1.000000000000000000 ) ) ;
#65335=ORIENTED_EDGE ( 'NONE', *, *, #4201, .T. ) ;
#65376=TOROIDAL_SURFACE ( 'NONE', #189869, 10.92000000000000348, 0.08000000000000000167 ) ;
#65416=ORIENTED_EDGE ( 'NONE', *, *, #105983, .T. ) ;
#65438=EDGE_CURVE ( 'NONE', #163559, #194999, #169723, .T. ) ;
#65471=SURFACE_STYLE_FILL_AREA ( #16725 ) ;
#65472=B_SPLINE_CURVE_WITH_KNOTS ( 'NONE', 3,
 ( #67368, #99912, #96742, #200578, #212577, #162790, #49037, #134578, #66304, #64216 ),
 .UNSPECIFIED., .F., .F.,
 ( 4, 2, 2, 2, 4 ),
 ( 0.000000000000000000, 0.0002503535593264579048, 0.0005007071186529158096, 0.0007510606779793737144, 0.001001414237305831619 ),
 .UNSPECIFIED. ) ;
#65507=EDGE_CURVE ( 'NONE', #82527, #74942, #208592, .T. ) ;
#65514=EDGE_LOOP ( 'NONE', ( #77859, #119841, #103014, #33019, #179984, #114772, #126425, #25568 ) ) ;
#65564=CARTESIAN_POINT ( 'NONE',  ( -7.787098537122150610, -5.543994141378503215, 7.698131257602418565 ) ) ;
#65579=CARTESIAN_POINT ( 'NONE',  ( 6.722000117219828930, -7.189371949512757709, -6.713552092916842184 ) ) ;
#65587=CARTESIAN_POINT ( 'NONE',  ( 0.03969736035583037309, -7.921780080556623638, -11.00000000000012967 ) ) ;
#65613=B_SPLINE_CURVE_WITH_KNOTS ( 'NONE', 3,
 ( #33388, #1931, #200141, #35516, #137317, #188171, #102670, #56052 ),
 .UNSPECIFIED., .F., .F.,
 ( 4, 2, 2, 4 ),
 ( 4.051276326462483916E-18, 0.0002224730689913823186, 0.0004449461379827605715, 0.0008898922759655192999 ),
 .UNSPECIFIED. ) ;
#65644=DIRECTION ( 'NONE',  ( 0.000000000000000000, 1.000000000000000000, 0.000000000000000000 ) ) ;
#65670=ORIENTED_EDGE ( 'NONE', *, *, #126069, .T. ) ;
#65683=PRESENTATION_STYLE_ASSIGNMENT (( #145941 ) ) ;
#65684=CARTESIAN_POINT ( 'NONE',  ( -0.08000000000000714873, -6.134628647623513231, 10.91970695577494865 ) ) ;
#65685=CARTESIAN_POINT ( 'NONE',  ( -0.1421055763938854355, -7.985988503423670615, -9.537847510268186113 ) ) ;
#65775=ORIENTED_EDGE ( 'NONE', *, *, #33554, .F. ) ;
#65792=CARTESIAN_POINT ( 'NONE',  ( 9.579698345292687378, -7.154544010627095219, 0.07602376731354922035 ) ) ;
#65816=CARTESIAN_POINT ( 'NONE',  ( -6.604641253243921817, -6.414086731524404783, -7.221001870987140414 ) ) ;
#65821=SURFACE_SIDE_STYLE ('',( #82100 ) ) ;
#65822=ADVANCED_FACE ( 'NONE', ( #18977 ), #181492, .T. ) ;
#65823=CARTESIAN_POINT ( 'NONE',  ( 9.578206935422338475, -9.907361015872668375, -0.1671882239541239157 ) ) ;
#65842=ORIENTED_EDGE ( 'NONE', *, *, #163961, .T. ) ;
#65889=EDGE_CURVE ( 'NONE', #109006, #94442, #200786, .T. ) ;
#65891=CARTESIAN_POINT ( 'NONE',  ( 0.000000000000000000, 0.7999999999999951594, 0.000000000000000000 ) ) ;
#65898=ORIENTED_EDGE ( 'NONE', *, *, #36376, .F. ) ;
#65920=CARTESIAN_POINT ( 'NONE',  ( -9.818302567231157241, -8.862962251182134210, 0.6073963244357452052 ) ) ;
#65942=TOROIDAL_SURFACE ( 'NONE', #38314, 10.92000000000000171, 0.08000000000000000167 ) ;
#65989=TOROIDAL_SURFACE ( 'NONE', #173197, 10.92000000000000348, 0.08000000000000000167 ) ;
#65995=CARTESIAN_POINT ( 'NONE',  ( 10.00050683067331114, 3.975933801733724238, 5.773795310721800966 ) ) ;
#66027=CARTESIAN_POINT ( 'NONE',  ( -0.08367765422325271207, -9.912493506416723221, -9.499631469177289844 ) ) ;
#66042=DIRECTION ( 'NONE',  ( 0.000000000000000000, 0.000000000000000000, 1.000000000000000000 ) ) ;
#66045=EDGE_CURVE ( 'NONE', #81487, #14615, #22384, .T. ) ;
#66066=ORIENTED_EDGE ( 'NONE', *, *, #72448, .F. ) ;
#66101=ORIENTED_EDGE ( 'NONE', *, *, #188521, .F. ) ;
#66107=DIRECTION ( 'NONE',  ( 0.000000000000000000, 0.000000000000000000, -1.000000000000000000 ) ) ;
#66132=ORIENTED_EDGE ( 'NONE', *, *, #15332, .F. ) ;
#66133=CARTESIAN_POINT ( 'NONE',  ( -9.578446392664467623, -9.953004327042588528, 0.1519871474491493735 ) ) ;
#66135=CARTESIAN_POINT ( 'NONE',  ( 0.000000000000000000, -13.99999999999999822, 0.000000000000000000 ) ) ;
#66137=VECTOR ( 'NONE', #41577, 1000.000000000000000 ) ;
#66162=ADVANCED_FACE ( 'NONE', ( #201973 ), #156839, .T. ) ;
#66195=CIRCLE ( 'NONE', #121671, 0.07999999999999993228 ) ;
#66206=( BOUNDED_SURFACE ( )  B_SPLINE_SURFACE ( 3, 2, ( 
 ( #157564, #40611, #75233 ),
 ( #106716, #141343, #142401 ),
 ( #207357, #190036, #58978 ),
 ( #191091, #126198, #109937 ) ),
 .UNSPECIFIED., .F., .F., .T. ) 
 B_SPLINE_SURFACE_WITH_KNOTS ( ( 4, 4 ),
 ( 3, 3 ),
 ( 0.004991389062828482590, 0.008017777006561210146 ),
 ( 0.000000000000000000, 1.000000000000000000 ),
 .UNSPECIFIED. ) 
 GEOMETRIC_REPRESENTATION_ITEM ( )  RATIONAL_B_SPLINE_SURFACE ( (
 ( 1.000000000000000000, 0.7184380228464046780, 1.000000000000000000),
 ( 1.000000000000000000, 0.7185467277397590280, 1.000000000000000000),
 ( 1.000000000000000000, 0.7186585579880989672, 1.000000000000000000),
 ( 1.000000000000000000, 0.7187737999613676987, 1.000000000000000000) ) ) 
 REPRESENTATION_ITEM ( '' )  SURFACE ( )  );
#66225=CARTESIAN_POINT ( 'NONE',  ( -6.773376349083140013, 7.849261790823902629, -6.661184041420947111 ) ) ;
#66228=CARTESIAN_POINT ( 'NONE',  ( 9.486277548414619787, -9.200719317737716452, -0.5196196971346837001 ) ) ;
#66295=ORIENTED_EDGE ( 'NONE', *, *, #78986, .T. ) ;
#66299=ORIENTED_EDGE ( 'NONE', *, *, #192938, .F. ) ;
#66301=CARTESIAN_POINT ( 'NONE',  ( 7.487360338304382523, -6.465328379374282619, -7.487360338304409169 ) ) ;
#66304=CARTESIAN_POINT ( 'NONE',  ( 7.720982897393566802, -5.823938088759704534, -7.834948825496931057 ) ) ;
#66347=AXIS2_PLACEMENT_3D ( 'NONE', #176648, #144196, #95425 ) ;
#66367=EDGE_LOOP ( 'NONE', ( #60187, #196410, #79026, #51512 ) ) ;
#66377=CARTESIAN_POINT ( 'NONE',  ( 0.07999999999999327094, -8.407420853759283830, 10.91970695577496286 ) ) ;
#66456=DIRECTION ( 'NONE',  ( 0.000000000000000000, 1.000000000000000000, 0.000000000000000000 ) ) ;
#66492=AXIS2_PLACEMENT_3D ( 'NONE', #8195, #122042, #190145 ) ;
#66523=CARTESIAN_POINT ( 'NONE',  ( -11.00038526257045568, -5.601932402265104471, 0.008494835128522478310 ) ) ;
#66527=SURFACE_SIDE_STYLE ('',( #65471 ) ) ;
#66550=TOROIDAL_SURFACE ( 'NONE', #25147, 11.70000000000000107, 0.2000000000000000111 ) ;
#66568=CARTESIAN_POINT ( 'NONE',  ( 9.605899910213576476, -6.890735599539920209, -0.05097232478520941079 ) ) ;
#66584=CARTESIAN_POINT ( 'NONE',  ( 0.3641668253325698879, -9.063144096568546360, -9.630238394150364201 ) ) ;
#66608=ORIENTED_EDGE ( 'NONE', *, *, #68459, .F. ) ;
#66616=CARTESIAN_POINT ( 'NONE',  ( 10.99683038201373719, -5.197079954928569556, -0.2726351642629408212 ) ) ;
#66626=AXIS2_PLACEMENT_3D ( 'NONE', #167388, #44324, #94153 ) ;
#66630=VECTOR ( 'NONE', #68411, 1000.000000000000000 ) ;
#66651=FACE_OUTER_BOUND ( 'NONE', #185287, .T. ) ;
#66678=AXIS2_PLACEMENT_3D ( 'NONE', #35116, #120731, #5793 ) ;
#66712=EDGE_CURVE ( 'NONE', #161735, #73749, #118002, .T. ) ;
#66715=ORIENTED_EDGE ( 'NONE', *, *, #47373, .T. ) ;
#66741=CARTESIAN_POINT ( 'NONE',  ( -11.16489891154634861, 3.742896273583264932, 3.684481756086905424 ) ) ;
#66743=CARTESIAN_POINT ( 'NONE',  ( -1.040834085586084257E-14, -7.473374494045017968, -9.579665964948867796 ) ) ;
#66771=CARTESIAN_POINT ( 'NONE',  ( 10.91970695577495043, -6.134628647623513231, 5.204170427930421283E-15 ) ) ;
#66790=ORIENTED_EDGE ( 'NONE', *, *, #137134, .F. ) ;
#66793=VERTEX_POINT ( 'NONE', #1403 ) ;
#66824=ORIENTED_EDGE ( 'NONE', *, *, #119166, .F. ) ;
#66830=VERTEX_POINT ( 'NONE', #67464 ) ;
#66836=CARTESIAN_POINT ( 'NONE',  ( 10.99967557777141103, -6.699439830718304734, -0.09581361862938142515 ) ) ;
#66887=( NAMED_UNIT ( * ) SI_UNIT ( $, .STERADIAN. ) SOLID_ANGLE_UNIT ( ) );
#66907=ORIENTED_EDGE ( 'NONE', *, *, #36152, .F. ) ;
#66947=ORIENTED_EDGE ( 'NONE', *, *, #173047, .F. ) ;
#66950=MECHANICAL_DESIGN_GEOMETRIC_PRESENTATION_REPRESENTATION('',(#11631),#1249);
#66977=ADVANCED_FACE ( 'NONE', ( #179686 ), #133394, .T. ) ;
#66986=CYLINDRICAL_SURFACE ( 'NONE', #73160, 0.08000000000000020983 ) ;
#66987=FACE_OUTER_BOUND ( 'NONE', #102304, .T. ) ;
#67036=CARTESIAN_POINT ( 'NONE',  ( 0.08000000000000020983, -7.246166700194011767, -9.579665964948882007 ) ) ;
#67037=LINE ( 'NONE', #165639, #124016 ) ;
#67042=DIRECTION ( 'NONE',  ( 0.000000000000000000, 0.000000000000000000, 1.000000000000000000 ) ) ;
#67059=VERTEX_POINT ( 'NONE', #99500 ) ;
#67089=LINE ( 'NONE', #71360, #14606 ) ;
#67115=EDGE_CURVE ( 'NONE', #21086, #1801, #49661, .T. ) ;
#67128=LINE ( 'NONE', #159594, #177289 ) ;
#67151=PLANE ( 'NONE',  #106804 ) ;
#67169=( LENGTH_UNIT ( ) NAMED_UNIT ( * ) SI_UNIT ( .MILLI., .METRE. ) );
#67209=CARTESIAN_POINT ( 'NONE',  ( -9.579764304849156531, -9.919999999999998153, 0.06720017513374074158 ) ) ;
#67220=VECTOR ( 'NONE', #186874, 1000.000000000000000 ) ;
#67222=VERTEX_POINT ( 'NONE', #100558 ) ;
#67261=DIRECTION ( 'NONE',  ( 0.000000000000000000, 0.000000000000000000, -1.000000000000000000 ) ) ;
#67298=CARTESIAN_POINT ( 'NONE',  ( 9.495512617570035729, -9.134774474195877403, -0.2994571439533144641 ) ) ;
#67329=CIRCLE ( 'NONE', #164306, 9.499999999999991118 ) ;
#67334=DIRECTION ( 'NONE',  ( -0.6743504407196689865, -1.104276606162287428E-12, -0.7384114592157872137 ) ) ;
#67358=EDGE_LOOP ( 'NONE', ( #14644, #84808, #192965, #189629 ) ) ;
#67362=( GEOMETRIC_REPRESENTATION_CONTEXT ( 3 ) GLOBAL_UNCERTAINTY_ASSIGNED_CONTEXT ( ( #142675 ) ) GLOBAL_UNIT_ASSIGNED_CONTEXT ( ( #178473, #196841, #111402 ) ) REPRESENTATION_CONTEXT ( 'NONE', 'WORKASPACE' ) );
#67363=EDGE_LOOP ( 'NONE', ( #178576, #104790, #17360, #101463 ) ) ;
#67365=CARTESIAN_POINT ( 'NONE',  ( 6.781144757626058173, -7.161464053357574855, -6.776370306708051849 ) ) ;
#67368=CARTESIAN_POINT ( 'NONE',  ( 8.081892667527529994, -5.166862915010145052, -7.462104991928515396 ) ) ;
#67370=EDGE_LOOP ( 'NONE', ( #101913, #169234, #107968, #38788 ) ) ;
#67375=CARTESIAN_POINT ( 'NONE',  ( -6.381095703207997794, -8.233137084989849086, -7.037870247915931188 ) ) ;
#67377=( GEOMETRIC_REPRESENTATION_CONTEXT ( 3 ) GLOBAL_UNCERTAINTY_ASSIGNED_CONTEXT ( ( #30210 ) ) GLOBAL_UNIT_ASSIGNED_CONTEXT ( ( #27032, #80059, #61682 ) ) REPRESENTATION_CONTEXT ( 'NONE', 'WORKASPACE' ) );
#67378=CARTESIAN_POINT ( 'NONE',  ( 9.499643733017418157, -9.912496545390952818, -0.08228199421454375495 ) ) ;
#67406=CARTESIAN_POINT ( 'NONE',  ( 10.99954523395721218, -9.918132210574695407, -0.1000458187401192384 ) ) ;
#67464=CARTESIAN_POINT ( 'NONE',  ( 0.4294077647110511320, -6.532648833121157850, 9.469892045836672878 ) ) ;
#67485=CARTESIAN_POINT ( 'NONE',  ( 0.1062647551455935674, -6.683951888245091233, 9.488025208486869033 ) ) ;
#67487=FACE_OUTER_BOUND ( 'NONE', #172415, .T. ) ;
#67494=B_SPLINE_CURVE_WITH_KNOTS ( 'NONE', 3,
 ( #96686, #180041, #31663, #82518, #147546, #162735, #68386, #163799 ),
 .UNSPECIFIED., .F., .F.,
 ( 4, 2, 2, 4 ),
 ( 0.000000000000000000, 0.0005156231957999836413, 0.0007734347936999756788, 0.001031246391599967716 ),
 .UNSPECIFIED. ) ;
#67510=CIRCLE ( 'NONE', #22673, 0.08000000000000020983 ) ;
#67522=CARTESIAN_POINT ( 'NONE',  ( 0.000000000000000000, 3.956598013261175772, 0.000000000000000000 ) ) ;
#67530=CARTESIAN_POINT ( 'NONE',  ( -6.234224025626352805, -6.938199013094628498, -6.849482339516213436 ) ) ;
#67540=CARTESIAN_POINT ( 'NONE',  ( 2.494940289813108780, 4.000000000000003553, -11.73777120880564695 ) ) ;
#67544=CARTESIAN_POINT ( 'NONE',  ( -8.832353407160665526, 3.956598013261175772, -7.432338980325321920 ) ) ;
#67550=LINE ( 'NONE', #117468, #174078 ) ;
#67592=CARTESIAN_POINT ( 'NONE',  ( -11.00023563321887643, -5.575210796978346650, -0.04341786867403560346 ) ) ;
#67633=CARTESIAN_POINT ( 'NONE',  ( 9.469892045836667549, -6.532648833121162291, -0.4294077647110499663 ) ) ;
#67649=CARTESIAN_POINT ( 'NONE',  ( -0.4370080631058587683, -8.003595416197006429, 10.68747925529770804 ) ) ;
#67650=CARTESIAN_POINT ( 'NONE',  ( 7.055228938194279209, -8.176568542494891290, -6.396834479292358822 ) ) ;
#67808=CARTESIAN_POINT ( 'NONE',  ( -9.469892045836674654, -6.532648833121171172, 0.4294077647110563500 ) ) ;
#67809=CARTESIAN_POINT ( 'NONE',  ( 7.777967379493318845, -6.134628647623485698, 7.664830294503448549 ) ) ;
#67836=ORIENTED_EDGE ( 'NONE', *, *, #101693, .F. ) ;
#67846=CARTESIAN_POINT ( 'NONE',  ( -1.138412281109779656E-15, -7.868711954895459826, -9.183873791909949347 ) ) ;
#67862=EDGE_CURVE ( 'NONE', #15203, #125480, #14330, .T. ) ;
#67879=CARTESIAN_POINT ( 'NONE',  ( 10.93186801223270521, -5.758458176070768708, 2.033726106357576692E-15 ) ) ;
#67908=EDGE_CURVE ( 'NONE', #175582, #113279, #146494, .T. ) ;
#67909=CARTESIAN_POINT ( 'NONE',  ( 10.99979681685432631, -6.306104522322590000, 0.07019693227477653841 ) ) ;
#67915=PLANE ( 'NONE',  #36622 ) ;
#68039=B_SPLINE_CURVE_WITH_KNOTS ( 'NONE', 3,
 ( #198619, #69683, #53454, #19876 ),
 .UNSPECIFIED., .F., .F.,
 ( 4, 4 ),
 ( 0.000000000000000000, 9.170750103568812571E-05 ),
 .UNSPECIFIED. ) ;
#68043=CYLINDRICAL_SURFACE ( 'NONE', #101887, 11.99999999999999112 ) ;
#68115=VECTOR ( 'NONE', #25581, 1000.000000000000000 ) ;
#68122=B_SPLINE_CURVE_WITH_KNOTS ( 'NONE', 3,
 ( #11162, #78307, #77239, #126081, #142284, #176887 ),
 .UNSPECIFIED., .F., .F.,
 ( 4, 2, 4 ),
 ( 0.0004065497138311910700, 0.0007003026727366323291, 0.0009940556316420734798 ),
 .UNSPECIFIED. ) ;
#68136=FILL_AREA_STYLE_COLOUR ( '', #138982 ) ;
#68144=CONICAL_SURFACE ( 'NONE', #16355, 10.99999999999999112, 0.7853981633974479459 ) ;
#68145=ORIENTED_EDGE ( 'NONE', *, *, #184735, .T. ) ;
#68165=VERTEX_POINT ( 'NONE', #191931 ) ;
#68168=CARTESIAN_POINT ( 'NONE',  ( -0.09264309395031754268, -9.919020119916163836, -9.499548513212880962 ) ) ;
#68180=CARTESIAN_POINT ( 'NONE',  ( -7.110792111438893670, -7.169578370797517586, -7.767011945534271433 ) ) ;
#68183=ORIENTED_EDGE ( 'NONE', *, *, #143796, .T. ) ;
#68204=SPHERICAL_SURFACE ( 'NONE', #141222, 9.500000000000001776 ) ;
#68221=ORIENTED_EDGE ( 'NONE', *, *, #184032, .T. ) ;
#68223=DIRECTION ( 'NONE',  ( 0.000000000000000000, 0.000000000000000000, -1.000000000000000000 ) ) ;
#68321=CARTESIAN_POINT ( 'NONE',  ( -6.773846765317318663, -7.246166700180828535, 6.773846765317342644 ) ) ;
#68339=CARTESIAN_POINT ( 'NONE',  ( 9.617648866954018771, -9.063431457505044975, -0.6035590660249217088 ) ) ;
#68366=( BOUNDED_SURFACE ( )  B_SPLINE_SURFACE ( 3, 2, ( 
 ( #146787, #27667, #144665 ),
 ( #126320, #160878, #163017 ),
 ( #62307, #12472, #11404 ),
 ( #15665, #93762, #192281 ) ),
 .UNSPECIFIED., .F., .F., .T. ) 
 B_SPLINE_SURFACE_WITH_KNOTS ( ( 4, 4 ),
 ( 3, 3 ),
 ( 0.005239860189960162014, 0.008266248133684695604 ),
 ( 0.000000000000000000, 1.000000000000000000 ),
 .UNSPECIFIED. ) 
 GEOMETRIC_REPRESENTATION_ITEM ( )  RATIONAL_B_SPLINE_SURFACE ( (
 ( 1.000000000000000000, 0.7187737999613659223, 1.000000000000000000),
 ( 1.000000000000000000, 0.7186585579881040742, 1.000000000000000000),
 ( 1.000000000000000000, 0.7185467277397524777, 1.000000000000000000),
 ( 1.000000000000000000, 0.7184380228464086748, 1.000000000000000000) ) ) 
 REPRESENTATION_ITEM ( '' )  SURFACE ( )  );
#68386=CARTESIAN_POINT ( 'NONE',  ( 7.503508839934897701, -6.893137084989714225, 8.043940816608046163 ) ) ;
#68401=CARTESIAN_POINT ( 'NONE',  ( -8.581532217057265655, 3.975933801733725570, -7.726846314510518177 ) ) ;
#68404=AXIS2_PLACEMENT_3D ( 'NONE', #140817, #206830, #58464 ) ;
#68411=DIRECTION ( 'NONE',  ( -0.000000000000000000, 1.000000000000000000, -0.000000000000000000 ) ) ;
#68450=AXIS2_PLACEMENT_3D ( 'NONE', #157192, #42390, #93273 ) ;
#68454=CARTESIAN_POINT ( 'NONE',  ( -6.444907381559357162, -8.233136965322206180, -6.980013479859866976 ) ) ;
#68456=CARTESIAN_POINT ( 'NONE',  ( -10.99954523395721218, -9.918132210574695407, 0.1000458187401208898 ) ) ;
#68459=EDGE_CURVE ( 'NONE', #138893, #93013, #104906, .T. ) ;
#68478=ORIENTED_EDGE ( 'NONE', *, *, #109387, .T. ) ;
#68481=DIRECTION ( 'NONE',  ( 0.000000000000000000, 1.000000000000000000, 0.000000000000000000 ) ) ;
#68484=CARTESIAN_POINT ( 'NONE',  ( 10.99943592164172657, -9.900000000000005684, -0.1113975120798811613 ) ) ;
#68509=ORIENTED_EDGE ( 'NONE', *, *, #28884, .T. ) ;
#68561=CARTESIAN_POINT ( 'NONE',  ( -6.735631571019096932E-15, -9.954378579146949235, 10.91970693179565544 ) ) ;
#68606=CARTESIAN_POINT ( 'NONE',  ( -7.769310276573725638, -5.221243112839681011, -7.769310276573695440 ) ) ;
#68613=CARTESIAN_POINT ( 'NONE',  ( 8.917737905728806425, 3.447199233515649386, 8.029567276306217138 ) ) ;
#68679=CARTESIAN_POINT ( 'NONE',  ( 0.4694063952341808177, -6.893137084989842123, 10.98997987423603995 ) ) ;
#68772=( BOUNDED_SURFACE ( )  B_SPLINE_SURFACE ( 3, 2, ( 
 ( #141997, #56446, #124731 ),
 ( #59635, #172334, #188569 ),
 ( #42349, #125793, #108464 ),
 ( #71598, #40200, #105212 ) ),
 .UNSPECIFIED., .F., .F., .F. ) 
 B_SPLINE_SURFACE_WITH_KNOTS ( ( 4, 4 ),
 ( 3, 3 ),
 ( 0.04893088146668655297, 0.05137248493452929027 ),
 ( 0.000000000000000000, 1.000000000000000000 ),
 .UNSPECIFIED. ) 
 GEOMETRIC_REPRESENTATION_ITEM ( )  RATIONAL_B_SPLINE_SURFACE ( (
 ( 1.000000000000000000, 0.7169884966214685740, 1.000000000000000000),
 ( 1.000000000000000000, 0.7174883642158066399, 1.000000000000000000),
 ( 1.000000000000000000, 0.7180610417773352072, 1.000000000000000000),
 ( 1.000000000000000000, 0.7187540717311200478, 1.000000000000000000) ) ) 
 REPRESENTATION_ITEM ( '' )  SURFACE ( )  );
#68781=VERTEX_POINT ( 'NONE', #22041 ) ;
#68788=CARTESIAN_POINT ( 'NONE',  ( 0.000000000000000000, 4.006659545634088992, 0.000000000000000000 ) ) ;
#68856=DIRECTION ( 'NONE',  ( -0.000000000000000000, -1.000000000000000000, -0.000000000000000000 ) ) ;
#68887=CARTESIAN_POINT ( 'NONE',  ( 10.91804383151480806, -8.407420853759271395, -0.1905751639681791121 ) ) ;
#68898=CARTESIAN_POINT ( 'NONE',  ( 0.04481625915944963123, -9.999534456186202291, 9.500049708089882472 ) ) ;
#68913=CARTESIAN_POINT ( 'NONE',  ( 7.664830294503436114, -6.134628647623485698, -7.777967379493309075 ) ) ;
#68918=CARTESIAN_POINT ( 'NONE',  ( -7.778383330260346007, -6.134628647623487474, 7.778383330260379758 ) ) ;
#68921=DIRECTION ( 'NONE',  ( -0.04267330865764933784, 4.780913106218958965E-15, -0.9990890794760041160 ) ) ;
#68964=EDGE_CURVE ( 'NONE', #54346, #82463, #160381, .T. ) ;
#68989=CARTESIAN_POINT ( 'NONE',  ( -9.488968570712932760, -6.747343053191825923, 0.2633404184769590484 ) ) ;
#69011=ORIENTED_EDGE ( 'NONE', *, *, #127553, .T. ) ;
#69027=CARTESIAN_POINT ( 'NONE',  ( -6.609253696060815031, -8.104785249476799791, -6.824425546749153249 ) ) ;
#69095=CARTESIAN_POINT ( 'NONE',  ( 0.1007326007325878847, -9.919999999999998153, 10.99953876047308476 ) ) ;
#69160=CARTESIAN_POINT ( 'NONE',  ( -0.003376046620579863274, -7.161464053357567749, -9.586610838029415049 ) ) ;
#69192=DIRECTION ( 'NONE',  ( 0.000000000000000000, 0.000000000000000000, 1.000000000000000000 ) ) ;
#69201=CARTESIAN_POINT ( 'NONE',  ( 8.581532217057311840, 3.975933801733725126, 7.726846314510468439 ) ) ;
#69226=CARTESIAN_POINT ( 'NONE',  ( -0.09916492693102199607, -10.00000000000016520, -9.499482423651642193 ) ) ;
#69266=SURFACE_STYLE_USAGE ( .BOTH. , #3195 ) ;
#69287=( GEOMETRIC_REPRESENTATION_CONTEXT ( 3 ) GLOBAL_UNCERTAINTY_ASSIGNED_CONTEXT ( ( #147905 ) ) GLOBAL_UNIT_ASSIGNED_CONTEXT ( ( #51279, #2486, #165019 ) ) REPRESENTATION_CONTEXT ( 'NONE', 'WORKASPACE' ) );
#69290=CARTESIAN_POINT ( 'NONE',  ( 7.654042494670958593E-16, 0.9200000000000041478, -6.250000000000000000 ) ) ;
#69310=DIRECTION ( 'NONE',  ( 0.000000000000000000, 0.000000000000000000, 1.000000000000000000 ) ) ;
#69312=VERTEX_POINT ( 'NONE', #102051 ) ;
#69313=CARTESIAN_POINT ( 'NONE',  ( -5.223082171297989432E-15, -6.148216694138040950, 10.67870335800436798 ) ) ;
#69322=ORIENTED_EDGE ( 'NONE', *, *, #121638, .F. ) ;
#69340=CARTESIAN_POINT ( 'NONE',  ( 0.000000000000000000, 1.000000000000000888, 0.000000000000000000 ) ) ;
#69344=LINE ( 'NONE', #135455, #163418 ) ;
#69379=CARTESIAN_POINT ( 'NONE',  ( -7.015831072854292749, -6.604036961759870650, 6.576431128232877121 ) ) ;
#69381=CARTESIAN_POINT ( 'NONE',  ( -8.673617379884035472E-15, -6.268611901546719878, -10.55819884875826453 ) ) ;
#69396=ORIENTED_EDGE ( 'NONE', *, *, #197437, .T. ) ;
#69438=CARTESIAN_POINT ( 'NONE',  ( 9.497898427948536337, -9.431315562283165477, -0.2398643602167310762 ) ) ;
#69453=AXIS2_PLACEMENT_3D ( 'NONE', #142230, #15103, #156326 ) ;
#69467=CARTESIAN_POINT ( 'NONE',  ( -8.846456096353129794, 0.9706168436483477713, -7.965384846859585366 ) ) ;
#69511=CARTESIAN_POINT ( 'NONE',  ( -6.594971851908696614, -6.631671897293978546, -6.818239719371401719 ) ) ;
#69519=CIRCLE ( 'NONE', #90278, 11.49999999999998934 ) ;
#69570=CARTESIAN_POINT ( 'NONE',  ( -9.499984059629559496, -7.809931833644718324, -0.02724524595755116463 ) ) ;
#69595=B_SPLINE_CURVE_WITH_KNOTS ( 'NONE', 3,
 ( #150588, #70354, #187327, #105039, #185182, #54141 ),
 .UNSPECIFIED., .F., .F.,
 ( 4, 2, 4 ),
 ( 0.000000000000000000, 0.001226111284895916318, 0.002452222569791832202 ),
 .UNSPECIFIED. ) ;
#69637=VERTEX_POINT ( 'NONE', #156148 ) ;
#69647=ADVANCED_FACE ( 'NONE', ( #7730 ), #167329, .T. ) ;
#69648=DIRECTION ( 'NONE',  ( 0.000000000000000000, 0.000000000000000000, 1.000000000000000000 ) ) ;
#69664=DIRECTION ( 'NONE',  ( 0.000000000000000000, 0.000000000000000000, 1.000000000000000000 ) ) ;
#69677=ORIENTED_EDGE ( 'NONE', *, *, #159645, .T. ) ;
#69683=CARTESIAN_POINT ( 'NONE',  ( 0.07801928546527701902, -7.184999792974072541, -9.499679989893801135 ) ) ;
#69693=CARTESIAN_POINT ( 'NONE',  ( 9.549638505170030101, -6.527411821100059797, -0.4330238300980903676 ) ) ;
#69701=CARTESIAN_POINT ( 'NONE',  ( 0.000000000000000000, 0.000000000000000000, 0.000000000000000000 ) ) ;
#69711=CIRCLE ( 'NONE', #571, 10.99999999999999112 ) ;
#69758=CARTESIAN_POINT ( 'NONE',  ( -0.06814526087293248935, -6.511064858252400889, -10.88932262995847822 ) ) ;
#69776=CARTESIAN_POINT ( 'NONE',  ( 9.491250020638661411, -6.775781654326489267, -0.2167848519283618325 ) ) ;
#69779=ORIENTED_EDGE ( 'NONE', *, *, #28627, .F. ) ;
#69785=ORIENTED_EDGE ( 'NONE', *, *, #207315, .T. ) ;
#69792=CARTESIAN_POINT ( 'NONE',  ( 7.002681350352349732, -8.176227052203545398, -6.455298931196944423 ) ) ;
#69919=ORIENTED_EDGE ( 'NONE', *, *, #177065, .T. ) ;
#69925=EDGE_CURVE ( 'NONE', #7438, #107724, #83750, .T. ) ;
#69934=CARTESIAN_POINT ( 'NONE',  ( -10.43625799253330122, 3.019799309333212722, 6.025376361321555407 ) ) ;
#69961=CARTESIAN_POINT ( 'NONE',  ( 0.07933194154487849259, -9.900000000000005684, 9.499668754385625746 ) ) ;
#69963=AXIS2_PLACEMENT_3D ( 'NONE', #149727, #50094, #162787 ) ;
#69985=CARTESIAN_POINT ( 'NONE',  ( -0.4630894006623515469, -6.442483420144702322, -11.24798772015292769 ) ) ;
#70011=CARTESIAN_POINT ( 'NONE',  ( 0.4355862708379926174, -6.583980363595115293, 9.606148981167594414 ) ) ;
#70046=CIRCLE ( 'NONE', #83834, 0.08000000000000050127 ) ;
#70099=( BOUNDED_SURFACE ( )  B_SPLINE_SURFACE ( 3, 2, ( 
 ( #164131, #16773, #181422 ),
 ( #115431, #1578, #97016 ),
 ( #148933, #196623, #15715 ),
 ( #132716, #81800, #147883 ) ),
 .UNSPECIFIED., .F., .F., .T. ) 
 B_SPLINE_SURFACE_WITH_KNOTS ( ( 4, 4 ),
 ( 3, 3 ),
 ( 0.01090155471707265726, 0.01336979040894267258 ),
 ( 0.000000000000000000, 1.000000000000000000 ),
 .UNSPECIFIED. ) 
 GEOMETRIC_REPRESENTATION_ITEM ( )  RATIONAL_B_SPLINE_SURFACE ( (
 ( 1.000000000000000000, 0.6967468848055777819, 1.000000000000000000),
 ( 1.000000000000000000, 0.6961913616436821162, 1.000000000000000000),
 ( 1.000000000000000000, 0.6955505937926295124, 1.000000000000000000),
 ( 1.000000000000000000, 0.6947640035364029965, 1.000000000000000000) ) ) 
 REPRESENTATION_ITEM ( '' )  SURFACE ( )  );
#70103=B_SPLINE_CURVE_WITH_KNOTS ( 'NONE', 3,
 ( #78251, #128170, #177902, #210374 ),
 .UNSPECIFIED., .F., .F.,
 ( 4, 4 ),
 ( 0.000000000000000000, 0.0002909236271752606252 ),
 .UNSPECIFIED. ) ;
#70126=CARTESIAN_POINT ( 'NONE',  ( 0.000000000000000000, 3.079999999999999183, 6.250000000000000000 ) ) ;
#70159=ORIENTED_EDGE ( 'NONE', *, *, #143150, .F. ) ;
#70184=CARTESIAN_POINT ( 'NONE',  ( 0.3866913795912775842, 3.974415841077574285, -11.53480748357603858 ) ) ;
#70188=ORIENTED_EDGE ( 'NONE', *, *, #36376, .T. ) ;
#70263=EDGE_LOOP ( 'NONE', ( #136147, #185439, #21183 ) ) ;
#70317=CARTESIAN_POINT ( 'NONE',  ( 7.004500933659072892, -6.920331743269710678, 7.004500933659049799 ) ) ;
#70324=CARTESIAN_POINT ( 'NONE',  ( 0.4355862708379926174, -6.583980363595115293, 9.606148981167594414 ) ) ;
#70354=CARTESIAN_POINT ( 'NONE',  ( -10.39230484541328181, 3.038454817776199857, -5.999999999999975131 ) ) ;
#70421=VERTEX_POINT ( 'NONE', #154948 ) ;
#70426=AXIS2_PLACEMENT_3D ( 'NONE', #63878, #33507, #214339 ) ;
#70440=CARTESIAN_POINT ( 'NONE',  ( 7.836017471263539313, -5.361065518611640712, -7.720011280421980260 ) ) ;
#70444=EDGE_LOOP ( 'NONE', ( #49165, #171834, #143387, #134105 ) ) ;
#70497=CARTESIAN_POINT ( 'NONE',  ( 9.603221262331027575, -9.439766061754880866, -0.1988025308400224733 ) ) ;
#70499=CARTESIAN_POINT ( 'NONE',  ( -2.020417662918760016, 3.956598013261175772, 11.36521191596583336 ) ) ;
#70500=CARTESIAN_POINT ( 'NONE',  ( 6.392587740394330531, -6.532648833121157850, 6.999862025036990509 ) ) ;
#70503=DIRECTION ( 'NONE',  ( 0.000000000000000000, 0.000000000000000000, 1.000000000000000000 ) ) ;
#70511=CARTESIAN_POINT ( 'NONE',  ( 0.000000000000000000, -1.000000000000000888, 0.000000000000000000 ) ) ;
#70558=CARTESIAN_POINT ( 'NONE',  ( -0.1236583036082171405, 1.000000000000000888, 11.99936284241579898 ) ) ;
#70580=VECTOR ( 'NONE', #36443, 1000.000000000000000 ) ;
#70601=CARTESIAN_POINT ( 'NONE',  ( 6.457408393014330450, -6.713678229394961505, 6.956254272497509383 ) ) ;
#70688=CARTESIAN_POINT ( 'NONE',  ( 0.09999999999990051569, -10.00000000000009592, 10.91954211494245008 ) ) ;
#70725=CIRCLE ( 'NONE', #105422, 11.99999999999999112 ) ;
#70736=ORIENTED_EDGE ( 'NONE', *, *, #85807, .F. ) ;
#70740=CARTESIAN_POINT ( 'NONE',  ( 7.487360338304411833, -6.465328379374277290, 7.487360338304385188 ) ) ;
#70744=ORIENTED_EDGE ( 'NONE', *, *, #66045, .F. ) ;
#70761=ORIENTED_EDGE ( 'NONE', *, *, #80621, .F. ) ;
#70766=CARTESIAN_POINT ( 'NONE',  ( -6.777910281175750562, -7.189645481333823085, 6.776323679500811714 ) ) ;
#70782=MECHANICAL_DESIGN_GEOMETRIC_PRESENTATION_REPRESENTATION('',(#198792),#195290);
#70788=( LENGTH_UNIT ( ) NAMED_UNIT ( * ) SI_UNIT ( .MILLI., .METRE. ) );
#70790=DIRECTION ( 'NONE',  ( 1.000000000000000000, 0.000000000000000000, 0.000000000000000000 ) ) ;
#70808=CARTESIAN_POINT ( 'NONE',  ( 1.637338291174485510E-15, -6.530144695498204754, 11.00000000000000178 ) ) ;
#70812=DIRECTION ( 'NONE',  ( 0.000000000000000000, 1.000000000000000000, 0.000000000000000000 ) ) ;
#70817=EDGE_CURVE ( 'NONE', #66793, #9078, #124918, .T. ) ;
#70838=ORIENTED_EDGE ( 'NONE', *, *, #190098, .F. ) ;
#70852=CARTESIAN_POINT ( 'NONE',  ( 7.778383330260375317, -5.907420853759296264, 7.778383330260354001 ) ) ;
#70856=CARTESIAN_POINT ( 'NONE',  ( -6.457408393014387293, -6.713678229394907326, -6.956254272497591096 ) ) ;
#70890=CARTESIAN_POINT ( 'NONE',  ( -10.91804383151481339, -8.407420853759283830, 0.1905751639681794174 ) ) ;
#70925=B_SPLINE_CURVE_WITH_KNOTS ( 'NONE', 3,
 ( #141047, #5625, #203838, #91206, #21878, #172445, #57623 ),
 .UNSPECIFIED., .F., .F.,
 ( 4, 3, 4 ),
 ( 0.0001135037246152992285, 0.0006245292469112881514, 0.002007692286193846990 ),
 .UNSPECIFIED. ) ;
#70954=CARTESIAN_POINT ( 'NONE',  ( 10.48884024596648601, 1.000000000000000888, -5.608780650328974104 ) ) ;
#70997=ORIENTED_EDGE ( 'NONE', *, *, #78986, .F. ) ;
#71032=CARTESIAN_POINT ( 'NONE',  ( 10.91914056351824414, 3.934209603697785607, -3.813461610468072749 ) ) ;
#71054=CARTESIAN_POINT ( 'NONE',  ( 10.91005274787795720, -6.893137084989842123, -0.4659925305415656971 ) ) ;
#71077=CARTESIAN_POINT ( 'NONE',  ( -10.91962425643199808, -9.999999999999994671, 0.09058751758333691284 ) ) ;
#71084=CYLINDRICAL_SURFACE ( 'NONE', #202202, 0.09999999999999986677 ) ;
#71092=CARTESIAN_POINT ( 'NONE',  ( 2.425588855776289687, 2.974000657016989901, -11.41149836408899709 ) ) ;
#71109=VERTEX_POINT ( 'NONE', #62759 ) ;
#71111=CARTESIAN_POINT ( 'NONE',  ( -8.917737905728751358, 3.499999999999989342, -8.029567276306261547 ) ) ;
#71125=CARTESIAN_POINT ( 'NONE',  ( 11.41267819554179042, 3.447199233515649386, -3.708203932499494648 ) ) ;
#71185=( GEOMETRIC_REPRESENTATION_CONTEXT ( 3 ) GLOBAL_UNCERTAINTY_ASSIGNED_CONTEXT ( ( #5154 ) ) GLOBAL_UNIT_ASSIGNED_CONTEXT ( ( #1434, #85919, #4627 ) ) REPRESENTATION_CONTEXT ( 'NONE', 'WORKASPACE' ) );
#71222=AXIS2_PLACEMENT_3D ( 'NONE', #164300, #148060, #214068 ) ;
#71234=CARTESIAN_POINT ( 'NONE',  ( -9.578206935422372226, -9.900000000000074962, 0.1671882239537618997 ) ) ;
#71250=CIRCLE ( 'NONE', #192316, 0.07999999999999993228 ) ;
#71258=ORIENTED_EDGE ( 'NONE', *, *, #121971, .F. ) ;
#71276=DIRECTION ( 'NONE',  ( 0.8660254037844327124, 0.000000000000000000, -0.5000000000000102141 ) ) ;
#71295=CARTESIAN_POINT ( 'NONE',  ( -0.2167848519283963049, -6.775781654326366699, -9.491250020638732465 ) ) ;
#71316=LINE ( 'NONE', #101708, #139012 ) ;
#71330=VERTEX_POINT ( 'NONE', #213266 ) ;
#71360=CARTESIAN_POINT ( 'NONE',  ( 9.579665964948882007, -7.325744180092283564, 1.734723475976807094E-15 ) ) ;
#71377=CARTESIAN_POINT ( 'NONE',  ( -6.595517585942705985, -7.896420114628011078, -7.253242555595321939 ) ) ;
#71382=CIRCLE ( 'NONE', #185652, 0.08000000000000020983 ) ;
#71478=SURFACE_SIDE_STYLE ('',( #119249 ) ) ;
#71479=CARTESIAN_POINT ( 'NONE',  ( -7.767011945534285644, -7.169578370797520250, 7.110792111438891894 ) ) ;
#71480=CARTESIAN_POINT ( 'NONE',  ( 6.549078289569722600, -6.948428148671506932, 6.549078289569701283 ) ) ;
#71514=CARTESIAN_POINT ( 'NONE',  ( 7.770158002575686673, -5.767087321558989288, -7.786489011998996901 ) ) ;
#71579=CARTESIAN_POINT ( 'NONE',  ( -10.91970695577495931, -6.134628647623513231, 0.000000000000000000 ) ) ;
#71598=CARTESIAN_POINT ( 'NONE',  ( -6.766604819867126253, -7.256397064628592020, 6.766604819867148457 ) ) ;
#71599=CARTESIAN_POINT ( 'NONE',  ( 0.000000000000000000, 0.000000000000000000, 0.000000000000000000 ) ) ;
#71601=CARTESIAN_POINT ( 'NONE',  ( -7.668547801473484249, -6.765616048178583419, -7.886602582589878452 ) ) ;
#71635=CARTESIAN_POINT ( 'NONE',  ( -10.91944002402978775, -9.999999999999994671, 0.1105873483556694958 ) ) ;
#71638=VERTEX_POINT ( 'NONE', #187176 ) ;
#71656=CARTESIAN_POINT ( 'NONE',  ( 6.663994888585877518, -7.154544010627095219, -6.770610912236881163 ) ) ;
#71781=VERTEX_POINT ( 'NONE', #6275 ) ;
#71794=ADVANCED_FACE ( 'NONE', ( #204470 ), #105990, .F. ) ;
#71880=FACE_OUTER_BOUND ( 'NONE', #100318, .T. ) ;
#71883=CARTESIAN_POINT ( 'NONE',  ( -9.617648866954029430, -9.063431457505044975, 0.6035590660249372519 ) ) ;
#71885=CARTESIAN_POINT ( 'NONE',  ( -2.276824562219559311E-15, -8.605993949662213538, -10.72098668450194303 ) ) ;
#71899=( BOUNDED_SURFACE ( )  B_SPLINE_SURFACE ( 3, 2, ( 
 ( #82901, #47246, #113360 ),
 ( #180418, #97062, #164174 ),
 ( #30987, #78640, #115475 ),
 ( #61340, #45114, #32036 ) ),
 .UNSPECIFIED., .F., .F., .T. ) 
 B_SPLINE_SURFACE_WITH_KNOTS ( ( 4, 4 ),
 ( 3, 3 ),
 ( 0.005330693667047291598, 0.008357081610771106145 ),
 ( 0.000000000000000000, 1.000000000000000000 ),
 .UNSPECIFIED. ) 
 GEOMETRIC_REPRESENTATION_ITEM ( )  RATIONAL_B_SPLINE_SURFACE ( (
 ( 1.000000000000000000, 0.7187737999613688089, 1.000000000000000000),
 ( 1.000000000000000000, 0.7186585579880990782, 1.000000000000000000),
 ( 1.000000000000000000, 0.7185467277397579178, 1.000000000000000000),
 ( 1.000000000000000000, 0.7184380228464051221, 1.000000000000000000) ) ) 
 REPRESENTATION_ITEM ( '' )  SURFACE ( )  );
#71962=DIRECTION ( 'NONE',  ( -8.881784197001252323E-16, 0.000000000000000000, 1.000000000000000000 ) ) ;
#71987=( LENGTH_UNIT ( ) NAMED_UNIT ( * ) SI_UNIT ( .MILLI., .METRE. ) );
#72018=PLANE ( 'NONE',  #175401 ) ;
#72057=ORIENTED_EDGE ( 'NONE', *, *, #954, .T. ) ;
#72060=EDGE_CURVE ( 'NONE', #76748, #183021, #130265, .T. ) ;
#72072=SURFACE_SIDE_STYLE ('',( #152287 ) ) ;
#72090=AXIS2_PLACEMENT_3D ( 'NONE', #188385, #9635, #108286 ) ;
#72113=PLANE ( 'NONE',  #186146 ) ;
#72148=EDGE_LOOP ( 'NONE', ( #122525, #117156, #43600, #44159 ) ) ;
#72180=ORIENTED_EDGE ( 'NONE', *, *, #121971, .T. ) ;
#72181=CARTESIAN_POINT ( 'NONE',  ( 9.496912337248827995, -9.201070920843591239, -0.2456386449429273644 ) ) ;
#72182=CIRCLE ( 'NONE', #179526, 0.08000000000000020983 ) ;
#72183=DIRECTION ( 'NONE',  ( 0.000000000000000000, 1.000000000000000000, 0.000000000000000000 ) ) ;
#72198=EDGE_CURVE ( 'NONE', #45106, #96541, #208750, .T. ) ;
#72234=CARTESIAN_POINT ( 'NONE',  ( -6.661184041420952440, -7.473374494058216300, 6.773376349083140013 ) ) ;
#72246=EDGE_LOOP ( 'NONE', ( #61535, #94561, #109755, #50406 ) ) ;
#72295=ORIENTED_EDGE ( 'NONE', *, *, #83213, .T. ) ;
#72309=FACE_OUTER_BOUND ( 'NONE', #150622, .T. ) ;
#72325=CARTESIAN_POINT ( 'NONE',  ( -7.147998200182420999E-13, 2.974000657017301652, -11.66643802584687251 ) ) ;
#72330=VERTEX_POINT ( 'NONE', #43100 ) ;
#72334=LINE ( 'NONE', #74497, #30442 ) ;
#72342=CARTESIAN_POINT ( 'NONE',  ( 0.000000000000000000, 4.000000000000003553, 0.000000000000000000 ) ) ;
#72347=DIRECTION ( 'NONE',  ( -1.000000000000000000, 0.000000000000000000, 0.000000000000000000 ) ) ;
#72358=CARTESIAN_POINT ( 'NONE',  ( -6.663994888585885512, -7.154544010627095219, 6.770610912236877610 ) ) ;
#72360=VECTOR ( 'NONE', #114328, 1000.000000000000227 ) ;
#72367=CARTESIAN_POINT ( 'NONE',  ( 1.337314304668908615E-15, -0.9200000000000041478, 10.91999999999999105 ) ) ;
#72387=CARTESIAN_POINT ( 'NONE',  ( -0.008694310353118022902, -8.101927612791783417, 11.00038155431018261 ) ) ;
#72444=TOROIDAL_SURFACE ( 'NONE', #82819, 10.92000000000000171, 0.08000000000000000167 ) ;
#72448=EDGE_CURVE ( 'NONE', #95548, #81487, #176853, .T. ) ;
#72452=CARTESIAN_POINT ( 'NONE',  ( 0.3183146091066056949, -6.808378554901781676, 10.86152993230179931 ) ) ;
#72492=VERTEX_POINT ( 'NONE', #148043 ) ;
#72520=ORIENTED_EDGE ( 'NONE', *, *, #190705, .T. ) ;
#72558=CARTESIAN_POINT ( 'NONE',  ( -8.002408263930261612, -6.836568542494980250, 7.346809171966449448 ) ) ;
#72585=CARTESIAN_POINT ( 'NONE',  ( -10.91944002402979130, -8.407420853759269619, 0.1105873483556677611 ) ) ;
#72592=CARTESIAN_POINT ( 'NONE',  ( 11.41267819554179042, 3.447199233515649386, -3.708203932499494648 ) ) ;
#72609=VERTEX_POINT ( 'NONE', #81958 ) ;
#72624=VECTOR ( 'NONE', #91924, 1000.000000000000114 ) ;
#72626=DIRECTION ( 'NONE',  ( 0.7071067811865462405, 0.000000000000000000, -0.7071067811865489050 ) ) ;
#72634=B_SPLINE_CURVE_WITH_KNOTS ( 'NONE', 3,
 ( #59059, #120950, #8174, #171744, #123106, #7086, #23341, #204210, #24403, #75317, #155504, #187987, #205295, #73158, #140352, #141433 ),
 .UNSPECIFIED., .F., .F.,
 ( 4, 3, 3, 3, 3, 4 ),
 ( 0.000000000000000000, 4.416163517948683538E-06, 1.117787330549789718E-05, 1.792356377819956129E-05, 2.465171878521282939E-05, 3.136847552908501679E-05 ),
 .UNSPECIFIED. ) ;
#72671=EDGE_LOOP ( 'NONE', ( #138088, #78118, #158228, #130207, #62359, #10360, #156964, #203310, #47790, #206464, #88051, #128091, #74837, #145846, #66295, #190726, #213871, #52687, #76530, #91422, #163727, #77123, #170293, #174810 ) ) ;
#72680=CARTESIAN_POINT ( 'NONE',  ( 0.09280742163705514580, -9.178267117872108471, -9.499822780340156925 ) ) ;
#72683=CARTESIAN_POINT ( 'NONE',  ( -7.834948825496938163, -6.134628647623485698, -7.720982897393567690 ) ) ;
#72714=CARTESIAN_POINT ( 'NONE',  ( 7.055228938193936372, -8.176568542494910830, -6.396834479292718534 ) ) ;
#72716=DIRECTION ( 'NONE',  ( 0.000000000000000000, 1.000000000000000000, 0.000000000000000000 ) ) ;
#72727=CARTESIAN_POINT ( 'NONE',  ( 0.1007670162816190901, -8.052608368926284399, 9.499791922504430275 ) ) ;
#72755=CARTESIAN_POINT ( 'NONE',  ( 6.531918710723870092, -6.583723166013912831, 7.057683771862373945 ) ) ;
#72786=CARTESIAN_POINT ( 'NONE',  ( -0.08522810233021893556, -9.999176686163549377, -9.579508557966956772 ) ) ;
#72793=ORIENTED_EDGE ( 'NONE', *, *, #98152, .F. ) ;
#72805=AXIS2_PLACEMENT_3D ( 'NONE', #129594, #30961, #195581 ) ;
#72987=EDGE_LOOP ( 'NONE', ( #54245, #24887, #189145 ) ) ;
#72994=FACE_OUTER_BOUND ( 'NONE', #119214, .T. ) ;
#73011=COLOUR_RGB ( '', 0.72549020, 0.75294118, 0.79215686) ;
#73038=DIRECTION ( 'NONE',  ( 0.000000000000000000, 1.000000000000000000, 0.000000000000000000 ) ) ;
#73084=CARTESIAN_POINT ( 'NONE',  ( -9.579665964935227151, -7.246166700194470067, 0.000000000000000000 ) ) ;
#73158=CARTESIAN_POINT ( 'NONE',  ( -9.499734081922108331, -9.919612995835006330, 0.07111086427374822827 ) ) ;
#73160=AXIS2_PLACEMENT_3D ( 'NONE', #133125, #199123, #50767 ) ;
#73182=DIRECTION ( 'NONE',  ( 0.000000000000000000, -1.000000000000000000, 0.000000000000000000 ) ) ;
#73184=CARTESIAN_POINT ( 'NONE',  ( 0.000000000000000000, -7.246166700194011767, 9.579665964935665912 ) ) ;
#73189=ORIENTED_EDGE ( 'NONE', *, *, #166799, .T. ) ;
#73212=CARTESIAN_POINT ( 'NONE',  ( 8.919266336783559623, 2.972657967447078775, 7.510420563956574647 ) ) ;
#73230=CARTESIAN_POINT ( 'NONE',  ( -0.001745240643731549302, -9.900000000000005684, -0.09998476951563611825 ) ) ;
#73241=ORIENTED_EDGE ( 'NONE', *, *, #67862, .F. ) ;
#73296=CARTESIAN_POINT ( 'NONE',  ( -6.935047222998407257, -6.682123388833687727, 6.658747417465787244 ) ) ;
#73338=EDGE_CURVE ( 'NONE', #26009, #82080, #57668, .T. ) ;
#73428=SURFACE_STYLE_USAGE ( .BOTH. , #56127 ) ;
#73451=EDGE_CURVE ( 'NONE', #172976, #183133, #166224, .T. ) ;
#73458=CARTESIAN_POINT ( 'NONE',  ( -9.498763045327489607, -9.581505939640113212, 0.1791256580974910639 ) ) ;
#73538=VECTOR ( 'NONE', #120425, 1000.000000000000000 ) ;
#73547=DIRECTION ( 'NONE',  ( 0.000000000000000000, 0.000000000000000000, 1.000000000000000000 ) ) ;
#73592=CARTESIAN_POINT ( 'NONE',  ( -11.19002393767586589, 0.9691415390508402172, 4.042856490848052431 ) ) ;
#73595=ORIENTED_EDGE ( 'NONE', *, *, #4542, .F. ) ;
#73604=CARTESIAN_POINT ( 'NONE',  ( -10.23394195678222651, -9.091017468561377157, 0.1786341213272082673 ) ) ;
#73620=UNCERTAINTY_MEASURE_WITH_UNIT (LENGTH_MEASURE( 1.000000000000000082E-05 ), #75431, 'distance_accuracy_value', 'NONE');
#73623=CARTESIAN_POINT ( 'NONE',  ( -10.61081979358358041, -7.079050064870600067, 0.4638907948587486230 ) ) ;
#73672=VERTEX_POINT ( 'NONE', #36953 ) ;
#73701=CARTESIAN_POINT ( 'NONE',  ( 0.07802162204156329328, -7.185026885903937455, -9.499679971350921903 ) ) ;
#73712=CARTESIAN_POINT ( 'NONE',  ( -7.778383330260348671, -5.907420853759295376, 7.778383330260377981 ) ) ;
#73727=B_SPLINE_CURVE_WITH_KNOTS ( 'NONE', 3,
 ( #89163, #170381, #39325, #155217 ),
 .UNSPECIFIED., .F., .F.,
 ( 4, 4 ),
 ( 0.000000000000000000, 9.170750103614400562E-05 ),
 .UNSPECIFIED. ) ;
#73742=CARTESIAN_POINT ( 'NONE',  ( -5.199652918878400189E-15, 3.038454817776198968, -11.99999999999998579 ) ) ;
#73745=EDGE_CURVE ( 'NONE', #53448, #114068, #117209, .T. ) ;
#73749=VERTEX_POINT ( 'NONE', #202635 ) ;
#73818=CARTESIAN_POINT ( 'NONE',  ( -9.499679971350920127, -7.185026885903970317, -0.07802162204179896587 ) ) ;
#73835=CARTESIAN_POINT ( 'NONE',  ( 0.000000000000000000, 3.956598013261175772, 0.000000000000000000 ) ) ;
#73863=CIRCLE ( 'NONE', #46209, 10.99999999999999112 ) ;
#73867=CARTESIAN_POINT ( 'NONE',  ( -8.914213045750475573, 3.487142912321096855, -8.026393478126237824 ) ) ;
#73869=CARTESIAN_POINT ( 'NONE',  ( -10.91944002402978775, -9.900000000000005684, 0.1105873483556694958 ) ) ;
#73945=ORIENTED_EDGE ( 'NONE', *, *, #21894, .T. ) ;
#73946=EDGE_LOOP ( 'NONE', ( #171368, #35429, #74598, #68183, #190428, #28532, #8683, #167358, #47043, #155252, #201633, #45304, #33828, #161536, #114412, #77248, #183812, #123965, #46124, #165994, #8825, #112796, #31900, #35490, #193661, #25614, #53473, #204837 ) ) ;
#73977=EDGE_CURVE ( 'NONE', #69312, #37010, #202251, .T. ) ;
#73998=ORIENTED_EDGE ( 'NONE', *, *, #137674, .F. ) ;
#74003=CARTESIAN_POINT ( 'NONE',  ( -6.775479680898221169, -7.217880409000307473, 6.775479680898245149 ) ) ;
#74049=DIRECTION ( 'NONE',  ( 0.000000000000000000, 1.561251128379122346E-12, 1.000000000000000000 ) ) ;
#74051=FACE_OUTER_BOUND ( 'NONE', #90140, .T. ) ;
#74064=DIRECTION ( 'NONE',  ( 0.000000000000000000, 1.000000000000000000, 0.000000000000000000 ) ) ;
#74065=COLOUR_RGB ( '', 0.40784314, 0.44705882, 0.49803922) ;
#74073=DIRECTION ( 'NONE',  ( -0.04520447523801534445, 0.000000000000000000, 0.9989777552170296948 ) ) ;
#74075=ADVANCED_FACE ( 'NONE', ( #40474 ), #4715, .F. ) ;
#74092=ORIENTED_EDGE ( 'NONE', *, *, #204228, .T. ) ;
#74106=CARTESIAN_POINT ( 'NONE',  ( 0.1588444833727359340, -6.630981389236866086, 9.484513307599966581 ) ) ;
#74131=CARTESIAN_POINT ( 'NONE',  ( 7.777967379493318845, -9.999999999999994671, 7.664830294503448549 ) ) ;
#74152=ORIENTED_EDGE ( 'NONE', *, *, #62840, .F. ) ;
#74171=FACE_OUTER_BOUND ( 'NONE', #206682, .T. ) ;
#74185=CARTESIAN_POINT ( 'NONE',  ( 0.000000000000000000, 7.849261790823902629, 0.000000000000000000 ) ) ;
#74228=EDGE_LOOP ( 'NONE', ( #60932, #29354, #12640, #171493, #192050 ) ) ;
#74280=DIRECTION ( 'NONE',  ( 0.000000000000000000, 0.000000000000000000, -1.000000000000000000 ) ) ;
#74308=( LENGTH_UNIT ( ) NAMED_UNIT ( * ) SI_UNIT ( .MILLI., .METRE. ) );
#74327=DIRECTION ( 'NONE',  ( -0.9998476951563912696, 0.000000000000000000, 0.01745240643728004568 ) ) ;
#74349=VERTEX_POINT ( 'NONE', #36176 ) ;
#74351=CARTESIAN_POINT ( 'NONE',  ( -0.2680151545362914889, -6.654245765634851040, -10.99740610014212550 ) ) ;
#74361=ORIENTED_EDGE ( 'NONE', *, *, #134113, .T. ) ;
#74362=EDGE_LOOP ( 'NONE', ( #3214, #2889, #35224, #47842 ) ) ;
#74488=EDGE_LOOP ( 'NONE', ( #127888, #46263 ) ) ;
#74497=CARTESIAN_POINT ( 'NONE',  ( 9.578206935422253210, -9.825744180092243596, -0.1671882239536598425 ) ) ;
#74522=ADVANCED_FACE ( 'NONE', ( #102252 ), #190743, .T. ) ;
#74544=CARTESIAN_POINT ( 'NONE',  ( -9.495512617570035729, -9.134774474195801020, 0.2994571439533236235 ) ) ;
#74547=CARTESIAN_POINT ( 'NONE',  ( -0.2863826248021646981, -7.730039540835470291, 10.99644352130520097 ) ) ;
#74585=SURFACE_STYLE_USAGE ( .BOTH. , #159031 ) ;
#74592=DIRECTION ( 'NONE',  ( -0.000000000000000000, -1.000000000000000000, -0.000000000000000000 ) ) ;
#74598=ORIENTED_EDGE ( 'NONE', *, *, #146528, .T. ) ;
#74621=B_SPLINE_CURVE_WITH_KNOTS ( 'NONE', 3,
 ( #146844, #85000, #49326, #100189, #199804, #67649, #213910 ),
 .UNSPECIFIED., .F., .F.,
 ( 4, 3, 4 ),
 ( 0.0001932309589017193582, 0.0009000000022123051842, 0.002089081127711805118 ),
 .UNSPECIFIED. ) ;
#74626=PRESENTATION_STYLE_ASSIGNMENT (( #123473 ) ) ;
#74634=EDGE_LOOP ( 'NONE', ( #167008, #5692, #20566, #70736 ) ) ;
#74655=CARTESIAN_POINT ( 'NONE',  ( 0.000000000000000000, -0.02379966007286238305, 0.000000000000000000 ) ) ;
#74669=CARTESIAN_POINT ( 'NONE',  ( -0.08000000000000714873, -5.907420853759267843, 10.91970695577494865 ) ) ;
#74709=CARTESIAN_POINT ( 'NONE',  ( -7.884707905546937567, -7.003075417673640501, 7.228805602686603216 ) ) ;
#74717=CARTESIAN_POINT ( 'NONE',  ( 9.261794192842835116, -6.948429295162968700, 9.269928574751061333E-15 ) ) ;
#74746=DIRECTION ( 'NONE',  ( 0.000000000000000000, 0.000000000000000000, -1.000000000000000000 ) ) ;
#74765=ORIENTED_EDGE ( 'NONE', *, *, #3537, .T. ) ;
#74789=CARTESIAN_POINT ( 'NONE',  ( -1.734723475976807094E-15, -8.407420853759283830, -10.91970695577494332 ) ) ;
#74837=ORIENTED_EDGE ( 'NONE', *, *, #51769, .T. ) ;
#74846=ADVANCED_FACE ( 'NONE', ( #76156 ), #89095, .F. ) ;
#74862=EDGE_LOOP ( 'NONE', ( #163817, #97670, #163779, #55403 ) ) ;
#74902=VERTEX_POINT ( 'NONE', #49783 ) ;
#74903=DIRECTION ( 'NONE',  ( 0.000000000000000000, 0.000000000000000000, -1.000000000000000000 ) ) ;
#74912=CARTESIAN_POINT ( 'NONE',  ( 10.99970480911018100, -6.304485801116100241, 0.08058605610353185289 ) ) ;
#74915=DIRECTION ( 'NONE',  ( 0.000000000000000000, -1.000000000000000000, 0.000000000000000000 ) ) ;
#74926=STYLED_ITEM ( 'NONE', ( #60043 ), #196809 ) ;
#74930=CARTESIAN_POINT ( 'NONE',  ( -2.373851744317279522, 1.000000000000000888, 11.76285798163022100 ) ) ;
#74937=CARTESIAN_POINT ( 'NONE',  ( 7.712474369503314442, -6.289226506789199256, -7.712474369503347305 ) ) ;
#74942=VERTEX_POINT ( 'NONE', #35654 ) ;
#74967=VERTEX_POINT ( 'NONE', #33531 ) ;
#74995=VERTEX_POINT ( 'NONE', #132145 ) ;
#75005=ORIENTED_EDGE ( 'NONE', *, *, #115899, .F. ) ;
#75029=CYLINDRICAL_SURFACE ( 'NONE', #110319, 0.08000000000000020983 ) ;
#75043=EDGE_CURVE ( 'NONE', #107467, #190376, #17859, .T. ) ;
#75064=ADVANCED_FACE ( 'NONE', ( #50853 ), #121733, .T. ) ;
#75158=ORIENTED_EDGE ( 'NONE', *, *, #111631, .F. ) ;
#75184=CARTESIAN_POINT ( 'NONE',  ( 0.08058608058607655278, -9.900000000000005684, 10.99970480893082225 ) ) ;
#75218=ORIENTED_EDGE ( 'NONE', *, *, #55286, .T. ) ;
#75228=AXIS2_PLACEMENT_3D ( 'NONE', #104478, #103401, #173765 ) ;
#75233=CARTESIAN_POINT ( 'NONE',  ( -2.093795543908766543, 0.9691415390508352212, 11.71227324440729234 ) ) ;
#75266=FILL_AREA_STYLE_COLOUR ( '', #112725 ) ;
#75281=CIRCLE ( 'NONE', #9559, 0.08000000000000020983 ) ;
#75305=VERTEX_POINT ( 'NONE', #207416 ) ;
#75317=CARTESIAN_POINT ( 'NONE',  ( -9.499671278040539235, -9.915617081696053603, 0.07902916658837459696 ) ) ;
#75318=CARTESIAN_POINT ( 'NONE',  ( 0.000000000000000000, 15.50000000000019362, 0.000000000000000000 ) ) ;
#75342=EDGE_CURVE ( 'NONE', #113976, #201530, #90585, .T. ) ;
#75427=CARTESIAN_POINT ( 'NONE',  ( -9.521443730523930782, -8.144690279336726846, 0.3123298761244260313 ) ) ;
#75428=CARTESIAN_POINT ( 'NONE',  ( 9.498884434226638973, -9.954196546781650667, -0.1657939142878195604 ) ) ;
#75431=( LENGTH_UNIT ( ) NAMED_UNIT ( * ) SI_UNIT ( .MILLI., .METRE. ) );
#75473=CARTESIAN_POINT ( 'NONE',  ( 0.000000000000000000, -6.836568542494925182, 0.000000000000000000 ) ) ;
#75507=CARTESIAN_POINT ( 'NONE',  ( 6.234224025626348364, -6.938199013094628498, 6.849482339516216989 ) ) ;
#75519=CARTESIAN_POINT ( 'NONE',  ( 0.000000000000000000, -7.154544010627095219, 0.000000000000000000 ) ) ;
#75556=EDGE_CURVE ( 'NONE', #94442, #69312, #156555, .T. ) ;
#75560=CARTESIAN_POINT ( 'NONE',  ( -9.516020521605595306, -8.176244038173962281, 0.3909723190919960900 ) ) ;
#75568=CARTESIAN_POINT ( 'NONE',  ( 10.91910517057295316, -9.994362614652946064, -0.1236848126708652712 ) ) ;
#75573=CARTESIAN_POINT ( 'NONE',  ( -9.811039896441892338, -7.242250812739402299, 9.077051502758969193E-18 ) ) ;
#75579=CARTESIAN_POINT ( 'NONE',  ( -11.25751254300905480, -6.452016313277408877, 1.138412281109779656E-15 ) ) ;
#75606=DIRECTION ( 'NONE',  ( 0.000000000000000000, 1.000000000000000000, 0.000000000000000000 ) ) ;
#75630=MECHANICAL_DESIGN_GEOMETRIC_PRESENTATION_REPRESENTATION('',(#99744),#79023);
#75634=ORIENTED_EDGE ( 'NONE', *, *, #75639, .T. ) ;
#75639=EDGE_CURVE ( 'NONE', #74995, #139509, #107952, .T. ) ;
#75711=AXIS2_PLACEMENT_3D ( 'NONE', #113469, #130782, #143812 ) ;
#75773=CARTESIAN_POINT ( 'NONE',  ( -7.253242555595325491, -7.896420114627995979, 6.595517585942709538 ) ) ;
#75777=AXIS2_PLACEMENT_3D ( 'NONE', #158239, #9828, #206959 ) ;
#75782=DIRECTION ( 'NONE',  ( 0.8660254037844363761, 0.000000000000000000, -0.5000000000000041078 ) ) ;
#75787=CARTESIAN_POINT ( 'NONE',  ( -0.1833053738655555376, -5.341077028191798526, -10.96562622554679578 ) ) ;
#75798=DIRECTION ( 'NONE',  ( -0.06183953750877529965, 0.9962285034897226943, -0.06086575749408236480 ) ) ;
#75827=ORIENTED_EDGE ( 'NONE', *, *, #2635, .F. ) ;
#75844=DIRECTION ( 'NONE',  ( -0.8660254037844328234, 0.000000000000000000, 0.5000000000000102141 ) ) ;
#75924=CARTESIAN_POINT ( 'NONE',  ( -7.564733433744393665, -6.863455982311501558, -7.986233326679976763 ) ) ;
#75925=CARTESIAN_POINT ( 'NONE',  ( 7.439168848973995551, -6.893137084989842123, 8.103009739378016718 ) ) ;
#75929=PLANE ( 'NONE',  #182546 ) ;
#75937=CARTESIAN_POINT ( 'NONE',  ( -10.95855051086950027, -7.723431457505071762, 0.6286713519883972978 ) ) ;
#75946=CARTESIAN_POINT ( 'NONE',  ( -9.579603127937250662, -9.746166700193986898, 0.08720040834116031536 ) ) ;
#75969=CARTESIAN_POINT ( 'NONE',  ( 0.1298625177950013254, -9.252181021551010076, -9.620122301472909143 ) ) ;
#76042=CARTESIAN_POINT ( 'NONE',  ( 0.000000000000000000, 1.000000000000000888, 0.000000000000000000 ) ) ;
#76059=DIRECTION ( 'NONE',  ( 0.000000000000000000, 0.000000000000000000, 1.000000000000000000 ) ) ;
#76120=( NAMED_UNIT ( * ) SI_UNIT ( $, .STERADIAN. ) SOLID_ANGLE_UNIT ( ) );
#76156=FACE_OUTER_BOUND ( 'NONE', #146736, .T. ) ;
#76209=EDGE_LOOP ( 'NONE', ( #10544, #79825, #177334, #156550 ) ) ;
#76216=CARTESIAN_POINT ( 'NONE',  ( -9.611175950047638139, -6.604184692106415788, 0.3106162252735236162 ) ) ;
#76228=DIRECTION ( 'NONE',  ( 0.000000000000000000, 0.000000000000000000, 1.000000000000000000 ) ) ;
#76229=B_SPLINE_CURVE_WITH_KNOTS ( 'NONE', 3,
 ( #157985, #59392, #191509, #140688, #57268, #143891, #11697, #58331, #160094, #77771 ),
 .UNSPECIFIED., .F., .F.,
 ( 4, 2, 2, 2, 4 ),
 ( 2.453269466693580506E-18, 0.0002503535593264591516, 0.0005007071186529159180, 0.0007510606779793734976, 0.001001414237305831186 ),
 .UNSPECIFIED. ) ;
#76253=EDGE_CURVE ( 'NONE', #14247, #61589, #59942, .T. ) ;
#76278=ORIENTED_EDGE ( 'NONE', *, *, #33969, .F. ) ;
#76307=CYLINDRICAL_SURFACE ( 'NONE', #155669, 10.24999999999998934 ) ;
#76377=CARTESIAN_POINT ( 'NONE',  ( 6.781144757626058173, -7.161464053357574855, -6.776370306708051849 ) ) ;
#76437=ORIENTED_EDGE ( 'NONE', *, *, #54068, .F. ) ;
#76442=ADVANCED_FACE ( 'NONE', ( #131559 ), #35348, .F. ) ;
#76470=CARTESIAN_POINT ( 'NONE',  ( -1.020505294851980891E-14, -6.134628647623514119, -11.00029519899099029 ) ) ;
#76481=CARTESIAN_POINT ( 'NONE',  ( -9.549252947205625119, -7.850763007174473174, 0.06856108760742210539 ) ) ;
#76514=CARTESIAN_POINT ( 'NONE',  ( -8.948250016579809341, 1.813773193624685920, -7.995571895478096103 ) ) ;
#76530=ORIENTED_EDGE ( 'NONE', *, *, #31233, .T. ) ;
#76535=TOROIDAL_SURFACE ( 'NONE', #197594, 11.29999999999999893, 0.2000000000000000111 ) ;
#76540=CARTESIAN_POINT ( 'NONE',  ( 0.01492041558614315595, -9.953728265215222137, 10.91968477554610040 ) ) ;
#76565=CARTESIAN_POINT ( 'NONE',  ( -0.1000000000000080685, -9.999999999999994671, -10.91954211494235238 ) ) ;
#76587=AXIS2_PLACEMENT_3D ( 'NONE', #179045, #30663, #146565 ) ;
#76603=EDGE_LOOP ( 'NONE', ( #165740, #3968 ) ) ;
#76612=( BOUNDED_SURFACE ( )  B_SPLINE_SURFACE ( 3, 2, ( 
 ( #79438, #64262, #45894 ),
 ( #61056, #127215, #193183 ),
 ( #196395, #43766, #48038 ),
 ( #92523, #195331, #158562 ) ),
 .UNSPECIFIED., .F., .F., .T. ) 
 B_SPLINE_SURFACE_WITH_KNOTS ( ( 4, 4 ),
 ( 3, 3 ),
 ( 0.04893088146668655297, 0.05137248493452929027 ),
 ( 0.000000000000000000, 1.000000000000000000 ),
 .UNSPECIFIED. ) 
 GEOMETRIC_REPRESENTATION_ITEM ( )  RATIONAL_B_SPLINE_SURFACE ( (
 ( 1.000000000000000000, 0.7169884966214681299, 1.000000000000000000),
 ( 1.000000000000000000, 0.7174883642158070840, 1.000000000000000000),
 ( 1.000000000000000000, 0.7180610417773362064, 1.000000000000000000),
 ( 1.000000000000000000, 0.7187540717311200478, 1.000000000000000000) ) ) 
 REPRESENTATION_ITEM ( '' )  SURFACE ( )  );
#76645=AXIS2_PLACEMENT_3D ( 'NONE', #149419, #34593, #181895 ) ;
#76659=ADVANCED_FACE ( 'NONE', ( #21716 ), #88909, .T. ) ;
#76662=CARTESIAN_POINT ( 'NONE',  ( -9.486277548414619787, -9.200719317737794611, 0.5196196971346862536 ) ) ;
#76675=MECHANICAL_DESIGN_GEOMETRIC_PRESENTATION_REPRESENTATION('',(#21291),#194189);
#76707=B_SPLINE_CURVE_WITH_KNOTS ( 'NONE', 3,
 ( #12836, #32310, #180684, #162318 ),
 .UNSPECIFIED., .F., .F.,
 ( 4, 4 ),
 ( 0.000000000000000000, 0.0002908967400263831236 ),
 .UNSPECIFIED. ) ;
#76727=CARTESIAN_POINT ( 'NONE',  ( 10.99462144896566862, -5.166862915010297819, -0.3541067150203519587 ) ) ;
#76728=CARTESIAN_POINT ( 'NONE',  ( 0.3536970929471299763, -9.200718514870473541, -9.493915151247827922 ) ) ;
#76740=CYLINDRICAL_SURFACE ( 'NONE', #27531, 11.99999999999999112 ) ;
#76748=VERTEX_POINT ( 'NONE', #124677 ) ;
#76761=ORIENTED_EDGE ( 'NONE', *, *, #9358, .F. ) ;
#76769=CARTESIAN_POINT ( 'NONE',  ( 7.045261094876550167, -5.790678129197933011, 7.662794434365309826 ) ) ;
#76780=CARTESIAN_POINT ( 'NONE',  ( 0.000000000000000000, -13.99999999999999822, 6.249999999999995559 ) ) ;
#76784=CARTESIAN_POINT ( 'NONE',  ( -10.96384816988334343, 2.972657967447018823, 3.969100948795338812 ) ) ;
#76793=ADVANCED_FACE ( 'NONE', ( #59582 ), #142706, .T. ) ;
#76837=EDGE_CURVE ( 'NONE', #165149, #101925, #155466, .T. ) ;
#76853=CARTESIAN_POINT ( 'NONE',  ( -1.409462824231155764E-15, 2.018041202054154493, 12.16970660573693586 ) ) ;
#76877=VERTEX_POINT ( 'NONE', #122555 ) ;
#76880=CIRCLE ( 'NONE', #14711, 9.499999999999991118 ) ;
#76935=ORIENTED_EDGE ( 'NONE', *, *, #63311, .T. ) ;
#76946=CARTESIAN_POINT ( 'NONE',  ( 6.493979434129337314, -7.868711957284896030, 6.493979434129313333 ) ) ;
#76947=VECTOR ( 'NONE', #98621, 1000.000000000000000 ) ;
#76977=CARTESIAN_POINT ( 'NONE',  ( -7.503508839934899477, -6.893137084989717778, -8.043940816608035504 ) ) ;
#76978=CARTESIAN_POINT ( 'NONE',  ( 7.505515594164131166, -6.699677480914246530, 8.042162931143014504 ) ) ;
#76987=ORIENTED_EDGE ( 'NONE', *, *, #93999, .F. ) ;
#76991=CARTESIAN_POINT ( 'NONE',  ( -10.99039737178640408, -7.697079954928536694, 0.4645147939555879235 ) ) ;
#77036=CIRCLE ( 'NONE', #135808, 0.07999999999999991840 ) ;
#77053=CARTESIAN_POINT ( 'NONE',  ( -7.624693973552363779, -5.341768514962208059, -7.882977371601961991 ) ) ;
#77056=ORIENTED_EDGE ( 'NONE', *, *, #137134, .T. ) ;
#77076=CARTESIAN_POINT ( 'NONE',  ( 6.773376349083131132, -7.246166700180801001, 6.661184041420955992 ) ) ;
#77083=( BOUNDED_SURFACE ( )  B_SPLINE_SURFACE ( 3, 2, ( 
 ( #19397, #85477, #172885 ),
 ( #7141, #151564, #3131 ),
 ( #119111, #9298, #73212 ),
 ( #189116, #69201, #141485 ) ),
 .UNSPECIFIED., .F., .F., .T. ) 
 B_SPLINE_SURFACE_WITH_KNOTS ( ( 4, 4 ),
 ( 3, 3 ),
 ( 0.005313560486515473899, 0.008339948430246690511 ),
 ( 0.000000000000000000, 1.000000000000000000 ),
 .UNSPECIFIED. ) 
 GEOMETRIC_REPRESENTATION_ITEM ( )  RATIONAL_B_SPLINE_SURFACE ( (
 ( 1.000000000000000000, 0.7184380228464071205, 1.000000000000000000),
 ( 1.000000000000000000, 0.7185467277397563635, 1.000000000000000000),
 ( 1.000000000000000000, 0.7186585579881024088, 1.000000000000000000),
 ( 1.000000000000000000, 0.7187737999613684758, 1.000000000000000000) ) ) 
 REPRESENTATION_ITEM ( '' )  SURFACE ( )  );
#77099=VECTOR ( 'NONE', #86781, 1000.000000000000000 ) ;
#77123=ORIENTED_EDGE ( 'NONE', *, *, #170125, .T. ) ;
#77138=ORIENTED_EDGE ( 'NONE', *, *, #107143, .T. ) ;
#77172=EDGE_LOOP ( 'NONE', ( #208295, #61968, #183967, #43965 ) ) ;
#77207=SURFACE_SIDE_STYLE ('',( #146517 ) ) ;
#77235=DIRECTION ( 'NONE',  ( 0.000000000000000000, -1.000000000000000000, 0.000000000000000000 ) ) ;
#77239=CARTESIAN_POINT ( 'NONE',  ( 0.09500528524172392741, -5.338246727548283665, 10.99984294789629935 ) ) ;
#77243=ADVANCED_FACE ( 'NONE', ( #206891 ), #170675, .T. ) ;
#77246=CARTESIAN_POINT ( 'NONE',  ( -9.579764304849156531, -9.999999999999994671, 0.06720017513374074158 ) ) ;
#77248=ORIENTED_EDGE ( 'NONE', *, *, #62637, .T. ) ;
#77257=CARTESIAN_POINT ( 'NONE',  ( -10.48884024596653397, 1.000000000000000888, 5.608780650328914597 ) ) ;
#77260=VERTEX_POINT ( 'NONE', #62772 ) ;
#77268=CIRCLE ( 'NONE', #11555, 0.08000000000000020983 ) ;
#77298=CARTESIAN_POINT ( 'NONE',  ( -0.08000000000000714873, -6.134628647623513231, 10.99970695577494872 ) ) ;
#77326=CARTESIAN_POINT ( 'NONE',  ( 9.579665964948885559, 7.849261790823902629, 0.07999999999999847511 ) ) ;
#77497=ORIENTED_EDGE ( 'NONE', *, *, #60250, .F. ) ;
#77512=EDGE_CURVE ( 'NONE', #167635, #131570, #208356, .T. ) ;
#77521=DIRECTION ( 'NONE',  ( -0.9999655912483514930, 0.000000000000000000, 0.008295560218253852924 ) ) ;
#77545=CARTESIAN_POINT ( 'NONE',  ( 0.000000000000000000, 3.956598013261175772, 0.000000000000000000 ) ) ;
#77554=FACE_OUTER_BOUND ( 'NONE', #149723, .T. ) ;
#77573=ORIENTED_EDGE ( 'NONE', *, *, #184656, .T. ) ;
#77609=CARTESIAN_POINT ( 'NONE',  ( 0.02191186323000256231, -9.962467934940974601, 10.91967397018795438 ) ) ;
#77615=PLANE ( 'NONE',  #57527 ) ;
#77660=EDGE_CURVE ( 'NONE', #14615, #160452, #17202, .T. ) ;
#77704=ORIENTED_EDGE ( 'NONE', *, *, #213278, .T. ) ;
#77731=CARTESIAN_POINT ( 'NONE',  ( -9.491602870538727643, -9.241975548351229364, 0.4178506376739494765 ) ) ;
#77763=EDGE_CURVE ( 'NONE', #160452, #160219, #13529, .T. ) ;
#77771=CARTESIAN_POINT ( 'NONE',  ( 7.834948825496932834, -5.907420853759296264, 7.720982897393586342 ) ) ;
#77795=CARTESIAN_POINT ( 'NONE',  ( 9.499668754385638181, -7.473374494045003757, 0.07933194154488365513 ) ) ;
#77857=AXIS2_PLACEMENT_3D ( 'NONE', #1065, #35716, #84471 ) ;
#77859=ORIENTED_EDGE ( 'NONE', *, *, #108140, .T. ) ;
#77872=( BOUNDED_SURFACE ( )  B_SPLINE_SURFACE ( 3, 2, ( 
 ( #133866, #1658, #199873 ),
 ( #42758, #38458, #41687 ),
 ( #191089, #90421, #104535 ),
 ( #186828, #154344, #190034 ),
 ( #106713, #24315, #156490 ),
 ( #6990, #137034, #105621 ),
 ( #170581, #89359, #26468 ),
 ( #39521, #107798, #9155 ) ),
 .UNSPECIFIED., .F., .F., .T. ) 
 B_SPLINE_SURFACE_WITH_KNOTS ( ( 4, 2, 2, 4 ),
 ( 3, 3 ),
 ( 0.000000000000000000, 0.0005109843281227146802, 0.0007664764921840720203, 0.001021968656245429360 ),
 ( 0.000000000000000000, 1.000000000000000000 ),
 .UNSPECIFIED. ) 
 GEOMETRIC_REPRESENTATION_ITEM ( )  RATIONAL_B_SPLINE_SURFACE ( (
 ( 1.000000000000000000, 0.7045118851637611757, 1.000000000000000000),
 ( 1.000000000000000000, 0.6478559580220908387, 1.000000000000000000),
 ( 1.000000000000000000, 0.5832506164448501007, 1.000000000000000000),
 ( 1.000000000000000000, 0.4879709628489244944, 1.000000000000000000),
 ( 1.000000000000000000, 0.4561823831825844722, 1.000000000000000000),
 ( 1.000000000000000000, 0.4039565156456113582, 1.000000000000000000),
 ( 1.000000000000000000, 0.3848936348730044310, 1.000000000000000000),
 ( 1.000000000000000000, 0.3826834323650832315, 1.000000000000000000) ) ) 
 REPRESENTATION_ITEM ( '' )  SURFACE ( )  );
#77890=DIRECTION ( 'NONE',  ( 0.000000000000000000, 1.000000000000000000, 0.000000000000000000 ) ) ;
#77910=VECTOR ( 'NONE', #83868, 1000.000000000000000 ) ;
#77924=CARTESIAN_POINT ( 'NONE',  ( -0.1796516426514560283, -8.073984524010633379, -9.498564853506501038 ) ) ;
#77927=CARTESIAN_POINT ( 'NONE',  ( 3.248783280693067424E-12, 2.974000657016963256, 11.66643802584408185 ) ) ;
#77932=CARTESIAN_POINT ( 'NONE',  ( -10.23127510237379667, 3.700502905159952949, 5.878152162067748598 ) ) ;
#77934=CYLINDRICAL_SURFACE ( 'NONE', #92615, 0.07999999999999993228 ) ;
#77941=CARTESIAN_POINT ( 'NONE',  ( -0.07933194154488883154, -7.473374494045017968, 9.499668754385636404 ) ) ;
#77994=DIRECTION ( 'NONE',  ( 0.000000000000000000, 0.000000000000000000, 1.000000000000000000 ) ) ;
#78000=CARTESIAN_POINT ( 'NONE',  ( -6.734029298721184276, -7.783114986501010080, -6.778728372092619914 ) ) ;
#78020=CARTESIAN_POINT ( 'NONE',  ( 7.137427454243371550, -7.616807780282499607, 7.137427454242994074 ) ) ;
#78029=ADVANCED_FACE ( 'NONE', ( #26824 ), #174181, .T. ) ;
#78035=CARTESIAN_POINT ( 'NONE',  ( 0.000000000000000000, 4.000000000000003553, -11.49999999999998934 ) ) ;
#78053=CARTESIAN_POINT ( 'NONE',  ( 6.808607288253659462, -8.010031549403118234, -6.625366561259649956 ) ) ;
#78056=CARTESIAN_POINT ( 'NONE',  ( 0.000000000000000000, 0.7999999999999951594, 0.000000000000000000 ) ) ;
#78062=ORIENTED_EDGE ( 'NONE', *, *, #111366, .T. ) ;
#78118=ORIENTED_EDGE ( 'NONE', *, *, #75556, .T. ) ;
#78144=CARTESIAN_POINT ( 'NONE',  ( 6.770610912236886492, -7.154544010627095219, 6.663994888585879295 ) ) ;
#78156=CARTESIAN_POINT ( 'NONE',  ( -9.578284150245952588, -9.932867526282002757, 0.1622940087187730029 ) ) ;
#78167=VECTOR ( 'NONE', #166138, 1000.000000000000000 ) ;
#78185=EDGE_CURVE ( 'NONE', #130351, #119003, #91865, .T. ) ;
#78199=VERTEX_POINT ( 'NONE', #158973 ) ;
#78205=EDGE_LOOP ( 'NONE', ( #187012, #126050, #163494, #202659 ) ) ;
#78251=CARTESIAN_POINT ( 'NONE',  ( -10.45358220256320436, 1.000000000000000888, 5.892590188894342162 ) ) ;
#78261=CARTESIAN_POINT ( 'NONE',  ( 7.548736457555743407, -7.034525084975653542, -7.548736457552916335 ) ) ;
#78273=CARTESIAN_POINT ( 'NONE',  ( -6.661184041420952440, -7.473374494058216300, 6.773376349083140013 ) ) ;
#78275=CARTESIAN_POINT ( 'NONE',  ( -1.734723475976807094E-15, -9.911192131523236526, -10.91970695577494332 ) ) ;
#78307=CARTESIAN_POINT ( 'NONE',  ( 0.03952929641551738982, -5.422159130394859972, 11.00000000000004974 ) ) ;
#78351=CARTESIAN_POINT ( 'NONE',  ( 0.08676667164121812381, -9.915770458193639669, 9.499603944220597285 ) ) ;
#78391=CARTESIAN_POINT ( 'NONE',  ( -7.552496594302674282, -5.254973434576990954, -7.962224162659105708 ) ) ;
#78399=CARTESIAN_POINT ( 'NONE',  ( -7.221001870987141302, -6.414086731524416329, 6.604641253243925370 ) ) ;
#78474=AXIS2_PLACEMENT_3D ( 'NONE', #116055, #203618, #51005 ) ;
#78480=EDGE_CURVE ( 'NONE', #81487, #74349, #207084, .T. ) ;
#78578=DIRECTION ( 'NONE',  ( -0.4999999999999978906, 0.000000000000000000, 0.8660254037844399289 ) ) ;
#78601=VERTEX_POINT ( 'NONE', #172023 ) ;
#78603=CARTESIAN_POINT ( 'NONE',  ( -0.3811408430856468854, -6.893136995914816545, -10.99374989157286819 ) ) ;
#78633=EDGE_LOOP ( 'NONE', ( #42923, #2362, #70188, #210250 ) ) ;
#78640=CARTESIAN_POINT ( 'NONE',  ( -10.20634067979475823, 1.972237431424362253, -5.892633538919750613 ) ) ;
#78644=CARTESIAN_POINT ( 'NONE',  ( -7.874499448206171870, -5.294771359305316061, 7.680942717881079851 ) ) ;
#78677=CARTESIAN_POINT ( 'NONE',  ( 0.000000000000000000, -9.919999999999998153, 0.000000000000000000 ) ) ;
#78734=EDGE_CURVE ( 'NONE', #138616, #204013, #124713, .T. ) ;
#78771=DIRECTION ( 'NONE',  ( 0.000000000000000000, 1.000000000000000000, 0.000000000000000000 ) ) ;
#78815=SURFACE_SIDE_STYLE ('',( #194706 ) ) ;
#78852=EDGE_CURVE ( 'NONE', #194558, #71109, #8382, .T. ) ;
#78858=( BOUNDED_SURFACE ( )  B_SPLINE_SURFACE ( 3, 2, ( 
 ( #166825, #33616, #153769 ),
 ( #133286, #120273, #168944 ),
 ( #186247, #20546, #152697 ),
 ( #170002, #84494, #87694 ) ),
 .UNSPECIFIED., .F., .F., .T. ) 
 B_SPLINE_SURFACE_WITH_KNOTS ( ( 4, 4 ),
 ( 3, 3 ),
 ( 0.01133669335851669041, 0.01377857026255017818 ),
 ( 0.000000000000000000, 1.000000000000000000 ),
 .UNSPECIFIED. ) 
 GEOMETRIC_REPRESENTATION_ITEM ( )  RATIONAL_B_SPLINE_SURFACE ( (
 ( 1.000000000000000000, 0.7169883299103952945, 1.000000000000000000),
 ( 1.000000000000000000, 0.7174882367753899759, 1.000000000000000000),
 ( 1.000000000000000000, 0.7180609655871071917, 1.000000000000000000),
 ( 1.000000000000000000, 0.7187540731122940008, 1.000000000000000000) ) ) 
 REPRESENTATION_ITEM ( '' )  SURFACE ( )  );
#78865=CARTESIAN_POINT ( 'NONE',  ( 6.775479680898270907, -7.217880409000325237, 6.775479680898254919 ) ) ;
#78905=CARTESIAN_POINT ( 'NONE',  ( 10.61081979358357863, -7.079050064870602732, -0.4638907948587486230 ) ) ;
#78925=EDGE_CURVE ( 'NONE', #119756, #93109, #103916, .T. ) ;
#78946=CARTESIAN_POINT ( 'NONE',  ( 0.4645846211130746917, -7.563986176625375535, 10.12536109763334302 ) ) ;
#78986=EDGE_CURVE ( 'NONE', #159016, #86684, #2970, .T. ) ;
#78995=DIRECTION ( 'NONE',  ( 0.000000000000000000, 0.000000000000000000, 1.000000000000000000 ) ) ;
#79023=( GEOMETRIC_REPRESENTATION_CONTEXT ( 3 ) GLOBAL_UNCERTAINTY_ASSIGNED_CONTEXT ( ( #179421 ) ) GLOBAL_UNIT_ASSIGNED_CONTEXT ( ( #83581, #133444, #117217 ) ) REPRESENTATION_CONTEXT ( 'NONE', 'WORKASPACE' ) );
#79026=ORIENTED_EDGE ( 'NONE', *, *, #152781, .F. ) ;
#79114=CARTESIAN_POINT ( 'NONE',  ( -7.806764249273705047, -6.480061791515693947, -7.750016138724921788 ) ) ;
#79144=CARTESIAN_POINT ( 'NONE',  ( -9.581975256308806976, -7.217880409008731846, -3.245988297567687842E-13 ) ) ;
#79196=CARTESIAN_POINT ( 'NONE',  ( -7.778383330260381534, -5.907420853759297152, -7.778383330260338901 ) ) ;
#79223=AXIS2_PLACEMENT_3D ( 'NONE', #12576, #144775, #80800 ) ;
#79229=CARTESIAN_POINT ( 'NONE',  ( 6.726126798029175902, -7.621055083280628750, 6.709229400514947095 ) ) ;
#79240=CIRCLE ( 'NONE', #13524, 9.523431457505068920 ) ;
#79296=DIRECTION ( 'NONE',  ( 0.08676574618400521854, 0.9962285034897236935, 0.0006885664517734813028 ) ) ;
#79322=CARTESIAN_POINT ( 'NONE',  ( 6.773376349083131132, -7.473374494058229622, 6.661184041420955992 ) ) ;
#79323=CARTESIAN_POINT ( 'NONE',  ( -7.317172100870442009, -6.705807707650950356, 7.317172100870468654 ) ) ;
#79326=CONICAL_SURFACE ( 'NONE', #114039, 11.53746066217573762, 0.1181278931043537039 ) ;
#79386=CARTESIAN_POINT ( 'NONE',  ( 1.347111479062088799E-15, -2.079999999999998295, -11.00000000000000178 ) ) ;
#79419=DIRECTION ( 'NONE',  ( 0.000000000000000000, 0.000000000000000000, 1.000000000000000000 ) ) ;
#79438=CARTESIAN_POINT ( 'NONE',  ( 7.987977580929889854, -5.530730635397379302, -7.987977580929920940 ) ) ;
#79451=B_SPLINE_CURVE_WITH_KNOTS ( 'NONE', 3,
 ( #104191, #21823, #2379, #87931, #68456, #200585, #52234, #118361, #57570, #41341, #143126, #205938, #91157, #6659, #125852, #157211 ),
 .UNSPECIFIED., .F., .F.,
 ( 4, 3, 3, 3, 3, 4 ),
 ( 0.000000000000000000, 6.763659418792604407E-06, 1.351747408346287881E-05, 2.025570936575418784E-05, 2.697948549281415037E-05, 3.136114954460948387E-05 ),
 .UNSPECIFIED. ) ;
#79470=CARTESIAN_POINT ( 'NONE',  ( -8.064677165291197269, -5.223431457505076203, 7.446209719563364082 ) ) ;
#79617=CARTESIAN_POINT ( 'NONE',  ( 0.000000000000000000, 0.2000000000000057288, 0.000000000000000000 ) ) ;
#79730=ORIENTED_EDGE ( 'NONE', *, *, #54696, .F. ) ;
#79747=FACE_OUTER_BOUND ( 'NONE', #6641, .T. ) ;
#79766=CARTESIAN_POINT ( 'NONE',  ( 6.999862025036645008, -6.532648833121171172, -6.392587740394702678 ) ) ;
#79807=ORIENTED_EDGE ( 'NONE', *, *, #95387, .T. ) ;
#79822=B_SPLINE_CURVE_WITH_KNOTS ( 'NONE', 3,
 ( #86590, #200319, #33574, #35698 ),
 .UNSPECIFIED., .F., .F.,
 ( 4, 4 ),
 ( 0.000000000000000000, 9.170750103614487298E-05 ),
 .UNSPECIFIED. ) ;
#79825=ORIENTED_EDGE ( 'NONE', *, *, #137160, .F. ) ;
#79831=FACE_BOUND ( 'NONE', #65514, .T. ) ;
#79883=( GEOMETRIC_REPRESENTATION_CONTEXT ( 3 ) GLOBAL_UNCERTAINTY_ASSIGNED_CONTEXT ( ( #155951 ) ) GLOBAL_UNIT_ASSIGNED_CONTEXT ( ( #39291, #188739, #108627 ) ) REPRESENTATION_CONTEXT ( 'NONE', 'WORKASPACE' ) );
#79889=EDGE_CURVE ( 'NONE', #45106, #58157, #211917, .T. ) ;
#79923=VECTOR ( 'NONE', #204018, 1000.000000000000000 ) ;
#79924=SURFACE_STYLE_USAGE ( .BOTH. , #96210 ) ;
#79928=LINE ( 'NONE', #30125, #91549 ) ;
#79941=ADVANCED_FACE ( 'NONE', ( #21525 ), #66550, .F. ) ;
#79943=CARTESIAN_POINT ( 'NONE',  ( 10.25877837909742318, 3.235871879154605057, -5.476282928277127482 ) ) ;
#79970=CARTESIAN_POINT ( 'NONE',  ( 0.000000000000000000, 3.447199233515649386, 12.00000000000000178 ) ) ;
#80057=DIRECTION ( 'NONE',  ( -0.9980789807931677027, -0.06195440338564740107, 0.000000000000000000 ) ) ;
#80059=( NAMED_UNIT ( * ) PLANE_ANGLE_UNIT ( ) SI_UNIT ( $, .RADIAN. ) );
#80129=AXIS2_PLACEMENT_3D ( 'NONE', #32006, #212863, #34118 ) ;
#80142=EDGE_LOOP ( 'NONE', ( #111775, #24924, #65416, #189531 ) ) ;
#80150=( BOUNDED_SURFACE ( )  B_SPLINE_SURFACE ( 3, 2, ( 
 ( #60813, #79196, #143183 ),
 ( #28314, #92288, #145311 ),
 ( #159380, #209174, #30461 ),
 ( #192932, #108568, #13118 ),
 ( #144254, #124833, #77053 ),
 ( #46721, #194003, #126974 ),
 ( #161532, #174595, #58685 ),
 ( #96546, #177776, #111769 ) ),
 .UNSPECIFIED., .F., .F., .T. ) 
 B_SPLINE_SURFACE_WITH_KNOTS ( ( 4, 2, 2, 4 ),
 ( 3, 3 ),
 ( 0.000000000000000000, 0.0004924884914732710617, 0.0007387327372099065925, 0.0009849769829465421234 ),
 ( 0.000000000000000000, 1.000000000000000000 ),
 .UNSPECIFIED. ) 
 GEOMETRIC_REPRESENTATION_ITEM ( )  RATIONAL_B_SPLINE_SURFACE ( (
 ( 1.000000000000000000, 0.7045118851637580670, 1.000000000000000000),
 ( 1.000000000000000000, 0.7593505504065410916, 1.000000000000000000),
 ( 1.000000000000000000, 0.8104906253031848307, 1.000000000000000000),
 ( 1.000000000000000000, 0.8722646935501724430, 1.000000000000000000),
 ( 1.000000000000000000, 0.8905178607894502774, 1.000000000000000000),
 ( 1.000000000000000000, 0.9170530604353909210, 1.000000000000000000),
 ( 1.000000000000000000, 0.9248184710077167470, 1.000000000000000000),
 ( 1.000000000000000000, 0.9238795325112880708, 1.000000000000000000) ) ) 
 REPRESENTATION_ITEM ( '' )  SURFACE ( )  );
#80182=CARTESIAN_POINT ( 'NONE',  ( 7.668547801473440728, -6.765616048178509701, 7.886602582589920196 ) ) ;
#80183=CARTESIAN_POINT ( 'NONE',  ( -0.4356160240586524068, -9.063431457505059186, 9.626717610576628559 ) ) ;
#80238=AXIS2_PLACEMENT_3D ( 'NONE', #76042, #142144, #89111 ) ;
#80255=SURFACE_STYLE_USAGE ( .BOTH. , #1108 ) ;
#80263=DIRECTION ( 'NONE',  ( 0.000000000000000000, 0.000000000000000000, 1.000000000000000000 ) ) ;
#80266=CARTESIAN_POINT ( 'NONE',  ( -0.03130284803980282887, -9.439835433791163410, 9.605218923937870912 ) ) ;
#80293=CARTESIAN_POINT ( 'NONE',  ( 6.773846765316628549, -7.473374494057231310, 6.773846765316613450 ) ) ;
#80297=CARTESIAN_POINT ( 'NONE',  ( 0.000000000000000000, -9.919999999999998153, 0.000000000000000000 ) ) ;
#80303=DIRECTION ( 'NONE',  ( -0.000000000000000000, 1.000000000000000000, -0.000000000000000000 ) ) ;
#80319=CARTESIAN_POINT ( 'NONE',  ( -7.721398836998370818, -5.827195405469540290, 7.721398836998400128 ) ) ;
#80384=CARTESIAN_POINT ( 'NONE',  ( 10.85717823004580218, -6.836271227032193032, -0.3852658704378455479 ) ) ;
#80394=SURFACE_STYLE_FILL_AREA ( #96678 ) ;
#80396=ADVANCED_FACE ( 'NONE', ( #72309 ), #85378, .T. ) ;
#80418=DIRECTION ( 'NONE',  ( 0.000000000000000000, 0.000000000000000000, -1.000000000000000000 ) ) ;
#80431=CARTESIAN_POINT ( 'NONE',  ( 0.03132844593996673976, -5.600264386820933638, 10.94526678918448681 ) ) ;
#80447=CARTESIAN_POINT ( 'NONE',  ( -6.772457744868586538, -7.185026885899632454, -6.662118508819935947 ) ) ;
#80448=EDGE_CURVE ( 'NONE', #19237, #201806, #4548, .T. ) ;
#80452=AXIS2_PLACEMENT_3D ( 'NONE', #144021, #32360, #61657 ) ;
#80481=EDGE_LOOP ( 'NONE', ( #117897, #210864, #63016, #24583 ) ) ;
#80491=ORIENTED_EDGE ( 'NONE', *, *, #41681, .T. ) ;
#80518=DIRECTION ( 'NONE',  ( -0.000000000000000000, -1.000000000000000000, -0.000000000000000000 ) ) ;
#80529=DIRECTION ( 'NONE',  ( 0.000000000000000000, 0.000000000000000000, 1.000000000000000000 ) ) ;
#80539=CARTESIAN_POINT ( 'NONE',  ( -7.461813752226491125, -6.074287852078599670, 6.844806938814765651 ) ) ;
#80621=EDGE_CURVE ( 'NONE', #119003, #50845, #132498, .T. ) ;
#80673=AXIS2_PLACEMENT_3D ( 'NONE', #22487, #6238, #37701 ) ;
#80718=VERTEX_POINT ( 'NONE', #156801 ) ;
#80737=VERTEX_POINT ( 'NONE', #159987 ) ;
#80750=EDGE_LOOP ( 'NONE', ( #98916, #153350, #155326, #44968 ) ) ;
#80758=AXIS2_PLACEMENT_3D ( 'NONE', #16931, #132877, #83011 ) ;
#80791=CARTESIAN_POINT ( 'NONE',  ( -7.721398836998370818, -5.907420853759296264, 7.721398836998400128 ) ) ;
#80800=DIRECTION ( 'NONE',  ( 0.000000000000000000, 0.000000000000000000, 1.000000000000000000 ) ) ;
#80827=CARTESIAN_POINT ( 'NONE',  ( -7.960263458454529761, -6.452016313277124659, -7.960263458454494234 ) ) ;
#80880=CARTESIAN_POINT ( 'NONE',  ( 7.720982897393566802, -9.999999999999994671, -7.834948825496929281 ) ) ;
#80895=EDGE_LOOP ( 'NONE', ( #8792, #57282, #7477, #10037, #59188 ) ) ;
#80907=SURFACE_SIDE_STYLE ('',( #62515 ) ) ;
#80971=ADVANCED_FACE ( 'NONE', ( #43062, #175188 ), #7307, .T. ) ;
#80978=ADVANCED_FACE ( 'NONE', ( #114503 ), #56168, .F. ) ;
#80996=CARTESIAN_POINT ( 'NONE',  ( 10.99620347397582698, -6.863457517656843088, -0.2978015046999226700 ) ) ;
#81040=CARTESIAN_POINT ( 'NONE',  ( -0.08058608058608254798, -8.407420853759283830, -10.99970480893080804 ) ) ;
#81045=FILL_AREA_STYLE ('',( #16013 ) ) ;
#81046=DIRECTION ( 'NONE',  ( 0.000000000000000000, -1.000000000000000000, 0.000000000000000000 ) ) ;
#81064=ORIENTED_EDGE ( 'NONE', *, *, #175600, .F. ) ;
#81102=FILL_AREA_STYLE_COLOUR ( '', #24928 ) ;
#81141=CARTESIAN_POINT ( 'NONE',  ( -9.260383576709818598, -9.448429295179884946, 0.1616405965916382914 ) ) ;
#81146=CARTESIAN_POINT ( 'NONE',  ( 0.2943368945748013332, -8.203192640252304102, 9.495705940876563389 ) ) ;
#81153=DIRECTION ( 'NONE',  ( 0.000000000000000000, 0.000000000000000000, 1.000000000000000000 ) ) ;
#81182=COLOUR_RGB ( '', 0.66274510, 0.83137255, 0.94901961) ;
#81219=CARTESIAN_POINT ( 'NONE',  ( 6.901817408925516872, -6.554751161430712791, -6.500815859343259895 ) ) ;
#81253=CARTESIAN_POINT ( 'NONE',  ( 0.03749947599223481948, -9.978860283170366330, 9.579600585153697168 ) ) ;
#81257=ORIENTED_EDGE ( 'NONE', *, *, #140838, .F. ) ;
#81293=CARTESIAN_POINT ( 'NONE',  ( -0.03866526371284068064, -9.261493551422349313, 9.500000000000152767 ) ) ;
#81321=DIRECTION ( 'NONE',  ( 0.000000000000000000, 1.000000000000000000, 0.000000000000000000 ) ) ;
#81359=CARTESIAN_POINT ( 'NONE',  ( 6.439526774796740405, -8.199734048663245289, 6.984891963203204490 ) ) ;
#81410=VERTEX_POINT ( 'NONE', #211690 ) ;
#81419=CARTESIAN_POINT ( 'NONE',  ( 9.860259297219576169, -8.821010173593821335, -0.6081441828345716116 ) ) ;
#81432=( BOUNDED_SURFACE ( )  B_SPLINE_SURFACE ( 3, 2, ( 
 ( #91706, #25592, #9354 ),
 ( #121059, #158814, #204317 ),
 ( #191287, #75428, #88487 ),
 ( #124268, #187026, #40810 ) ),
 .UNSPECIFIED., .F., .F., .T. ) 
 B_SPLINE_SURFACE_WITH_KNOTS ( ( 4, 4 ),
 ( 3, 3 ),
 ( 8.470329472543003391E-22, 3.124390317667046857E-05 ),
 ( 0.000000000000000000, 1.000000000000000000 ),
 .UNSPECIFIED. ) 
 GEOMETRIC_REPRESENTATION_ITEM ( )  RATIONAL_B_SPLINE_SURFACE ( (
 ( 1.000000000000000000, 0.7071067811861172503, 1.000000000000000000),
 ( 1.000000000000000000, 0.7090998123827566557, 1.000000000000000000),
 ( 1.000000000000000000, 0.7100789167762185938, 1.000000000000000000),
 ( 1.000000000000000000, 0.7100530722022274643, 1.000000000000000000) ) ) 
 REPRESENTATION_ITEM ( '' )  SURFACE ( )  );
#81433=CIRCLE ( 'NONE', #43417, 0.07999999999999993228 ) ;
#81437=ADVANCED_FACE ( 'NONE', ( #210635 ), #147788, .T. ) ;
#81469=CARTESIAN_POINT ( 'NONE',  ( 7.137427359598738086, -7.616807914308158622, -7.137427359597695364 ) ) ;
#81487=VERTEX_POINT ( 'NONE', #148839 ) ;
#81498=CARTESIAN_POINT ( 'NONE',  ( -1.063873381751401226E-14, -5.907420853759270507, 11.00029519899100094 ) ) ;
#81516=( BOUNDED_SURFACE ( )  B_SPLINE_SURFACE ( 3, 2, ( 
 ( #89746, #155795, #24704 ),
 ( #191468, #61484, #10587 ),
 ( #209845, #76662, #11658 ),
 ( #90806, #77731, #74544 ),
 ( #43133, #109249, #188274 ),
 ( #192533, #44187, #7379 ),
 ( #110307, #73458, #176315 ),
 ( #27919, #94015, #139560 ) ),
 .UNSPECIFIED., .F., .F., .T. ) 
 B_SPLINE_SURFACE_WITH_KNOTS ( ( 4, 2, 2, 4 ),
 ( 3, 3 ),
 ( 0.000000000000000000, 0.0002469787127373868161, 0.0004939574254747736322, 0.0009879148509495472644 ),
 ( 0.000000000000000000, 1.000000000000000000 ),
 .UNSPECIFIED. ) 
 GEOMETRIC_REPRESENTATION_ITEM ( )  RATIONAL_B_SPLINE_SURFACE ( (
 ( 1.000000000000000000, 0.3826834323650766811, 1.000000000000000000),
 ( 1.000000000000000000, 0.3798541548343959406, 1.000000000000000000),
 ( 1.000000000000000000, 0.3995981355978913130, 1.000000000000000000),
 ( 1.000000000000000000, 0.4556299950042939639, 1.000000000000000000),
 ( 1.000000000000000000, 0.4903550589607226229, 1.000000000000000000),
 ( 1.000000000000000000, 0.5915489574623006286, 1.000000000000000000),
 ( 1.000000000000000000, 0.6554239218402544420, 1.000000000000000000),
 ( 1.000000000000000000, 0.7100530722070637069, 1.000000000000000000) ) ) 
 REPRESENTATION_ITEM ( '' )  SURFACE ( )  );
#81591=CARTESIAN_POINT ( 'NONE',  ( -7.698131257602420341, -5.543994141378503215, -7.787098537122147945 ) ) ;
#81695=( BOUNDED_SURFACE ( )  B_SPLINE_SURFACE ( 3, 2, ( 
 ( #202551, #201484, #2211 ),
 ( #99750, #119259, #185245 ),
 ( #36867, #102951, #37952 ),
 ( #7559, #74717, #204686 ) ),
 .UNSPECIFIED., .F., .F., .F. ) 
 B_SPLINE_SURFACE_WITH_KNOTS ( ( 4, 4 ),
 ( 3, 3 ),
 ( 0.01133669335851671296, 0.01377857026255084431 ),
 ( 0.000000000000000000, 1.000000000000000000 ),
 .UNSPECIFIED. ) 
 GEOMETRIC_REPRESENTATION_ITEM ( )  RATIONAL_B_SPLINE_SURFACE ( (
 ( 1.000000000000000000, 0.7169883299103946284, 1.000000000000000000),
 ( 1.000000000000000000, 0.7174882367753905310, 1.000000000000000000),
 ( 1.000000000000000000, 0.7180609655871069696, 1.000000000000000000),
 ( 1.000000000000000000, 0.7187540731122941118, 1.000000000000000000) ) ) 
 REPRESENTATION_ITEM ( '' )  SURFACE ( )  );
#81699=ORIENTED_EDGE ( 'NONE', *, *, #32385, .F. ) ;
#81800=CARTESIAN_POINT ( 'NONE',  ( -2.303929616531696922E-15, -8.198316280121936472, 9.513083155459831630 ) ) ;
#81818=EDGE_CURVE ( 'NONE', #81410, #187130, #67550, .T. ) ;
#81844=CARTESIAN_POINT ( 'NONE',  ( -7.765925996254661179, -5.615420858948581895, 7.710915694720366531 ) ) ;
#81848=CARTESIAN_POINT ( 'NONE',  ( 11.00023563321887643, -5.575210796978345762, 0.04341786867414096363 ) ) ;
#81873=( GEOMETRIC_REPRESENTATION_CONTEXT ( 3 ) GLOBAL_UNCERTAINTY_ASSIGNED_CONTEXT ( ( #100553 ) ) GLOBAL_UNIT_ASSIGNED_CONTEXT ( ( #108866, #24318, #11281 ) ) REPRESENTATION_CONTEXT ( 'NONE', 'WORKASPACE' ) );
#81880=CARTESIAN_POINT ( 'NONE',  ( -9.611344009005486910, -6.731960136058444455, 0.1523027874135076676 ) ) ;
#81885=EDGE_CURVE ( 'NONE', #94238, #44666, #208659, .T. ) ;
#81958=CARTESIAN_POINT ( 'NONE',  ( 9.499700864329909678, -7.154544010627095219, 0.07538891330675402680 ) ) ;
#81962=CARTESIAN_POINT ( 'NONE',  ( -11.01272219801457375, 3.870433085555834651, 3.737564583532713591 ) ) ;
#82012=B_SPLINE_CURVE_WITH_KNOTS ( 'NONE', 3,
 ( #160981, #29917, #12572, #78644, #13643, #47250, #144770, #46178, #210780, #194531 ),
 .UNSPECIFIED., .F., .F.,
 ( 4, 2, 2, 2, 4 ),
 ( 0.000000000000000000, 0.0002503535593264583385, 0.0005007071186529166770, 0.0007510606779793750154, 0.001001414237305833354 ),
 .UNSPECIFIED. ) ;
#82018=AXIS2_PLACEMENT_3D ( 'NONE', #113421, #33157, #179427 ) ;
#82023=DIRECTION ( 'NONE',  ( 0.000000000000000000, 0.000000000000000000, -1.000000000000000000 ) ) ;
#82072=CARTESIAN_POINT ( 'NONE',  ( -0.08058608058609216529, -8.407420853759283830, -10.99970480893080271 ) ) ;
#82077=ORIENTED_EDGE ( 'NONE', *, *, #180435, .F. ) ;
#82080=VERTEX_POINT ( 'NONE', #206109 ) ;
#82094=CARTESIAN_POINT ( 'NONE',  ( -7.245729715095584389, -5.507058666270985725, -7.863746947443975621 ) ) ;
#82100=SURFACE_STYLE_FILL_AREA ( #81045 ) ;
#82163=CARTESIAN_POINT ( 'NONE',  ( -9.499606459999013097, -9.910930816046743530, 0.08647025586260563557 ) ) ;
#82186=FACE_OUTER_BOUND ( 'NONE', #185021, .T. ) ;
#82199=ADVANCED_FACE ( 'NONE', ( #171486 ), #25789, .F. ) ;
#82265=ORIENTED_EDGE ( 'NONE', *, *, #206395, .F. ) ;
#82280=ORIENTED_EDGE ( 'NONE', *, *, #117967, .F. ) ;
#82304=CARTESIAN_POINT ( 'NONE',  ( -6.773846765307993678, -7.473374494058229622, -6.773846765307958151 ) ) ;
#82307=CARTESIAN_POINT ( 'NONE',  ( 0.000000000000000000, -6.054403199333757257, 10.91970695577495931 ) ) ;
#82319=ORIENTED_EDGE ( 'NONE', *, *, #65507, .T. ) ;
#82327=SURFACE_SIDE_STYLE ('',( #176651 ) ) ;
#82376=CARTESIAN_POINT ( 'NONE',  ( -0.3387883092347166447, -5.166862915010296042, -10.99523224158953383 ) ) ;
#82385=( NAMED_UNIT ( * ) SI_UNIT ( $, .STERADIAN. ) SOLID_ANGLE_UNIT ( ) );
#82411=VERTEX_POINT ( 'NONE', #196278 ) ;
#82412=CARTESIAN_POINT ( 'NONE',  ( -9.578539647746888264, -9.962495449538964820, 0.1460552299441092994 ) ) ;
#82447=CARTESIAN_POINT ( 'NONE',  ( 6.979380938965668690, -8.233137084989705201, -6.445605026751793254 ) ) ;
#82463=VERTEX_POINT ( 'NONE', #11103 ) ;
#82472=CARTESIAN_POINT ( 'NONE',  ( 10.95855051086948251, -7.723431457505092190, -0.6286713519883923018 ) ) ;
#82507=B_SPLINE_CURVE_WITH_KNOTS ( 'NONE', 3,
 ( #82472, #134471, #2263, #133404, #15329, #81419, #68339 ),
 .UNSPECIFIED., .F., .F.,
 ( 4, 3, 4 ),
 ( 3.314949680324038239E-05, 0.0009000000012044577329, 0.001928999666871126280 ),
 .UNSPECIFIED. ) ;
#82512=PRESENTATION_STYLE_ASSIGNMENT (( #13255 ) ) ;
#82518=CARTESIAN_POINT ( 'NONE',  ( 7.709579522695849008, -6.700642373080283321, 7.846302513400023493 ) ) ;
#82527=VERTEX_POINT ( 'NONE', #94532 ) ;
#82531=EDGE_CURVE ( 'NONE', #135108, #128654, #53128, .T. ) ;
#82593=EDGE_CURVE ( 'NONE', #16465, #120494, #70103, .T. ) ;
#82693=DIRECTION ( 'NONE',  ( 0.000000000000000000, 0.000000000000000000, 1.000000000000000000 ) ) ;
#82694=SURFACE_STYLE_USAGE ( .BOTH. , #131507 ) ;
#82706=EDGE_LOOP ( 'NONE', ( #56489, #9931, #202598, #184102, #127164 ) ) ;
#82712=STYLED_ITEM ( 'NONE', ( #65683 ), #43581 ) ;
#82720=( BOUNDED_SURFACE ( )  B_SPLINE_SURFACE ( 3, 2, ( 
 ( #55150, #139623, #54086 ),
 ( #205646, #124502, #22621 ),
 ( #123446, #120222, #186196 ),
 ( #121297, #190461, #189408 ),
 ( #41050, #37829, #103907 ),
 ( #38898, #44242, #129825 ),
 ( #144960, #63671, #43188 ),
 ( #111425, #194729, #178497 ) ),
 .UNSPECIFIED., .F., .F., .T. ) 
 B_SPLINE_SURFACE_WITH_KNOTS ( ( 4, 2, 2, 4 ),
 ( 3, 3 ),
 ( 0.000000000000000000, 0.0002568729646053799498, 0.0005137459292107598996, 0.001027491858421519799 ),
 ( 0.000000000000000000, 1.000000000000000000 ),
 .UNSPECIFIED. ) 
 GEOMETRIC_REPRESENTATION_ITEM ( )  RATIONAL_B_SPLINE_SURFACE ( (
 ( 1.000000000000000000, 0.3826834323651039926, 1.000000000000000000),
 ( 1.000000000000000000, 0.3847114443833997699, 1.000000000000000000),
 ( 1.000000000000000000, 0.4039255759075961461, 1.000000000000000000),
 ( 1.000000000000000000, 0.4557194474495045444, 1.000000000000000000),
 ( 1.000000000000000000, 0.4874388927523756743, 1.000000000000000000),
 ( 1.000000000000000000, 0.5833547384516969414, 1.000000000000000000),
 ( 1.000000000000000000, 0.6470545345836524742, 1.000000000000000000),
 ( 1.000000000000000000, 0.7045118851637717228, 1.000000000000000000) ) ) 
 REPRESENTATION_ITEM ( '' )  SURFACE ( )  );
#82819=AXIS2_PLACEMENT_3D ( 'NONE', #186657, #23073, #140082 ) ;
#82832=ORIENTED_EDGE ( 'NONE', *, *, #12404, .T. ) ;
#82851=CARTESIAN_POINT ( 'NONE',  ( 9.609247538824295276, -6.583727468837977881, -0.3728355200474618991 ) ) ;
#82895=VERTEX_POINT ( 'NONE', #70500 ) ;
#82901=CARTESIAN_POINT ( 'NONE',  ( -10.33323920393396200, 4.021557182957058885, -5.965898435992030180 ) ) ;
#82904=CARTESIAN_POINT ( 'NONE',  ( 10.99976946526262900, -5.360092950639649523, -0.08269815893117112016 ) ) ;
#82925=CARTESIAN_POINT ( 'NONE',  ( -0.02903434592766130848, -5.609732095436329224, -10.94445979172680694 ) ) ;
#82936=CARTESIAN_POINT ( 'NONE',  ( -7.626074735689159390, -6.442483420751607959, -8.280982046698074583 ) ) ;
#82964=AXIS2_PLACEMENT_3D ( 'NONE', #190403, #75606, #108174 ) ;
#82989=CARTESIAN_POINT ( 'NONE',  ( 10.39230484541330135, 3.038454817776198968, 5.999999999999906741 ) ) ;
#83007=VERTEX_POINT ( 'NONE', #38040 ) ;
#83011=DIRECTION ( 'NONE',  ( 0.000000000000000000, 0.000000000000000000, 1.000000000000000000 ) ) ;
#83021=CARTESIAN_POINT ( 'NONE',  ( -1.013809028830076341E-14, -7.550885189219946447, -9.573337995800475397 ) ) ;
#83064=( GEOMETRIC_REPRESENTATION_CONTEXT ( 3 ) GLOBAL_UNCERTAINTY_ASSIGNED_CONTEXT ( ( #15737 ) ) GLOBAL_UNIT_ASSIGNED_CONTEXT ( ( #142410, #45963, #182320 ) ) REPRESENTATION_CONTEXT ( 'NONE', 'WORKASPACE' ) );
#83082=DIRECTION ( 'NONE',  ( 0.000000000000000000, -1.000000000000000000, 0.000000000000000000 ) ) ;
#83087=DIRECTION ( 'NONE',  ( 0.000000000000000000, 1.000000000000000000, 0.000000000000000000 ) ) ;
#83135=CARTESIAN_POINT ( 'NONE',  ( -0.08058608058609216529, -8.270571484000473816, -10.99970480893080271 ) ) ;
#83141=ORIENTED_EDGE ( 'NONE', *, *, #65438, .T. ) ;
#83172=AXIS2_PLACEMENT_3D ( 'NONE', #39776, #155659, #44861 ) ;
#83213=EDGE_CURVE ( 'NONE', #208229, #179210, #107366, .T. ) ;
#83253=DIRECTION ( 'NONE',  ( 0.000000000000000000, 0.000000000000000000, 1.000000000000000000 ) ) ;
#83257=DIRECTION ( 'NONE',  ( 0.000000000000000000, -1.000000000000000000, 0.000000000000000000 ) ) ;
#83307=DIRECTION ( 'NONE',  ( 0.000000000000000000, 1.000000000000000000, 0.000000000000000000 ) ) ;
#83370=PRODUCT_DEFINITION_FORMATION_WITH_SPECIFIED_SOURCE ( 'ANY', '', #92073, .NOT_KNOWN. ) ;
#83378=CARTESIAN_POINT ( 'NONE',  ( 10.99970480893080627, -9.999999999999994671, 0.08058608058608522640 ) ) ;
#83417=CARTESIAN_POINT ( 'NONE',  ( 0.000000000000000000, 0.2000000000000057288, 0.000000000000000000 ) ) ;
#83424=CARTESIAN_POINT ( 'NONE',  ( 0.000000000000000000, -7.723431457505077979, 0.000000000000000000 ) ) ;
#83442=FILL_AREA_STYLE ('',( #116013 ) ) ;
#83452=CARTESIAN_POINT ( 'NONE',  ( -2.331034670843834533E-15, -6.027819618361843546, 10.79920600060117941 ) ) ;
#83477=DIRECTION ( 'NONE',  ( 0.000000000000000000, 0.000000000000000000, -1.000000000000000000 ) ) ;
#83480=DIRECTION ( 'NONE',  ( 0.000000000000000000, 1.000000000000000000, 0.000000000000000000 ) ) ;
#83514=CARTESIAN_POINT ( 'NONE',  ( 6.661184041420940005, -7.473374494058216300, -6.773376349083132908 ) ) ;
#83523=ORIENTED_EDGE ( 'NONE', *, *, #136119, .F. ) ;
#83530=CARTESIAN_POINT ( 'NONE',  ( 10.02012520139314589, 1.794419290072776896, 6.231960695612015932 ) ) ;
#83534=CARTESIAN_POINT ( 'NONE',  ( 0.000000000000000000, -0.9200000000000041478, 0.000000000000000000 ) ) ;
#83566=ORIENTED_EDGE ( 'NONE', *, *, #187477, .F. ) ;
#83574=CARTESIAN_POINT ( 'NONE',  ( 9.617101990990372329, -9.241291349679091383, -0.3048231516917216388 ) ) ;
#83576=CARTESIAN_POINT ( 'NONE',  ( -2.157015650737198253, 3.934209603697780278, 11.36298392073394048 ) ) ;
#83581=( LENGTH_UNIT ( ) NAMED_UNIT ( * ) SI_UNIT ( .MILLI., .METRE. ) );
#83636=EDGE_LOOP ( 'NONE', ( #190634, #190286, #200641, #100172 ) ) ;
#83638=VERTEX_POINT ( 'NONE', #188944 ) ;
#83668=DIRECTION ( 'NONE',  ( 0.000000000000000000, 1.000000000000000000, 0.000000000000000000 ) ) ;
#83676=FACE_OUTER_BOUND ( 'NONE', #165466, .T. ) ;
#83679=CARTESIAN_POINT ( 'NONE',  ( 0.3175553531547097852, 3.956598013261177105, -11.53924059509142452 ) ) ;
#83734=ORIENTED_EDGE ( 'NONE', *, *, #108718, .T. ) ;
#83750=B_SPLINE_CURVE_WITH_KNOTS ( 'NONE', 3,
 ( #85670, #19597, #53175, #83530, #115043, #183172, #151756 ),
 .UNSPECIFIED., .F., .F.,
 ( 4, 3, 4 ),
 ( 0.000000000000000000, 0.0008000000000004423928, 0.002977368225425629754 ),
 .UNSPECIFIED. ) ;
#83761=CARTESIAN_POINT ( 'NONE',  ( 0.1007326007325003298, -10.00000000000001243, 10.99953876047307944 ) ) ;
#83782=DIRECTION ( 'NONE',  ( -0.000000000000000000, -1.000000000000000000, -0.000000000000000000 ) ) ;
#83804=CARTESIAN_POINT ( 'NONE',  ( -7.047292192037971859, -5.787795860784245683, -7.664865541498026680 ) ) ;
#83834=AXIS2_PLACEMENT_3D ( 'NONE', #140374, #24427, #206391 ) ;
#83837=VECTOR ( 'NONE', #50032, 1000.000000000000000 ) ;
#83868=DIRECTION ( 'NONE',  ( 0.1470157664651973450, 0.7071067811865536790, -0.6916548014802195166 ) ) ;
#83896=VECTOR ( 'NONE', #125218, 1000.000000000000114 ) ;
#83921=EDGE_CURVE ( 'NONE', #19237, #36083, #196341, .T. ) ;
#83929=CARTESIAN_POINT ( 'NONE',  ( 0.2663167167780124411, -9.037303891206541095, -9.496500708127754820 ) ) ;
#83966=CARTESIAN_POINT ( 'NONE',  ( 10.93220419382046416, -5.754340240174431464, -5.996486861200787814E-16 ) ) ;
#83980=CARTESIAN_POINT ( 'NONE',  ( 6.719405205105350554, -7.217450603038201962, -6.716119544744036496 ) ) ;
#83989=EDGE_CURVE ( 'NONE', #69637, #200355, #98138, .T. ) ;
#83990=CARTESIAN_POINT ( 'NONE',  ( 0.3388969742604112101, -7.666862915010149493, -10.99522790877599832 ) ) ;
#83999=B_SPLINE_CURVE_WITH_KNOTS ( 'NONE', 3,
 ( #115704, #181695, #165460, #48533, #32271, #79943, #50646 ),
 .UNSPECIFIED., .F., .F.,
 ( 4, 3, 4 ),
 ( 0.000000000000000000, 0.0008000000000004425012, 0.002977368225425631489 ),
 .UNSPECIFIED. ) ;
#84022=DIRECTION ( 'NONE',  ( 0.000000000000000000, 1.000000000000000000, 0.000000000000000000 ) ) ;
#84039=( BOUNDED_SURFACE ( )  B_SPLINE_SURFACE ( 3, 2, ( 
 ( #52504, #103392, #55702 ),
 ( #185688, #117570, #36239 ),
 ( #1589, #37317, #101248 ),
 ( #168391, #21039, #87137 ),
 ( #102317, #171584, #4778 ),
 ( #51450, #70856, #121857 ),
 ( #38388, #22098, #183565 ),
 ( #3716, #135901, #201919 ) ),
 .UNSPECIFIED., .F., .F., .T. ) 
 B_SPLINE_SURFACE_WITH_KNOTS ( ( 4, 2, 2, 4 ),
 ( 3, 3 ),
 ( 0.000000000000000000, 0.0004401918256853558494, 0.0006602877385280337200, 0.0008803836513707116989 ),
 ( 0.000000000000000000, 1.000000000000000000 ),
 .UNSPECIFIED. ) 
 GEOMETRIC_REPRESENTATION_ITEM ( )  RATIONAL_B_SPLINE_SURFACE ( (
 ( 1.000000000000000000, 0.6787756258918318242, 1.000000000000000000),
 ( 1.000000000000000000, 0.6284487096092253866, 1.000000000000000000),
 ( 1.000000000000000000, 0.5704014816693694367, 1.000000000000000000),
 ( 1.000000000000000000, 0.4882303283124204696, 1.000000000000000000),
 ( 1.000000000000000000, 0.4617370933882668504, 1.000000000000000000),
 ( 1.000000000000000000, 0.4222438920368297710, 1.000000000000000000),
 ( 1.000000000000000000, 0.4105126989449011665, 1.000000000000000000),
 ( 1.000000000000000000, 0.4127341956165110348, 1.000000000000000000) ) ) 
 REPRESENTATION_ITEM ( '' )  SURFACE ( )  );
#84054=( GEOMETRIC_REPRESENTATION_CONTEXT ( 3 ) GLOBAL_UNCERTAINTY_ASSIGNED_CONTEXT ( ( #28073 ) ) GLOBAL_UNIT_ASSIGNED_CONTEXT ( ( #48390, #112370, #165307 ) ) REPRESENTATION_CONTEXT ( 'NONE', 'WORKASPACE' ) );
#84066=ADVANCED_FACE ( 'NONE', ( #97878 ), #212210, .F. ) ;
#84079=CARTESIAN_POINT ( 'NONE',  ( 9.499668754396997983, -7.215568602690315636, 0.07933194018460217045 ) ) ;
#84110=EDGE_CURVE ( 'NONE', #103298, #65129, #69519, .T. ) ;
#84115=DIRECTION ( 'NONE',  ( 0.000000000000000000, 1.000000000000000000, 0.000000000000000000 ) ) ;
#84128=CARTESIAN_POINT ( 'NONE',  ( -7.952857047016746783, -6.836289462023503738, 7.401194801147176427 ) ) ;
#84141=MECHANICAL_DESIGN_GEOMETRIC_PRESENTATION_REPRESENTATION('',(#87697),#60019);
#84200=AXIS2_PLACEMENT_3D ( 'NONE', #28574, #80518, #213682 ) ;
#84243=CARTESIAN_POINT ( 'NONE',  ( 9.579764304849151202, -9.999999999999994671, -0.06720017513373727214 ) ) ;
#84306=CARTESIAN_POINT ( 'NONE',  ( -9.498884310698272770, -9.900000000000076739, 0.1658036423890281996 ) ) ;
#84324=CARTESIAN_POINT ( 'NONE',  ( -0.4683205530892509683, -8.233137084989849086, -9.568546172724143872 ) ) ;
#84326=FILL_AREA_STYLE_COLOUR ( '', #98487 ) ;
#84338=ORIENTED_EDGE ( 'NONE', *, *, #158865, .T. ) ;
#84357=CARTESIAN_POINT ( 'NONE',  ( -5.204170427930421283E-15, -7.126685749120009739, -9.926723642588084928 ) ) ;
#84382=CARTESIAN_POINT ( 'NONE',  ( -7.792125355486790639, -6.646943093533965730, 7.591565991045880146 ) ) ;
#84414=DIRECTION ( 'NONE',  ( -0.8660254037844362651, 0.000000000000000000, 0.5000000000000041078 ) ) ;
#84454=DIRECTION ( 'NONE',  ( 0.000000000000000000, 0.000000000000000000, 1.000000000000000000 ) ) ;
#84471=DIRECTION ( 'NONE',  ( 0.000000000000000000, 0.000000000000000000, 1.000000000000000000 ) ) ;
#84493=CARTESIAN_POINT ( 'NONE',  ( 10.87166355890667191, -6.717152734873750752, -0.1969747848976913240 ) ) ;
#84494=CARTESIAN_POINT ( 'NONE',  ( -1.138412281109779656E-15, -6.948429295162514840, -9.261794192843264995 ) ) ;
#84509=AXIS2_PLACEMENT_3D ( 'NONE', #34926, #186521, #6691 ) ;
#84524=CARTESIAN_POINT ( 'NONE',  ( -0.4294425147611466986, -9.199999999999988631, 9.490288674561783822 ) ) ;
#84554=CYLINDRICAL_SURFACE ( 'NONE', #63075, 6.249999999999995559 ) ;
#84608=ORIENTED_EDGE ( 'NONE', *, *, #202732, .F. ) ;
#84644=CARTESIAN_POINT ( 'NONE',  ( 9.590670562337447080, -9.593477663480472373, -0.1674057773689586193 ) ) ;
#84659=CARTESIAN_POINT ( 'NONE',  ( 0.000000000000000000, 15.50000000000019362, 0.000000000000000000 ) ) ;
#84669=CARTESIAN_POINT ( 'NONE',  ( 10.04957930738609839, 3.829867255648771618, 5.932860765075322007 ) ) ;
#84681=AXIS2_PLACEMENT_3D ( 'NONE', #65792, #114653, #131941 ) ;
#84754=DIRECTION ( 'NONE',  ( 0.000000000000000000, 0.000000000000000000, 1.000000000000000000 ) ) ;
#84756=CARTESIAN_POINT ( 'NONE',  ( 10.99949329275126253, -9.914220445327725173, -0.1055954338740888176 ) ) ;
#84782=ORIENTED_EDGE ( 'NONE', *, *, #165066, .F. ) ;
#84808=ORIENTED_EDGE ( 'NONE', *, *, #127713, .F. ) ;
#84824=CIRCLE ( 'NONE', #109182, 0.07999999999999993228 ) ;
#84878=CARTESIAN_POINT ( 'NONE',  ( 0.000000000000000000, -6.583980363594976737, 0.000000000000000000 ) ) ;
#84888=EDGE_LOOP ( 'NONE', ( #12127, #44472, #155303, #142134, #16181 ) ) ;
#84925=EDGE_CURVE ( 'NONE', #181416, #51191, #15053, .T. ) ;
#84945=CARTESIAN_POINT ( 'NONE',  ( 7.110792111438888341, -7.169578370797516698, 7.767011945534281203 ) ) ;
#84990=CARTESIAN_POINT ( 'NONE',  ( 6.785280070212259318, -6.896483513897647910, -6.645879322773438069 ) ) ;
#85000=CARTESIAN_POINT ( 'NONE',  ( -0.4358566159019752195, -8.896924251528570693, 9.793384314894463927 ) ) ;
#85011=DIRECTION ( 'NONE',  ( -0.000000000000000000, -1.000000000000000000, -0.000000000000000000 ) ) ;
#85038=CARTESIAN_POINT ( 'NONE',  ( 10.99126615174919053, -5.199999999999992184, -0.4382560683119160472 ) ) ;
#85141=EDGE_LOOP ( 'NONE', ( #40322, #142285, #153014, #93229, #126701 ) ) ;
#85162=CARTESIAN_POINT ( 'NONE',  ( 10.98633066092261323, -7.699791778944355514, -0.5535395452644623626 ) ) ;
#85179=CARTESIAN_POINT ( 'NONE',  ( -0.08000000000000714873, -9.999999999999994671, 10.99970695577494872 ) ) ;
#85196=CARTESIAN_POINT ( 'NONE',  ( 10.38614328979769041, 3.507114751586604129, 5.996442624206595795 ) ) ;
#85257=CARTESIAN_POINT ( 'NONE',  ( 10.99370838174331233, -6.893137084989840346, -0.3821126922044815744 ) ) ;
#85259=CARTESIAN_POINT ( 'NONE',  ( -9.606148981167452305, -6.583980363594983842, 0.4355862708380028314 ) ) ;
#85260=ORIENTED_EDGE ( 'NONE', *, *, #83213, .F. ) ;
#85264=CARTESIAN_POINT ( 'NONE',  ( -6.717278222822391953, -7.473374494058216300, 6.830415307812263137 ) ) ;
#85268=MECHANICAL_DESIGN_GEOMETRIC_PRESENTATION_REPRESENTATION('',(#74926),#81873);
#85311=CARTESIAN_POINT ( 'NONE',  ( 9.578932859269645661, -9.985077769980609474, -0.1209251627559674580 ) ) ;
#85334=ADVANCED_FACE ( 'NONE', ( #67487 ), #65942, .T. ) ;
#85378=CYLINDRICAL_SURFACE ( 'NONE', #163701, 0.08000000000000020983 ) ;
#85399=CARTESIAN_POINT ( 'NONE',  ( -7.720982897393583677, -6.134628647623485698, 7.834948825496934610 ) ) ;
#85411=EDGE_CURVE ( 'NONE', #157333, #178508, #172766, .T. ) ;
#85445=CARTESIAN_POINT ( 'NONE',  ( 8.845566791370190529, 3.603011019375345736, 7.955782632700100443 ) ) ;
#85477=CARTESIAN_POINT ( 'NONE',  ( 8.846456096353175980, 0.9706168436483472162, 7.965384846859531187 ) ) ;
#85507=ADVANCED_FACE ( 'NONE', ( #23013 ), #140022, .F. ) ;
#85518=CARTESIAN_POINT ( 'NONE',  ( 0.4265819271708388150, -6.701306620465361519, 10.99180900346492251 ) ) ;
#85532=CARTESIAN_POINT ( 'NONE',  ( -9.499606442108985860, -9.580649465752454574, 0.08647222121308685561 ) ) ;
#85540=SURFACE_STYLE_FILL_AREA ( #186230 ) ;
#85541=ORIENTED_EDGE ( 'NONE', *, *, #35731, .T. ) ;
#85556=CARTESIAN_POINT ( 'NONE',  ( 9.260383576709811493, -9.448429295179890275, -0.1616405965916348220 ) ) ;
#85584=DIRECTION ( 'NONE',  ( 0.000000000000000000, 1.000000000000000000, 0.000000000000000000 ) ) ;
#85586=CARTESIAN_POINT ( 'NONE',  ( -0.3536970929470897307, -9.200718514870397158, 9.493915151247904305 ) ) ;
#85616=CARTESIAN_POINT ( 'NONE',  ( -8.912450614902597934, 3.507114751586604129, -8.024806578263023127 ) ) ;
#85620=CARTESIAN_POINT ( 'NONE',  ( -10.91804383151480629, -9.900000000000005684, 0.1905751639681794174 ) ) ;
#85652=CARTESIAN_POINT ( 'NONE',  ( 7.761717428875247293, -5.600320323339640360, -7.717216217110713039 ) ) ;
#85670=CARTESIAN_POINT ( 'NONE',  ( 10.10176665042273392, 1.000000000000000888, 6.279211784079129721 ) ) ;
#85673=ORIENTED_EDGE ( 'NONE', *, *, #107653, .T. ) ;
#85714=EDGE_CURVE ( 'NONE', #102475, #183550, #17564, .T. ) ;
#85729=CARTESIAN_POINT ( 'NONE',  ( 0.3617799047494585918, -7.723163706540469242, -10.97113338213670808 ) ) ;
#85743=CARTESIAN_POINT ( 'NONE',  ( -7.346809171966848240, -6.836568542494916301, -8.002408263929963184 ) ) ;
#85744=AXIS2_PLACEMENT_3D ( 'NONE', #101515, #151349, #49561 ) ;
#85781=CARTESIAN_POINT ( 'NONE',  ( 0.4359508081057527629, -6.362962251423731175, 9.827407719474875236 ) ) ;
#85789=CARTESIAN_POINT ( 'NONE',  ( -6.770610912236888268, -7.154544010627095219, -6.663994888585867749 ) ) ;
#85795=CARTESIAN_POINT ( 'NONE',  ( -6.726126798029754106, -7.621055083280781517, -6.709229400517475739 ) ) ;
#85807=EDGE_CURVE ( 'NONE', #190182, #169714, #129655, .T. ) ;
#85823=EDGE_CURVE ( 'NONE', #50845, #119003, #157254, .T. ) ;
#85832=AXIS2_PLACEMENT_3D ( 'NONE', #205364, #56998, #123171 ) ;
#85853=ORIENTED_EDGE ( 'NONE', *, *, #190367, .F. ) ;
#85889=CARTESIAN_POINT ( 'NONE',  ( 6.484567079770447329, -6.583980363594976737, 7.100579091573052004 ) ) ;
#85897=B_SPLINE_CURVE_WITH_KNOTS ( 'NONE', 3,
 ( #32072, #164207, #128598, #81880, #180455, #147964, #144804, #63509 ),
 .UNSPECIFIED., .F., .F.,
 ( 4, 2, 2, 4 ),
 ( 0.000000000000000000, 0.0003954713701971478341, 0.0005932070552957217783, 0.0007909427403942956682 ),
 .UNSPECIFIED. ) ;
#85917=EDGE_LOOP ( 'NONE', ( #130528, #94894, #109271, #54787 ) ) ;
#85919=( NAMED_UNIT ( * ) PLANE_ANGLE_UNIT ( ) SI_UNIT ( $, .RADIAN. ) );
#85964=B_SPLINE_CURVE_WITH_KNOTS ( 'NONE', 3,
 ( #87959, #120539, #99945, #185443, #67406, #151902, #100996, #84756, #166010, #37063, #17595, #150843, #186516, #2405, #103145, #68484 ),
 .UNSPECIFIED., .F., .F.,
 ( 4, 3, 3, 3, 3, 4 ),
 ( 0.000000000000000000, 6.763659418792606948E-06, 1.351747408346288389E-05, 2.025570936575419461E-05, 2.697948549281416054E-05, 3.136114954460949742E-05 ),
 .UNSPECIFIED. ) ;
#85988=EDGE_CURVE ( 'NONE', #68165, #21223, #88135, .T. ) ;
#86005=FILL_AREA_STYLE ('',( #136901 ) ) ;
#86007=DIRECTION ( 'NONE',  ( 0.000000000000000000, -1.000000000000000000, 0.000000000000000000 ) ) ;
#86016=CARTESIAN_POINT ( 'NONE',  ( 2.093795543908758994, 0.9691415390508362204, -11.71227324440729411 ) ) ;
#86101=ADVANCED_FACE ( 'NONE', ( #144047 ), #50481, .F. ) ;
#86110=CARTESIAN_POINT ( 'NONE',  ( 10.99643026930483991, -5.229832900979420884, -0.2868663046952705242 ) ) ;
#86132=FILL_AREA_STYLE ('',( #37376 ) ) ;
#86264=CARTESIAN_POINT ( 'NONE',  ( -7.827294160508087906, -6.717993526550283256, 7.547439985188244549 ) ) ;
#86273=CIRCLE ( 'NONE', #210735, 0.07999999999999996003 ) ;
#86281=ORIENTED_EDGE ( 'NONE', *, *, #50401, .T. ) ;
#86288=ORIENTED_EDGE ( 'NONE', *, *, #110858, .T. ) ;
#86295=DIRECTION ( 'NONE',  ( 0.6123724356957872539, 0.7071067811865541231, -0.3535533905932732313 ) ) ;
#86324=ORIENTED_EDGE ( 'NONE', *, *, #126186, .F. ) ;
#86335=ORIENTED_EDGE ( 'NONE', *, *, #199147, .F. ) ;
#86366=B_SPLINE_CURVE_WITH_KNOTS ( 'NONE', 3,
 ( #154988, #122581, #138749, #105189, #153926, #23897, #190661, #171226, #90003, #206919 ),
 .UNSPECIFIED., .F., .F.,
 ( 4, 2, 2, 2, 4 ),
 ( 0.000000000000000000, 0.0002334048330869030008, 0.0004668096661738060016, 0.0007002144992607089481, 0.0009336193323476120031 ),
 .UNSPECIFIED. ) ;
#86399=CARTESIAN_POINT ( 'NONE',  ( -10.99962150373186631, -9.919999999999998153, 0.09125116240079726715 ) ) ;
#86473=CARTESIAN_POINT ( 'NONE',  ( -9.499262961676867789, -8.008893676012023732, 0.1288460037566295513 ) ) ;
#86477=VERTEX_POINT ( 'NONE', #99520 ) ;
#86506=CARTESIAN_POINT ( 'NONE',  ( -0.3525790917593719653, -6.713792789267393424, -9.484899655072640101 ) ) ;
#86509=ADVANCED_FACE ( 'NONE', ( #82186 ), #68043, .T. ) ;
#86515=CARTESIAN_POINT ( 'NONE',  ( -7.712474369503325988, -6.289226506789196591, 7.712474369503350857 ) ) ;
#86540=CARTESIAN_POINT ( 'NONE',  ( 8.915975476025575830, 3.467171072964057910, 8.027980377473637574 ) ) ;
#86552=CARTESIAN_POINT ( 'NONE',  ( 2.494940289813108780, 3.038492715500545227, -11.73777120880564873 ) ) ;
#86557=ADVANCED_FACE ( 'NONE', ( #147217 ), #100436, .F. ) ;
#86590=CARTESIAN_POINT ( 'NONE',  ( 9.499700864329909678, -7.154544010627095219, 0.07538891330675402680 ) ) ;
#86621=CARTESIAN_POINT ( 'NONE',  ( -10.40319425600960201, -5.787668213791931748, 0.4366904681730437443 ) ) ;
#86655=FILL_AREA_STYLE ('',( #116020 ) ) ;
#86676=CARTESIAN_POINT ( 'NONE',  ( 9.492899823913848678, -8.233137084989849086, -0.3774118403930767363 ) ) ;
#86684=VERTEX_POINT ( 'NONE', #132666 ) ;
#86686=CARTESIAN_POINT ( 'NONE',  ( 0.000000000000000000, 3.000000000000002665, 8.049999999999993605 ) ) ;
#86723=CARTESIAN_POINT ( 'NONE',  ( -1.387778780781445676E-14, -5.907420853759282053, -10.91970695577495398 ) ) ;
#86731=EDGE_LOOP ( 'NONE', ( #22509, #124055, #5511, #28084 ) ) ;
#86737=ORIENTED_EDGE ( 'NONE', *, *, #21894, .F. ) ;
#86742=EDGE_LOOP ( 'NONE', ( #139844, #191414, #125049, #27051 ) ) ;
#86755=CIRCLE ( 'NONE', #83172, 0.08000000000000020983 ) ;
#86757=DIRECTION ( 'NONE',  ( 0.000000000000000000, 0.000000000000000000, 1.000000000000000000 ) ) ;
#86767=CARTESIAN_POINT ( 'NONE',  ( -1.040834085586084257E-14, -8.763419982614969683, -10.56339547890105202 ) ) ;
#86771=EDGE_CURVE ( 'NONE', #144299, #83007, #17780, .T. ) ;
#86781=DIRECTION ( 'NONE',  ( 0.000000000000000000, 1.000000000000000000, 0.000000000000000000 ) ) ;
#86783=CARTESIAN_POINT ( 'NONE',  ( -2.421437874748401775, 3.696394713403113208, 11.55257195323929231 ) ) ;
#86819=ADVANCED_FACE ( 'NONE', ( #131618 ), #144778, .T. ) ;
#86848=CARTESIAN_POINT ( 'NONE',  ( 0.4350533241460359801, -6.938200158402027640, 9.251576347356904151 ) ) ;
#86865=CARTESIAN_POINT ( 'NONE',  ( 9.499671278040523248, -9.915617081696053603, -0.07902916658836418862 ) ) ;
#86879=ORIENTED_EDGE ( 'NONE', *, *, #195623, .F. ) ;
#86888=ORIENTED_EDGE ( 'NONE', *, *, #126196, .T. ) ;
#86918=CARTESIAN_POINT ( 'NONE',  ( -0.04698948850442342950, -9.984793193541563028, -9.579582872750561862 ) ) ;
#86925=CARTESIAN_POINT ( 'NONE',  ( 0.000000000000000000, 15.50000000000019362, 0.000000000000000000 ) ) ;
#86927=CARTESIAN_POINT ( 'NONE',  ( 7.654042494670958593E-16, 3.799999999999998046, -6.250000000000000000 ) ) ;
#86928=CARTESIAN_POINT ( 'NONE',  ( 9.481348452320371933, -9.006862915010128035, -0.5950054837411746789 ) ) ;
#86951=DIRECTION ( 'NONE',  ( 0.000000000000000000, 0.000000000000000000, -1.000000000000000000 ) ) ;
#87060=CARTESIAN_POINT ( 'NONE',  ( -1.040834085586084257E-14, -7.246166700194011767, -9.579665964935651701 ) ) ;
#87092=CYLINDRICAL_SURFACE ( 'NONE', #92084, 0.07999999999999993228 ) ;
#87099=DIRECTION ( 'NONE',  ( 0.000000000000000000, -1.000000000000000000, 0.000000000000000000 ) ) ;
#87107=CARTESIAN_POINT ( 'NONE',  ( -10.99620347397582876, -6.863457517656843088, 0.2978015046999314408 ) ) ;
#87109=ORIENTED_EDGE ( 'NONE', *, *, #77660, .T. ) ;
#87137=CARTESIAN_POINT ( 'NONE',  ( -6.634380621478864093, -6.684699875907221589, -6.783773251375836644 ) ) ;
#87175=EDGE_CURVE ( 'NONE', #114100, #151754, #76229, .T. ) ;
#87246=TOROIDAL_SURFACE ( 'NONE', #201466, 9.580000000000001847, 0.08000000000000000167 ) ;
#87254=CARTESIAN_POINT ( 'NONE',  ( 0.01167607004786809163, -5.765528217051462789, -11.00020965659732930 ) ) ;
#87262=CARTESIAN_POINT ( 'NONE',  ( 0.000000000000000000, -0.02379966007286238305, -6.277139874739035896 ) ) ;
#87287=ORIENTED_EDGE ( 'NONE', *, *, #86771, .F. ) ;
#87291=CARTESIAN_POINT ( 'NONE',  ( -9.994890815243229198, 3.870538056096196833, -5.945519334325427785 ) ) ;
#87300=CARTESIAN_POINT ( 'NONE',  ( 0.09999999999999592548, -9.900000000000005684, 6.938893903907228378E-15 ) ) ;
#87314=CIRCLE ( 'NONE', #208358, 11.54340198673881979 ) ;
#87322=CARTESIAN_POINT ( 'NONE',  ( -9.620326184871647257, -9.190313392136378212, 0.3418113563954127132 ) ) ;
#87334=CARTESIAN_POINT ( 'NONE',  ( 0.09999999999999592548, -9.919999999999998153, 9.579478065113978147 ) ) ;
#87364=CARTESIAN_POINT ( 'NONE',  ( -10.91838098853858519, -9.962496060591744751, 0.1694417511252961916 ) ) ;
#87368=CARTESIAN_POINT ( 'NONE',  ( -7.465774003072956688, -6.268611901546733201, 7.465774003072982445 ) ) ;
#87406=STYLED_ITEM ( 'NONE', ( #137967 ), #52970 ) ;
#87461=VERTEX_POINT ( 'NONE', #126610 ) ;
#87466=ADVANCED_FACE ( 'NONE', ( #124487 ), #43307, .F. ) ;
#87569=CARTESIAN_POINT ( 'NONE',  ( -0.4370932794886463468, -5.427673425445475708, -10.76345817711984054 ) ) ;
#87592=CARTESIAN_POINT ( 'NONE',  ( -6.735605996566196296E-15, -8.407420853759283830, 11.00029519899101338 ) ) ;
#87603=CIRCLE ( 'NONE', #205086, 0.08000000000000020983 ) ;
#87636=FILL_AREA_STYLE_COLOUR ( '', #111661 ) ;
#87659=CARTESIAN_POINT ( 'NONE',  ( -7.002681350352347067, -8.176227052203543622, 6.455298931196943535 ) ) ;
#87671=CARTESIAN_POINT ( 'NONE',  ( -10.95632728729436600, -7.911711732698783806, 0.3221646467111946022 ) ) ;
#87678=ORIENTED_EDGE ( 'NONE', *, *, #188204, .T. ) ;
#87694=CARTESIAN_POINT ( 'NONE',  ( -1.138412281109779656E-15, -7.256398209935981392, -9.569423160902221781 ) ) ;
#87697=STYLED_ITEM ( 'NONE', ( #24308 ), #66162 ) ;
#87702=CARTESIAN_POINT ( 'NONE',  ( 0.000000000000000000, -8.407420853759283830, 10.91970695577495931 ) ) ;
#87726=CARTESIAN_POINT ( 'NONE',  ( -0.3641668253325896498, -9.063144096568910513, 9.630238394150005377 ) ) ;
#87751=ORIENTED_EDGE ( 'NONE', *, *, #6325, .T. ) ;
#87754=DIRECTION ( 'NONE',  ( -0.000000000000000000, 1.000000000000000000, -0.000000000000000000 ) ) ;
#87784=CARTESIAN_POINT ( 'NONE',  ( 10.48884024596648601, 1.000000000000000888, -5.608780650328974104 ) ) ;
#87839=CARTESIAN_POINT ( 'NONE',  ( -7.720982897393580124, -5.907420853759296264, 7.834948825496934610 ) ) ;
#87853=EDGE_CURVE ( 'NONE', #50012, #89957, #192461, .T. ) ;
#87878=CARTESIAN_POINT ( 'NONE',  ( -8.669853050657241766, 2.974000657017267901, -7.806370750283158522 ) ) ;
#87880=CARTESIAN_POINT ( 'NONE',  ( -7.470306724222256278, -6.701288531902446444, -8.074422843256989779 ) ) ;
#87900=CARTESIAN_POINT ( 'NONE',  ( 10.38614328979755719, 3.507114751586604129, -5.996442624206805405 ) ) ;
#87906=ORIENTED_EDGE ( 'NONE', *, *, #62295, .T. ) ;
#87913=ORIENTED_EDGE ( 'NONE', *, *, #114510, .F. ) ;
#87931=CARTESIAN_POINT ( 'NONE',  ( -10.99956415888072492, -9.918872522958837479, 0.09791994008663019999 ) ) ;
#87947=CARTESIAN_POINT ( 'NONE',  ( -6.434831245971854408, -8.233137084989849086, -7.097136523687855636 ) ) ;
#87959=CARTESIAN_POINT ( 'NONE',  ( 10.99962150373185210, -9.919999999999998153, -0.09125116240077391083 ) ) ;
#87974=STYLED_ITEM ( 'NONE', ( #138455 ), #108668 ) ;
#87987=ORIENTED_EDGE ( 'NONE', *, *, #76253, .F. ) ;
#87992=ORIENTED_EDGE ( 'NONE', *, *, #170841, .F. ) ;
#88001=CARTESIAN_POINT ( 'NONE',  ( -0.3553982319964891778, -6.532648833121158738, -9.473247973006305500 ) ) ;
#88051=ORIENTED_EDGE ( 'NONE', *, *, #87175, .T. ) ;
#88053=CARTESIAN_POINT ( 'NONE',  ( -0.4644097342743094270, -8.233137084989863297, -9.488641820551086070 ) ) ;
#88077=FACE_OUTER_BOUND ( 'NONE', #62429, .T. ) ;
#88110=ORIENTED_EDGE ( 'NONE', *, *, #199274, .F. ) ;
#88135=CIRCLE ( 'NONE', #136536, 0.07999999999999993228 ) ;
#88179=CARTESIAN_POINT ( 'NONE',  ( -9.579665964948885559, -7.246166700194470067, -0.07999999999998980149 ) ) ;
#88211=CARTESIAN_POINT ( 'NONE',  ( 6.953912913643685911, -8.144978210217292514, -6.511381374296902003 ) ) ;
#88223=AXIS2_PLACEMENT_3D ( 'NONE', #74655, #90922, #43242 ) ;
#88291=ADVANCED_FACE ( 'NONE', ( #209117 ), #60754, .T. ) ;
#88307=CARTESIAN_POINT ( 'NONE',  ( 9.584291988782252858, -7.189630408304556575, -0.001123102408822191766 ) ) ;
#88311=CARTESIAN_POINT ( 'NONE',  ( 0.000000000000000000, -8.233137084989849086, 0.000000000000000000 ) ) ;
#88335=CARTESIAN_POINT ( 'NONE',  ( -0.1007326007326104361, -9.919999999999998153, -10.99953876047306167 ) ) ;
#88373=CARTESIAN_POINT ( 'NONE',  ( 10.95700306400770785, -7.901429653175738643, -0.3289054322349463377 ) ) ;
#88438=ORIENTED_EDGE ( 'NONE', *, *, #15624, .T. ) ;
#88441=CARTESIAN_POINT ( 'NONE',  ( -10.91910517057295671, -9.994362614652946064, 0.1236848126708565976 ) ) ;
#88472=CARTESIAN_POINT ( 'NONE',  ( 9.495541471879706208, -9.135662283479117463, -0.2985557471763389259 ) ) ;
#88487=CARTESIAN_POINT ( 'NONE',  ( 9.578206920975004479, -9.954640969533222972, -0.1671882237015355210 ) ) ;
#88526=CARTESIAN_POINT ( 'NONE',  ( -6.689586359223961054, -7.817744194000433744, 6.745922712994593340 ) ) ;
#88537=ORIENTED_EDGE ( 'NONE', *, *, #162856, .T. ) ;
#88547=STYLED_ITEM ( 'NONE', ( #63469 ), #194681 ) ;
#88658=CARTESIAN_POINT ( 'NONE',  ( 0.07538891330674687974, -7.154544010627095219, -9.499700864329895467 ) ) ;
#88667=CARTESIAN_POINT ( 'NONE',  ( -7.900729602272470231, -6.805008568744116637, 7.460470246983066822 ) ) ;
#88742=AXIS2_PLACEMENT_3D ( 'NONE', #84324, #1978, #22503 ) ;
#88772=CARTESIAN_POINT ( 'NONE',  ( -10.14529669463614070, -6.681160345275602985, 1.138412281109779656E-15 ) ) ;
#88779=CARTESIAN_POINT ( 'NONE',  ( 9.499606442108964544, 7.849261790823902629, -0.08647222121513191417 ) ) ;
#88839=ORIENTED_EDGE ( 'NONE', *, *, #45284, .F. ) ;
#88840=FACE_BOUND ( 'NONE', #76603, .T. ) ;
#88876=CARTESIAN_POINT ( 'NONE',  ( 7.784592198500480897, -5.601927612791806510, -7.772296586883602920 ) ) ;
#88878=CARTESIAN_POINT ( 'NONE',  ( 11.41010744128096555, 2.630042260599927850, -3.716153451272507180 ) ) ;
#88909=PLANE ( 'NONE',  #139118 ) ;
#88934=B_SPLINE_CURVE_WITH_KNOTS ( 'NONE', 3,
 ( #53533, #24211, #138000, #89258, #69758, #22062, #122907, #57805, #156385, #121821 ),
 .UNSPECIFIED., .F., .F.,
 ( 4, 2, 2, 2, 4 ),
 ( 0.000000000000000000, 0.0002299353307164155296, 0.0004598706614328310592, 0.0006898059921492465888, 0.0009197413228656621184 ),
 .UNSPECIFIED. ) ;
#88983=B_SPLINE_CURVE_WITH_KNOTS ( 'NONE', 3,
 ( #93059, #125620, #56274, #140759, #76769, #7495, #24820 ),
 .UNSPECIFIED., .F., .F.,
 ( 4, 3, 4 ),
 ( 0.0001788552925466765887, 0.0009000000022260272806, 0.002103779968145167399 ),
 .UNSPECIFIED. ) ;
#89000=CARTESIAN_POINT ( 'NONE',  ( 9.498256814137546300, -6.950186805636712428, 0.04218801535506153805 ) ) ;
#89001=ORIENTED_EDGE ( 'NONE', *, *, #201793, .F. ) ;
#89022=CARTESIAN_POINT ( 'NONE',  ( -9.584290747383006348, -7.189645481338096111, 0.001121896803080109622 ) ) ;
#89041=ORIENTED_EDGE ( 'NONE', *, *, #60148, .T. ) ;
#89068=CARTESIAN_POINT ( 'NONE',  ( -8.917737905728749581, 3.447199233515649386, -8.029567276306266876 ) ) ;
#89070=CARTESIAN_POINT ( 'NONE',  ( -0.05647967004079332970, -9.990726209582318162, -9.579565160031974003 ) ) ;
#89095=( BOUNDED_SURFACE ( )  B_SPLINE_SURFACE ( 3, 2, ( 
 ( #11139, #65995, #127131 ),
 ( #41549, #44752, #110859 ),
 ( #28477, #94568, #200277 ),
 ( #169925, #101732, #134269 ) ),
 .UNSPECIFIED., .F., .F., .F. ) 
 B_SPLINE_SURFACE_WITH_KNOTS ( ( 4, 4 ),
 ( 3, 3 ),
 ( 0.005330693667047302006, 0.008357081610771109614 ),
 ( 0.000000000000000000, 1.000000000000000000 ),
 .UNSPECIFIED. ) 
 GEOMETRIC_REPRESENTATION_ITEM ( )  RATIONAL_B_SPLINE_SURFACE ( (
 ( 1.000000000000000000, 0.7187737999613676987, 1.000000000000000000),
 ( 1.000000000000000000, 0.7186585579881007435, 1.000000000000000000),
 ( 1.000000000000000000, 0.7185467277397570296, 1.000000000000000000),
 ( 1.000000000000000000, 0.7184380228464053442, 1.000000000000000000) ) ) 
 REPRESENTATION_ITEM ( '' )  SURFACE ( )  );
#89111=DIRECTION ( 'NONE',  ( 0.000000000000000000, 0.000000000000000000, 1.000000000000000000 ) ) ;
#89130=CARTESIAN_POINT ( 'NONE',  ( -5.232130268375919232E-15, -8.644755361503010604, 10.68216772480111132 ) ) ;
#89131=DIRECTION ( 'NONE',  ( 0.000000000000000000, -1.000000000000000000, 0.000000000000000000 ) ) ;
#89163=CARTESIAN_POINT ( 'NONE',  ( -9.499700864329909678, -7.154544010627095219, -0.07538891330675229208 ) ) ;
#89198=DIRECTION ( 'NONE',  ( 0.4999999999999917843, 0.000000000000000000, -0.8660254037844433705 ) ) ;
#89199=VERTEX_POINT ( 'NONE', #154801 ) ;
#89214=EDGE_CURVE ( 'NONE', #93709, #1871, #171751, .T. ) ;
#89220=CARTESIAN_POINT ( 'NONE',  ( -0.08522875510949735889, -9.999176759342303100, -10.91956886450204145 ) ) ;
#89225=DIRECTION ( 'NONE',  ( 0.000000000000000000, -1.000000000000000000, 0.000000000000000000 ) ) ;
#89234=CARTESIAN_POINT ( 'NONE',  ( -11.00020965659414784, -5.765528217051525850, -0.01167607004747446206 ) ) ;
#89246=CARTESIAN_POINT ( 'NONE',  ( -6.773846765317340868, -7.246166700180801001, -6.773846765317303564 ) ) ;
#89254=EDGE_CURVE ( 'NONE', #179210, #155393, #210489, .T. ) ;
#89258=CARTESIAN_POINT ( 'NONE',  ( -0.04208621775141922761, -6.437359833193936787, -10.89523958697327011 ) ) ;
#89267=VERTEX_POINT ( 'NONE', #90883 ) ;
#89270=EDGE_CURVE ( 'NONE', #76877, #167216, #93018, .T. ) ;
#89285=CARTESIAN_POINT ( 'NONE',  ( 6.828399852920184365, -6.891066458783410731, -6.756361134959164794 ) ) ;
#89289=CARTESIAN_POINT ( 'NONE',  ( 7.462104991928525166, -5.200000000000006395, 8.081892667527540652 ) ) ;
#89299=B_SPLINE_CURVE_WITH_KNOTS ( 'NONE', 3,
 ( #110379, #140720, #127720, #177447, #206734, #94086, #12783 ),
 .UNSPECIFIED., .F., .F.,
 ( 4, 3, 4 ),
 ( 0.000000000000000000, 0.0008000000000004425012, 0.002977368225425632356 ),
 .UNSPECIFIED. ) ;
#89307=AXIS2_PLACEMENT_3D ( 'NONE', #171103, #42199, #37911 ) ;
#89359=CARTESIAN_POINT ( 'NONE',  ( -10.99180900346419243, -6.701306620466445985, 0.4265819271708525262 ) ) ;
#89452=CARTESIAN_POINT ( 'NONE',  ( 10.99440753328297582, -7.824706741106266072, -0.3572413387871992696 ) ) ;
#89493=CARTESIAN_POINT ( 'NONE',  ( -1.138412281109779656E-15, -7.287292266289732368, -9.765991025965622185 ) ) ;
#89505=PLANE ( 'NONE',  #209695 ) ;
#89522=EDGE_CURVE ( 'NONE', #182484, #183422, #89299, .T. ) ;
#89525=EDGE_CURVE ( 'NONE', #45420, #117856, #145703, .T. ) ;
#89560=EDGE_LOOP ( 'NONE', ( #135757, #8427, #204240, #129836 ) ) ;
#89561=AXIS2_PLACEMENT_3D ( 'NONE', #58588, #205894, #189647 ) ;
#89565=FILL_AREA_STYLE_COLOUR ( '', #136518 ) ;
#89566=B_SPLINE_CURVE_WITH_KNOTS ( 'NONE', 3,
 ( #75184, #141296, #58927, #155359, #204069, #125086, #92530, #6944, #191044, #208362, #126146, #43773, #159634, #105571, #171603, #209419 ),
 .UNSPECIFIED., .F., .F.,
 ( 4, 3, 3, 3, 3, 4 ),
 ( 0.000000000000000000, 6.716675436050588027E-06, 1.344324725954647930E-05, 2.018532118334301782E-05, 2.694176617305359190E-05, 3.135538808398834659E-05 ),
 .UNSPECIFIED. ) ;
#89582=ORIENTED_EDGE ( 'NONE', *, *, #31074, .F. ) ;
#89614=DIRECTION ( 'NONE',  ( 0.000000000000000000, 1.000000000000000000, 0.000000000000000000 ) ) ;
#89620=AXIS2_PLACEMENT_3D ( 'NONE', #154326, #186808, #20034 ) ;
#89717=CIRCLE ( 'NONE', #96197, 9.499999999999992895 ) ;
#89746=CARTESIAN_POINT ( 'NONE',  ( -9.617648866954043640, -9.063431457505050304, 0.6035590660245172545 ) ) ;
#89791=EDGE_CURVE ( 'NONE', #204013, #194558, #79928, .T. ) ;
#89817=CARTESIAN_POINT ( 'NONE',  ( -9.488725015150309972, -6.691474851359276776, 0.09393477316945002265 ) ) ;
#89829=CARTESIAN_POINT ( 'NONE',  ( -10.96314634606098259, -7.723163831703881321, 0.5532327639488945348 ) ) ;
#89853=CARTESIAN_POINT ( 'NONE',  ( 9.836090041150102437, -8.872041098393760095, -0.1716895903079586339 ) ) ;
#89867=LINE ( 'NONE', #42181, #181775 ) ;
#89914=DIRECTION ( 'NONE',  ( 0.000000000000000000, 1.000000000000000000, 0.000000000000000000 ) ) ;
#89950=ORIENTED_EDGE ( 'NONE', *, *, #98152, .T. ) ;
#89954=DIRECTION ( 'NONE',  ( -0.6762880771785568790, 0.000000000000000000, -0.7366372490351884572 ) ) ;
#89957=VERTEX_POINT ( 'NONE', #137245 ) ;
#89963=ORIENTED_EDGE ( 'NONE', *, *, #213856, .T. ) ;
#89977=CARTESIAN_POINT ( 'NONE',  ( -0.01083140255524777523, -7.162053774861989019, -9.500385102287573602 ) ) ;
#89984=CARTESIAN_POINT ( 'NONE',  ( -10.38614328979765489, 3.507114751586604129, -5.996442624206661520 ) ) ;
#90003=CARTESIAN_POINT ( 'NONE',  ( 9.573337995800486055, -7.550885189219932236, 1.710794795216873110E-15 ) ) ;
#90029=CARTESIAN_POINT ( 'NONE',  ( -8.876521693626852283, 3.555461883994700312, -7.992456032239074304 ) ) ;
#90115=ADVANCED_FACE ( 'NONE', ( #3990 ), #67915, .F. ) ;
#90140=EDGE_LOOP ( 'NONE', ( #101618, #107464, #205281, #30679 ) ) ;
#90168=VERTEX_POINT ( 'NONE', #2921 ) ;
#90200=SURFACE_SIDE_STYLE ('',( #24097 ) ) ;
#90202=ORIENTED_EDGE ( 'NONE', *, *, #102912, .F. ) ;
#90204=CARTESIAN_POINT ( 'NONE',  ( -0.09463244300326445479, -8.038540703696433809, -9.499633399276474321 ) ) ;
#90243=EDGE_LOOP ( 'NONE', ( #151294, #125272, #166971, #170213 ) ) ;
#90252=CARTESIAN_POINT ( 'NONE',  ( -7.960263458884766052, -6.452016312668098941, 7.960263458884793586 ) ) ;
#90258=( LENGTH_UNIT ( ) NAMED_UNIT ( * ) SI_UNIT ( .MILLI., .METRE. ) );
#90278=AXIS2_PLACEMENT_3D ( 'NONE', #15514, #134651, #65325 ) ;
#90304=DIRECTION ( 'NONE',  ( 1.535693738322999099E-12, 1.000000000000000000, -1.561558963378103181E-12 ) ) ;
#90306=CARTESIAN_POINT ( 'NONE',  ( 0.000000000000000000, -7.699999999999998401, 0.000000000000000000 ) ) ;
#90309=VERTEX_POINT ( 'NONE', #204321 ) ;
#90314=COLOUR_RGB ( '', 0.31764706, 0.68627451, 0.89019608) ;
#90320=CARTESIAN_POINT ( 'NONE',  ( 0.000000000000000000, -7.154544010627095219, 0.000000000000000000 ) ) ;
#90324=ORIENTED_EDGE ( 'NONE', *, *, #25109, .T. ) ;
#90346=CARTESIAN_POINT ( 'NONE',  ( 7.730132016633517011, -5.756136661604418947, 7.730132016633493919 ) ) ;
#90360=AXIS2_PLACEMENT_3D ( 'NONE', #67036, #165638, #100631 ) ;
#90421=CARTESIAN_POINT ( 'NONE',  ( -11.00057242252814760, -6.459673408256604965, 0.07917133907650250602 ) ) ;
#90432=ADVANCED_FACE ( 'NONE', ( #77554 ), #43154, .F. ) ;
#90439=CARTESIAN_POINT ( 'NONE',  ( -9.581972888692712687, -7.217909409572546231, -3.920744210608467172E-13 ) ) ;
#90478=AXIS2_PLACEMENT_3D ( 'NONE', #77545, #171851, #57039 ) ;
#90480=CARTESIAN_POINT ( 'NONE',  ( -9.586610838029429260, -7.161464053357574855, 0.003376046620574835178 ) ) ;
#90492=CARTESIAN_POINT ( 'NONE',  ( 0.000000000000000000, 0.2000000000000057288, 11.29999999999998828 ) ) ;
#90575=VERTEX_POINT ( 'NONE', #9357 ) ;
#90583=VERTEX_POINT ( 'NONE', #177201 ) ;
#90585=CIRCLE ( 'NONE', #135574, 0.2000000000000005107 ) ;
#90601=ORIENTED_EDGE ( 'NONE', *, *, #139862, .F. ) ;
#90615=B_SPLINE_CURVE_WITH_KNOTS ( 'NONE', 3,
 ( #195156, #82447, #132317, #165845, #30530, #34760, #17431, #83514 ),
 .UNSPECIFIED., .F., .F.,
 ( 4, 2, 2, 4 ),
 ( 0.000000000000000000, 0.0002567066673176301821, 0.0005134133346352603641, 0.001026826669270521596 ),
 .UNSPECIFIED. ) ;
#90624=CARTESIAN_POINT ( 'NONE',  ( 9.616417370072170456, -9.251786168353179463, -0.2979722244324772840 ) ) ;
#90627=ORIENTED_EDGE ( 'NONE', *, *, #126677, .F. ) ;
#90628=CARTESIAN_POINT ( 'NONE',  ( -9.555169238417182243, -7.776896528353606897, 0.04234008746932083761 ) ) ;
#90686=ADVANCED_FACE ( 'NONE', ( #123958 ), #116959, .F. ) ;
#90690=EDGE_LOOP ( 'NONE', ( #27433, #120934, #180584, #205922, #128045, #178145, #63161, #158337, #203829, #185589, #7893, #154186, #175580 ) ) ;
#90744=CIRCLE ( 'NONE', #211764, 9.579999999999992966 ) ;
#90763=CARTESIAN_POINT ( 'NONE',  ( -9.488641820551103834, -8.233137084989849086, 0.4644097342743111478 ) ) ;
#90773=AXIS2_PLACEMENT_3D ( 'NONE', #67209, #198287, #183121 ) ;
#90806=CARTESIAN_POINT ( 'NONE',  ( -9.620809655836554342, -9.180994456877138887, 0.3503521373105362158 ) ) ;
#90809=CARTESIAN_POINT ( 'NONE',  ( -0.03146710860974352708, -8.100320323339552431, 10.94525894661336274 ) ) ;
#90814=CARTESIAN_POINT ( 'NONE',  ( -0.06290936665214684476, -8.043994141378487228, 10.94971099608171627 ) ) ;
#90864=VERTEX_POINT ( 'NONE', #164629 ) ;
#90883=CARTESIAN_POINT ( 'NONE',  ( 11.40591166468351503, 3.507114751586604129, -3.706005353348470255 ) ) ;
#90922=DIRECTION ( 'NONE',  ( -0.000000000000000000, 1.000000000000000000, -0.000000000000000000 ) ) ;
#90931=CARTESIAN_POINT ( 'NONE',  ( -0.08058608058608696112, -6.134628647623513231, 10.99970480893081870 ) ) ;
#90946=CARTESIAN_POINT ( 'NONE',  ( -9.906083622534515243, -9.418601272609036457, 0.1729113328156593465 ) ) ;
#90979=TOROIDAL_SURFACE ( 'NONE', #63289, 6.330000000000000959, 0.08000000000000000167 ) ;
#90986=CARTESIAN_POINT ( 'NONE',  ( 0.000000000000000000, 0.000000000000000000, 0.000000000000000000 ) ) ;
#90996=EDGE_CURVE ( 'NONE', #117856, #43490, #68122, .T. ) ;
#91034=ORIENTED_EDGE ( 'NONE', *, *, #73451, .T. ) ;
#91045=COLOUR_RGB ( '', 0.09019608, 0.27058824, 0.51372549) ;
#91101=VERTEX_POINT ( 'NONE', #209352 ) ;
#91102=CARTESIAN_POINT ( 'NONE',  ( 7.752014238602739730E-16, 0.9200000000000041478, -6.329999999999995630 ) ) ;
#91144=CARTESIAN_POINT ( 'NONE',  ( -10.99665086521320490, -7.860092950639682385, 0.2746580110251921614 ) ) ;
#91149=EDGE_CURVE ( 'NONE', #123257, #89199, #42494, .T. ) ;
#91156=DIRECTION ( 'NONE',  ( 0.000000000000000000, -2.190088388420720976E-12, -1.000000000000000000 ) ) ;
#91157=CARTESIAN_POINT ( 'NONE',  ( -10.99944088594793179, -9.904389777384739801, 0.1109062511178791205 ) ) ;
#91172=DIRECTION ( 'NONE',  ( 0.000000000000000000, -1.000000000000000000, 0.000000000000000000 ) ) ;
#91198=CARTESIAN_POINT ( 'NONE',  ( -2.189868734255737248, 1.000000000000000888, 11.69137891449146771 ) ) ;
#91206=CARTESIAN_POINT ( 'NONE',  ( 7.465774003072942477, -6.268611901546733201, -7.465774003072967346 ) ) ;
#91268=SURFACE_STYLE_USAGE ( .BOTH. , #42521 ) ;
#91274=EDGE_CURVE ( 'NONE', #183707, #83007, #50138, .T. ) ;
#91306=EDGE_LOOP ( 'NONE', ( #168600, #842, #211931, #177980 ) ) ;
#91330=FACE_OUTER_BOUND ( 'NONE', #59944, .T. ) ;
#91386=CARTESIAN_POINT ( 'NONE',  ( 10.99943594186085782, -9.910930717204459839, -0.1113955156348795106 ) ) ;
#91388=ORIENTED_EDGE ( 'NONE', *, *, #173163, .F. ) ;
#91397=ORIENTED_EDGE ( 'NONE', *, *, #52034, .F. ) ;
#91422=ORIENTED_EDGE ( 'NONE', *, *, #67115, .T. ) ;
#91428=ORIENTED_EDGE ( 'NONE', *, *, #32207, .F. ) ;
#91430=CARTESIAN_POINT ( 'NONE',  ( 7.653681110113487840, -5.402328468025356933, 7.847520364415523808 ) ) ;
#91503=AXIS2_PLACEMENT_3D ( 'NONE', #56503, #22901, #43473 ) ;
#91519=DIRECTION ( 'NONE',  ( 0.000000000000000000, 1.000000000000000000, 0.000000000000000000 ) ) ;
#91529=ADVANCED_FACE ( 'NONE', ( #97233, #197894 ), #31160, .T. ) ;
#91541=CARTESIAN_POINT ( 'NONE',  ( 0.000000000000000000, 0.2000000000000057288, 0.000000000000000000 ) ) ;
#91549=VECTOR ( 'NONE', #33311, 1000.000000000000000 ) ;
#91557=EDGE_LOOP ( 'NONE', ( #121369, #52113, #8694, #39142 ) ) ;
#91559=CARTESIAN_POINT ( 'NONE',  ( -0.08058608058609216529, -9.900000000000005684, -10.99970480893080271 ) ) ;
#91564=STYLED_ITEM ( 'NONE', ( #60609 ), #86101 ) ;
#91641=CARTESIAN_POINT ( 'NONE',  ( 0.1178541238725807350, -5.389012432655391649, 10.99948089704805199 ) ) ;
#91649=SURFACE_STYLE_USAGE ( .BOTH. , #8224 ) ;
#91664=CARTESIAN_POINT ( 'NONE',  ( 0.000000000000000000, -6.532648833121171172, 0.000000000000000000 ) ) ;
#91667=CIRCLE ( 'NONE', #36256, 0.08000000000000020983 ) ;
#91692=CARTESIAN_POINT ( 'NONE',  ( 0.003376046620571365731, -7.161464053357560644, 9.586610838029431036 ) ) ;
#91705=CARTESIAN_POINT ( 'NONE',  ( -9.579665964948882007, -7.473374494045003757, 5.204170427930421283E-15 ) ) ;
#91706=CARTESIAN_POINT ( 'NONE',  ( 9.499766273075879397, -9.919999999999998153, -0.06663900456894614188 ) ) ;
#91845=CARTESIAN_POINT ( 'NONE',  ( 10.91808280586644919, -9.921948886890824326, -0.1881369732364152614 ) ) ;
#91864=CARTESIAN_POINT ( 'NONE',  ( 0.08058608058606961388, -5.907420853759267843, -10.99970480893079738 ) ) ;
#91865=LINE ( 'NONE', #157921, #833 ) ;
#91885=FACE_OUTER_BOUND ( 'NONE', #39699, .T. ) ;
#91924=DIRECTION ( 'NONE',  ( 8.659560562354987092E-17, 0.7071067811865432429, -0.7071067811865517916 ) ) ;
#91953=( GEOMETRIC_REPRESENTATION_CONTEXT ( 3 ) GLOBAL_UNCERTAINTY_ASSIGNED_CONTEXT ( ( #176767 ) ) GLOBAL_UNIT_ASSIGNED_CONTEXT ( ( #107834, #25435, #26505 ) ) REPRESENTATION_CONTEXT ( 'NONE', 'WORKASPACE' ) );
#91982=DIRECTION ( 'NONE',  ( 0.000000000000000000, 0.000000000000000000, -1.000000000000000000 ) ) ;
#91988=ORIENTED_EDGE ( 'NONE', *, *, #72060, .F. ) ;
#92055=DIRECTION ( 'NONE',  ( -0.7347175152297780176, 0.000000000000000000, 0.6783731810844091381 ) ) ;
#92073=PRODUCT ( 'air flow regulation', 'air flow regulation', '', ( #151174 ) ) ;
#92084=AXIS2_PLACEMENT_3D ( 'NONE', #4737, #70812, #115399 ) ;
#92101=ORIENTED_EDGE ( 'NONE', *, *, #199274, .T. ) ;
#92140=DIRECTION ( 'NONE',  ( 0.000000000000000000, 0.000000000000000000, 1.000000000000000000 ) ) ;
#92177=CARTESIAN_POINT ( 'NONE',  ( 7.317172109023883486, -6.705807696135622997, 7.317172109023855953 ) ) ;
#92190=CARTESIAN_POINT ( 'NONE',  ( 0.09999999999999592548, -9.999999999999994671, 9.579478065113978147 ) ) ;
#92246=ORIENTED_EDGE ( 'NONE', *, *, #37148, .T. ) ;
#92255=CARTESIAN_POINT ( 'NONE',  ( -1.016884229002468915E-14, -9.671843677217918156, -9.585733692702609332 ) ) ;
#92265=FACE_OUTER_BOUND ( 'NONE', #138024, .T. ) ;
#92288=CARTESIAN_POINT ( 'NONE',  ( -7.786489011996894583, -5.767087321558959978, -7.770158002575229261 ) ) ;
#92330=CARTESIAN_POINT ( 'NONE',  ( -11.41042268598796561, 3.467171072964049028, 3.707471073020331076 ) ) ;
#92346=PRESENTATION_STYLE_ASSIGNMENT (( #91268 ) ) ;
#92353=EDGE_LOOP ( 'NONE', ( #52904, #10530, #54621, #70997, #107533, #15126 ) ) ;
#92379=EDGE_CURVE ( 'NONE', #201806, #128654, #22530, .T. ) ;
#92451=DIRECTION ( 'NONE',  ( -0.008295560218254071499, -1.694007603815957969E-16, -0.9999655912483517151 ) ) ;
#92479=CARTESIAN_POINT ( 'NONE',  ( -10.43434622977936854, 1.529612873802629780, 5.577395135400619708 ) ) ;
#92515=DIRECTION ( 'NONE',  ( 0.000000000000000000, 0.000000000000000000, -1.000000000000000000 ) ) ;
#92523=CARTESIAN_POINT ( 'NONE',  ( 6.766604819867117371, -7.256397064628601790, -6.766604819867143128 ) ) ;
#92530=CARTESIAN_POINT ( 'NONE',  ( 0.08500055850266946544, -9.912493587006867557, 10.99967158169071446 ) ) ;
#92615=AXIS2_PLACEMENT_3D ( 'NONE', #61689, #193808, #100586 ) ;
#92629=ADVANCED_FACE ( 'NONE', ( #155013 ), #39717, .T. ) ;
#92642=ADVANCED_FACE ( 'NONE', ( #173415 ), #68772, .F. ) ;
#92661=FACE_OUTER_BOUND ( 'NONE', #67358, .T. ) ;
#92701=CARTESIAN_POINT ( 'NONE',  ( 0.4382560683119198774, -5.200000000000008171, 10.99126615174921007 ) ) ;
#92711=AXIS2_PLACEMENT_3D ( 'NONE', #137791, #201674, #55456 ) ;
#92726=CIRCLE ( 'NONE', #26963, 8.049999999999993605 ) ;
#92794=CARTESIAN_POINT ( 'NONE',  ( -6.796206128891405740, -7.030236945366977075, 6.776587425048123059 ) ) ;
#92825=( BOUNDED_SURFACE ( )  B_SPLINE_SURFACE ( 3, 2, ( 
 ( #81040, #128803, #193717 ),
 ( #194785, #176419, #13886 ),
 ( #32293, #64782, #28026 ),
 ( #162301, #97309, #211020 ),
 ( #46421, #143958, #62644 ),
 ( #213152, #127761, #94124 ),
 ( #212082, #142886, #160162 ),
 ( #98359, #130923, #164424 ) ),
 .UNSPECIFIED., .F., .F., .T. ) 
 B_SPLINE_SURFACE_WITH_KNOTS ( ( 4, 2, 2, 4 ),
 ( 3, 3 ),
 ( 0.000000000000000000, 0.0004924884914732687849, 0.0007387327372099031231, 0.0009849769829465375697 ),
 ( 0.000000000000000000, 1.000000000000000000 ),
 .UNSPECIFIED. ) 
 GEOMETRIC_REPRESENTATION_ITEM ( )  RATIONAL_B_SPLINE_SURFACE ( (
 ( 1.000000000000000000, 0.7045118851637608426, 1.000000000000000000),
 ( 1.000000000000000000, 0.7593505504064975709, 1.000000000000000000),
 ( 1.000000000000000000, 0.8104906253032382324, 1.000000000000000000),
 ( 1.000000000000000000, 0.8722646935501497945, 1.000000000000000000),
 ( 1.000000000000000000, 0.8905178607896807597, 1.000000000000000000),
 ( 1.000000000000000000, 0.9170530604351546655, 1.000000000000000000),
 ( 1.000000000000000000, 0.9248184710078904969, 1.000000000000000000),
 ( 1.000000000000000000, 0.9238795325112871826, 1.000000000000000000) ) ) 
 REPRESENTATION_ITEM ( '' )  SURFACE ( )  );
#92876=FILL_AREA_STYLE_COLOUR ( '', #32257 ) ;
#92881=STYLED_ITEM ( 'NONE', ( #203569 ), #203429 ) ;
#92907=CARTESIAN_POINT ( 'NONE',  ( 10.91864124492992616, -9.978085788838701120, -0.1530507449821316146 ) ) ;
#92919=CARTESIAN_POINT ( 'NONE',  ( -6.688963559358025890, -6.732807188596383163, -6.903494779225468392 ) ) ;
#92958=CIRCLE ( 'NONE', #131190, 11.54340198673881979 ) ;
#92976=CARTESIAN_POINT ( 'NONE',  ( -2.493954129951868826, 3.487142912321097299, 11.73313169142968881 ) ) ;
#92980=EDGE_CURVE ( 'NONE', #146105, #129260, #153565, .T. ) ;
#92992=DIRECTION ( 'NONE',  ( 0.000000000000000000, 1.000000000000000000, 0.000000000000000000 ) ) ;
#93013=VERTEX_POINT ( 'NONE', #61262 ) ;
#93016=CARTESIAN_POINT ( 'NONE',  ( 0.2514851628624798496, -9.242341987627179734, -9.497468999145715074 ) ) ;
#93018=LINE ( 'NONE', #58364, #46876 ) ;
#93029=FACE_OUTER_BOUND ( 'NONE', #113595, .T. ) ;
#93059=CARTESIAN_POINT ( 'NONE',  ( 6.484567079770447329, -6.583980363594976737, 7.100579091573052004 ) ) ;
#93064=DIRECTION ( 'NONE',  ( -0.9980366791917738567, 0.000000000000000000, 0.06263215618080149316 ) ) ;
#93075=ORIENTED_EDGE ( 'NONE', *, *, #4848, .T. ) ;
#93109=VERTEX_POINT ( 'NONE', #70558 ) ;
#93122=CARTESIAN_POINT ( 'NONE',  ( 0.000000000000000000, 0.7999999999999951594, 11.69999999999999041 ) ) ;
#93127=CARTESIAN_POINT ( 'NONE',  ( -0.2868663046952891760, -5.229832900979432431, -10.99643026930490919 ) ) ;
#93154=CARTESIAN_POINT ( 'NONE',  ( 0.3080734816350748084, -8.169755926620672071, 9.495223711095322372 ) ) ;
#93184=ORIENTED_EDGE ( 'NONE', *, *, #138625, .F. ) ;
#93206=CARTESIAN_POINT ( 'NONE',  ( -9.579665964948885559, -7.473374494045003757, -0.07999999999998980149 ) ) ;
#93218=CARTESIAN_POINT ( 'NONE',  ( -7.636191794455552184, -6.027819618361864862, -7.636191794455517545 ) ) ;
#93229=ORIENTED_EDGE ( 'NONE', *, *, #6621, .F. ) ;
#93237=CARTESIAN_POINT ( 'NONE',  ( 10.58872653680447584, -6.465328379374285284, 9.269928574751062911E-15 ) ) ;
#93239=CARTESIAN_POINT ( 'NONE',  ( -10.10516068267232548, -6.085430761754775375, 0.4362825330288350734 ) ) ;
#93271=CARTESIAN_POINT ( 'NONE',  ( 7.005920419302681168, -8.176248043968630697, -6.451695228974969609 ) ) ;
#93273=DIRECTION ( 'NONE',  ( 0.000000000000000000, 0.000000000000000000, 1.000000000000000000 ) ) ;
#93280=CARTESIAN_POINT ( 'NONE',  ( -10.91804383151480806, -8.407420853759271395, 0.1905751639681790843 ) ) ;
#93292=LINE ( 'NONE', #59689, #1461 ) ;
#93297=CARTESIAN_POINT ( 'NONE',  ( -9.499668754396999759, -7.215568602690300537, -0.07933194018451479590 ) ) ;
#93314=CARTESIAN_POINT ( 'NONE',  ( -7.680942717881084292, -5.294771359305316061, -7.874499448206164764 ) ) ;
#93349=EDGE_LOOP ( 'NONE', ( #1832, #30946, #161495, #196620 ) ) ;
#93422=ORIENTED_EDGE ( 'NONE', *, *, #63875, .F. ) ;
#93430=CARTESIAN_POINT ( 'NONE',  ( -10.99681319029664728, -5.196788179137224795, 0.2733121965684452426 ) ) ;
#93494=ORIENTED_EDGE ( 'NONE', *, *, #44939, .T. ) ;
#93501=EDGE_LOOP ( 'NONE', ( #25827, #171878, #120524, #3440 ) ) ;
#93518=CARTESIAN_POINT ( 'NONE',  ( -6.770610912236891821, -7.154544010627095219, -6.663994888585869525 ) ) ;
#93575=FACE_OUTER_BOUND ( 'NONE', #122409, .T. ) ;
#93674=EDGE_CURVE ( 'NONE', #15203, #109724, #105601, .T. ) ;
#93703=ADVANCED_FACE ( 'NONE', ( #208043 ), #179530, .T. ) ;
#93709=VERTEX_POINT ( 'NONE', #196083 ) ;
#93762=CARTESIAN_POINT ( 'NONE',  ( 10.30923643716940141, 0.9706168436483928463, -5.952040432139411585 ) ) ;
#93767=CARTESIAN_POINT ( 'NONE',  ( 0.3540227772641007520, -5.166863022244653436, 10.99462479582587271 ) ) ;
#93788=ORIENTED_EDGE ( 'NONE', *, *, #85411, .T. ) ;
#93812=ORIENTED_EDGE ( 'NONE', *, *, #153420, .T. ) ;
#93821=CARTESIAN_POINT ( 'NONE',  ( -0.2970643657731193432, -6.863149499369280093, -10.99622371251743225 ) ) ;
#93920=CARTESIAN_POINT ( 'NONE',  ( -0.07933194154488912297, -7.246166700194011767, 9.499668754385634628 ) ) ;
#93956=EDGE_CURVE ( 'NONE', #194558, #184212, #205341, .T. ) ;
#93999=EDGE_CURVE ( 'NONE', #206986, #178508, #52656, .T. ) ;
#94015=CARTESIAN_POINT ( 'NONE',  ( -9.498884310698281652, -9.746166700192997467, 0.1658036423878506416 ) ) ;
#94022=CARTESIAN_POINT ( 'NONE',  ( 9.579603127937247109, -9.900000000000005684, -0.08720040834114990702 ) ) ;
#94046=CARTESIAN_POINT ( 'NONE',  ( 0.000000000000000000, 3.000000000000002665, 0.000000000000000000 ) ) ;
#94047=CARTESIAN_POINT ( 'NONE',  ( 10.39230484541330313, 3.447199233515649386, 5.999999999999906741 ) ) ;
#94053=SURFACE_STYLE_FILL_AREA ( #44228 ) ;
#94083=DIRECTION ( 'NONE',  ( 0.000000000000000000, 0.000000000000000000, 1.000000000000000000 ) ) ;
#94086=CARTESIAN_POINT ( 'NONE',  ( -0.3867890553498209427, 3.235871879154603725, 11.62250415223148003 ) ) ;
#94124=CARTESIAN_POINT ( 'NONE',  ( 0.2972806740312853857, -7.751137252134813416, -10.97067717498809891 ) ) ;
#94139=CARTESIAN_POINT ( 'NONE',  ( 0.4356160240586420263, -9.063431457505059186, -9.626717610576610795 ) ) ;
#94153=DIRECTION ( 'NONE',  ( 0.000000000000000000, 0.000000000000000000, 1.000000000000000000 ) ) ;
#94196=ORIENTED_EDGE ( 'NONE', *, *, #124205, .F. ) ;
#94234=VERTEX_POINT ( 'NONE', #163312 ) ;
#94238=VERTEX_POINT ( 'NONE', #208839 ) ;
#94305=EDGE_LOOP ( 'NONE', ( #15681, #94196, #118591, #87987 ) ) ;
#94314=CARTESIAN_POINT ( 'NONE',  ( -11.41267819554183127, 3.499999999999989342, 3.708203932499423150 ) ) ;
#94334=CARTESIAN_POINT ( 'NONE',  ( -7.439168848973998216, -6.893137084989842123, -8.103009739377998955 ) ) ;
#94353=CARTESIAN_POINT ( 'NONE',  ( -10.39025099420812204, 3.467171072964039702, 5.998814208453899788 ) ) ;
#94354=DIRECTION ( 'NONE',  ( 0.000000000000000000, 0.000000000000000000, 1.000000000000000000 ) ) ;
#94400=ADVANCED_FACE ( 'NONE', ( #11205 ), #192082, .F. ) ;
#94404=ORIENTED_EDGE ( 'NONE', *, *, #4848, .F. ) ;
#94429=CIRCLE ( 'NONE', #198132, 9.500000000000001776 ) ;
#94442=VERTEX_POINT ( 'NONE', #109861 ) ;
#94443=FACE_OUTER_BOUND ( 'NONE', #115437, .T. ) ;
#94484=VERTEX_POINT ( 'NONE', #207278 ) ;
#94505=ORIENTED_EDGE ( 'NONE', *, *, #156087, .T. ) ;
#94532=CARTESIAN_POINT ( 'NONE',  ( 0.000000000000000000, -0.9200000000000041478, 11.00000000000000178 ) ) ;
#94561=ORIENTED_EDGE ( 'NONE', *, *, #152940, .F. ) ;
#94568=CARTESIAN_POINT ( 'NONE',  ( 10.20634067979362669, 1.972237431424148646, 5.892633538918198965 ) ) ;
#94587=CARTESIAN_POINT ( 'NONE',  ( -6.830415307812264025, 7.849261790823902629, -6.717278222822378630 ) ) ;
#94607=CARTESIAN_POINT ( 'NONE',  ( -10.46159335054558781, 1.264806443676224301, 5.593087811558907774 ) ) ;
#94617=CARTESIAN_POINT ( 'NONE',  ( 0.4330588727801780724, -9.006862915010128035, -9.570206894979136791 ) ) ;
#94689=AXIS2_PLACEMENT_3D ( 'NONE', #69701, #89198, #188810 ) ;
#94783=( LENGTH_UNIT ( ) NAMED_UNIT ( * ) SI_UNIT ( .MILLI., .METRE. ) );
#94831=EDGE_CURVE ( 'NONE', #17720, #178508, #67510, .T. ) ;
#94842=ORIENTED_EDGE ( 'NONE', *, *, #68964, .T. ) ;
#94862=EDGE_CURVE ( 'NONE', #105253, #181416, #185392, .T. ) ;
#94869=ORIENTED_EDGE ( 'NONE', *, *, #159427, .F. ) ;
#94871=CARTESIAN_POINT ( 'NONE',  ( -2.026920941591053626, 3.691791674785632082, 11.39597588158940411 ) ) ;
#94894=ORIENTED_EDGE ( 'NONE', *, *, #110555, .F. ) ;
#94908=AXIS2_PLACEMENT_3D ( 'NONE', #189690, #172393, #138833 ) ;
#94928=CARTESIAN_POINT ( 'NONE',  ( -7.842350841322885735, -5.412329794880682776, 7.657759090810040803 ) ) ;
#94946=ORIENTED_EDGE ( 'NONE', *, *, #116636, .F. ) ;
#94979=CARTESIAN_POINT ( 'NONE',  ( -9.578206935409053102, -9.746166700193986898, 0.1671882239534360770 ) ) ;
#94983=CARTESIAN_POINT ( 'NONE',  ( 7.580882385732059525, -6.105993949506566487, 7.580882385732033768 ) ) ;
#95017=CARTESIAN_POINT ( 'NONE',  ( 7.978162878861384755, -5.230039540835521805, -7.573156686838170337 ) ) ;
#95035=CARTESIAN_POINT ( 'NONE',  ( 7.253242555595320162, -7.896420114628004860, -6.595517585942703320 ) ) ;
#95047=CARTESIAN_POINT ( 'NONE',  ( 0.4382560683119269829, -7.666862915010147717, -10.99126615174920296 ) ) ;
#95057=EDGE_CURVE ( 'NONE', #17507, #193127, #126547, .T. ) ;
#95065=CIRCLE ( 'NONE', #109022, 0.08000000000000020983 ) ;
#95081=VECTOR ( 'NONE', #149504, 1000.000000000000000 ) ;
#95110=AXIS2_PLACEMENT_3D ( 'NONE', #172149, #155896, #7484 ) ;
#95138=CARTESIAN_POINT ( 'NONE',  ( 9.499262961676938843, -8.008893676011952678, -0.1288460037566319938 ) ) ;
#95154=EDGE_CURVE ( 'NONE', #197280, #40132, #89867, .T. ) ;
#95186=FACE_OUTER_BOUND ( 'NONE', #203216, .T. ) ;
#95197=CONICAL_SURFACE ( 'NONE', #57152, 11.49999999999998934, 0.7853981633974396193 ) ;
#95202=FACE_OUTER_BOUND ( 'NONE', #3427, .T. ) ;
#95216=CARTESIAN_POINT ( 'NONE',  ( 0.000000000000000000, 0.000000000000000000, 0.000000000000000000 ) ) ;
#95231=UNCERTAINTY_MEASURE_WITH_UNIT (LENGTH_MEASURE( 1.000000000000000082E-05 ), #120207, 'distance_accuracy_value', 'NONE');
#95245=ORIENTED_EDGE ( 'NONE', *, *, #148514, .F. ) ;
#95253=CARTESIAN_POINT ( 'NONE',  ( 6.773846765317333762, -7.246166700180801001, 6.773846765317311558 ) ) ;
#95262=DIRECTION ( 'NONE',  ( 0.000000000000000000, 0.000000000000000000, 1.000000000000000000 ) ) ;
#95288=ORIENTED_EDGE ( 'NONE', *, *, #123001, .F. ) ;
#95316=ORIENTED_EDGE ( 'NONE', *, *, #115695, .F. ) ;
#95370=AXIS2_PLACEMENT_3D ( 'NONE', #75946, #110650, #91156 ) ;
#95376=MECHANICAL_DESIGN_GEOMETRIC_PRESENTATION_REPRESENTATION('',(#88547),#123270);
#95387=EDGE_CURVE ( 'NONE', #192862, #82080, #101761, .T. ) ;
#95401=ORIENTED_EDGE ( 'NONE', *, *, #134348, .T. ) ;
#95406=CARTESIAN_POINT ( 'NONE',  ( -0.03870269234685246723, -9.454881121928412568, 9.603712783164930045 ) ) ;
#95409=FACE_BOUND ( 'NONE', #11984, .T. ) ;
#95412=CIRCLE ( 'NONE', #195732, 0.07999999999999993228 ) ;
#95425=DIRECTION ( 'NONE',  ( 0.000000000000000000, 0.000000000000000000, -1.000000000000000000 ) ) ;
#95429=FACE_OUTER_BOUND ( 'NONE', #139348, .T. ) ;
#95436=CIRCLE ( 'NONE', #130121, 0.07999999999999993228 ) ;
#95516=CARTESIAN_POINT ( 'NONE',  ( -9.578219923806457814, -9.914766490055704651, 0.1663656176996666236 ) ) ;
#95542=CARTESIAN_POINT ( 'NONE',  ( 0.000000000000000000, 0.9200000000000041478, 0.000000000000000000 ) ) ;
#95548=VERTEX_POINT ( 'NONE', #191451 ) ;
#95561=ORIENTED_EDGE ( 'NONE', *, *, #48296, .T. ) ;
#95607=CARTESIAN_POINT ( 'NONE',  ( 11.46094690312845898, 3.019799309332868553, -3.723887386306110159 ) ) ;
#95632=B_SPLINE_CURVE_WITH_KNOTS ( 'NONE', 3,
 ( #40238, #105250, #41319, #122643, #104174, #189669, #38102 ),
 .UNSPECIFIED., .F., .F.,
 ( 4, 3, 4 ),
 ( 1.399251010623063628E-17, 0.0008000000000005097218, 0.002977368225425562100 ),
 .UNSPECIFIED. ) ;
#95681=ORIENTED_EDGE ( 'NONE', *, *, #89791, .T. ) ;
#95694=EDGE_LOOP ( 'NONE', ( #66715, #22591, #149720, #199791 ) ) ;
#95737=AXIS2_PLACEMENT_3D ( 'NONE', #69340, #37941, #187379 ) ;
#95747=DIRECTION ( 'NONE',  ( 0.000000000000000000, 1.000000000000000000, 0.000000000000000000 ) ) ;
#95751=CARTESIAN_POINT ( 'NONE',  ( 7.461813752226484020, -6.074287852078599670, -6.844806938814754105 ) ) ;
#95773=DIRECTION ( 'NONE',  ( 0.000000000000000000, 0.000000000000000000, -1.000000000000000000 ) ) ;
#95796=CIRCLE ( 'NONE', #43843, 11.89429233241351902 ) ;
#95844=EDGE_LOOP ( 'NONE', ( #173067, #24232, #211941, #192750 ) ) ;
#95855=( NAMED_UNIT ( * ) PLANE_ANGLE_UNIT ( ) SI_UNIT ( $, .RADIAN. ) );
#95870=CONICAL_SURFACE ( 'NONE', #130554, 11.49999999999998934, 0.7853981633974396193 ) ;
#95902=CARTESIAN_POINT ( 'NONE',  ( 7.664830294503436114, -5.907420853759296264, -7.777967379493309075 ) ) ;
#95943=CIRCLE ( 'NONE', #158088, 9.499999999999992895 ) ;
#96032=CARTESIAN_POINT ( 'NONE',  ( -9.579698345292687378, -7.154544010627095219, -0.07602376731354575090 ) ) ;
#96073=EDGE_CURVE ( 'NONE', #82527, #99453, #163245, .T. ) ;
#96077=CARTESIAN_POINT ( 'NONE',  ( -1.219727444046192488E-15, -7.721243112841094103, 10.98746396341379317 ) ) ;
#96114=DIRECTION ( 'NONE',  ( 0.000000000000000000, -1.000000000000000000, 0.000000000000000000 ) ) ;
#96171=CIRCLE ( 'NONE', #68450, 11.54340198673881979 ) ;
#96195=VERTEX_POINT ( 'NONE', #11642 ) ;
#96197=AXIS2_PLACEMENT_3D ( 'NONE', #17324, #37863, #101797 ) ;
#96210=SURFACE_SIDE_STYLE ('',( #30121 ) ) ;
#96214=CARTESIAN_POINT ( 'NONE',  ( -0.05470795666946129399, -5.634700952767740745, 11.00000000000002487 ) ) ;
#96226=CARTESIAN_POINT ( 'NONE',  ( -1.734723475976807094E-15, -6.134628647623513231, -10.91970695577494332 ) ) ;
#96258=ADVANCED_FACE ( 'NONE', ( #178433 ), #164643, .T. ) ;
#96261=CARTESIAN_POINT ( 'NONE',  ( 10.36809559534897573, -7.321523296574929063, -0.4642244361878615222 ) ) ;
#96301=CARTESIAN_POINT ( 'NONE',  ( 0.4638907948587486785, -7.079050064870604508, 10.61081979358357863 ) ) ;
#96313=FILL_AREA_STYLE ('',( #81102 ) ) ;
#96317=CARTESIAN_POINT ( 'NONE',  ( 6.776323704810607751, -7.189630408300039299, 6.777912011469599207 ) ) ;
#96339=ADVANCED_FACE ( 'NONE', ( #179497 ), #143963, .T. ) ;
#96341=CARTESIAN_POINT ( 'NONE',  ( -1.355252715606880543E-15, 4.021557182957054444, 11.93179687198411720 ) ) ;
#96355=CARTESIAN_POINT ( 'NONE',  ( 0.1489494290324722969, -7.995840219786913394, 9.536979704252537715 ) ) ;
#96378=DIRECTION ( 'NONE',  ( 0.000000000000000000, 0.000000000000000000, 1.000000000000000000 ) ) ;
#96395=ADVANCED_FACE ( 'NONE', ( #169627 ), #134004, .T. ) ;
#96438=B_SPLINE_CURVE_WITH_KNOTS ( 'NONE', 3,
 ( #155523, #190141, #8191, #156599, #7104, #203172, #189083, #38569 ),
 .UNSPECIFIED., .F., .F.,
 ( 4, 2, 2, 4 ),
 ( 1.065747948313845892E-15, 0.0004636157603174433485, 0.0006954236404756316495, 0.0009272315206338199505 ),
 .UNSPECIFIED. ) ;
#96467=VERTEX_POINT ( 'NONE', #21210 ) ;
#96477=ORIENTED_EDGE ( 'NONE', *, *, #169747, .T. ) ;
#96523=CIRCLE ( 'NONE', #207182, 6.329999999999995630 ) ;
#96541=VERTEX_POINT ( 'NONE', #63384 ) ;
#96546=CARTESIAN_POINT ( 'NONE',  ( -7.462104991928526054, -5.166862915010159263, -8.081892667527538876 ) ) ;
#96550=CARTESIAN_POINT ( 'NONE',  ( -0.07406709734315156113, -9.431556885384965838, 9.500634193481339196 ) ) ;
#96571=VECTOR ( 'NONE', #112840, 1000.000000000000000 ) ;
#96577=CARTESIAN_POINT ( 'NONE',  ( 6.608557002163613525, -8.105676417795780964, 6.825099317097805596 ) ) ;
#96609=FACE_OUTER_BOUND ( 'NONE', #76209, .T. ) ;
#96623=VERTEX_POINT ( 'NONE', #184573 ) ;
#96632=CARTESIAN_POINT ( 'NONE',  ( -10.99934730582667797, -5.294005300192715424, 0.1376907581457726126 ) ) ;
#96645=( BOUNDED_SURFACE ( )  B_SPLINE_SURFACE ( 3, 2, ( 
 ( #100331, #198872, #32142 ),
 ( #98222, #117720, #116642 ),
 ( #151231, #182637, #84079 ),
 ( #34259, #166398, #17989 ) ),
 .UNSPECIFIED., .F., .F., .T. ) 
 B_SPLINE_SURFACE_WITH_KNOTS ( ( 4, 4 ),
 ( 3, 3 ),
 ( 0.000000000000000000, 9.170893477967426329E-05 ),
 ( 0.000000000000000000, 1.000000000000000000 ),
 .UNSPECIFIED. ) 
 GEOMETRIC_REPRESENTATION_ITEM ( )  RATIONAL_B_SPLINE_SURFACE ( (
 ( 1.000000000000000000, 0.6787756258918243857, 1.000000000000000000),
 ( 1.000000000000000000, 0.6894756946173453693, 1.000000000000000000),
 ( 1.000000000000000000, 0.6998898451713360114, 1.000000000000000000),
 ( 1.000000000000000000, 0.7100530722072171397, 1.000000000000000000) ) ) 
 REPRESENTATION_ITEM ( '' )  SURFACE ( )  );
#96665=CARTESIAN_POINT ( 'NONE',  ( 6.688963559358025002, -6.732807188596389381, 6.903494779225465727 ) ) ;
#96678=FILL_AREA_STYLE ('',( #32705 ) ) ;
#96686=CARTESIAN_POINT ( 'NONE',  ( 7.834948825496932834, -6.134628647623485698, 7.720982897393586342 ) ) ;
#96742=CARTESIAN_POINT ( 'NONE',  ( 7.968844136639799736, -5.196967604326696133, -7.583016927391841300 ) ) ;
#96762=ORIENTED_EDGE ( 'NONE', *, *, #118406, .F. ) ;
#96772=CARTESIAN_POINT ( 'NONE',  ( -9.497255425109827343, -6.896119493545144863, 0.09872732973945987089 ) ) ;
#96781=DIRECTION ( 'NONE',  ( 0.000000000000000000, 1.000000000000000000, 0.000000000000000000 ) ) ;
#96801=FACE_OUTER_BOUND ( 'NONE', #189045, .T. ) ;
#96812=LINE ( 'NONE', #134642, #50636 ) ;
#96819=DIRECTION ( 'NONE',  ( 0.000000000000000000, 1.000000000000000000, 0.000000000000000000 ) ) ;
#96853=CARTESIAN_POINT ( 'NONE',  ( 0.000000000000000000, -2.000000000000001776, 0.000000000000000000 ) ) ;
#96917=ORIENTED_EDGE ( 'NONE', *, *, #114330, .F. ) ;
#96941=AXIS2_PLACEMENT_3D ( 'NONE', #47854, #64076, #192990 ) ;
#96969=CARTESIAN_POINT ( 'NONE',  ( 0.000000000000000000, 15.50000000000019362, 0.000000000000000000 ) ) ;
#96981=DIRECTION ( 'NONE',  ( 0.000000000000000000, 0.000000000000000000, 1.000000000000000000 ) ) ;
#96997=CARTESIAN_POINT ( 'NONE',  ( 9.611344009005486910, -6.731960136058449784, -0.1523027874134945669 ) ) ;
#97016=CARTESIAN_POINT ( 'NONE',  ( 0.4637852190931108232, -7.024005807102823518, 10.66594404249596728 ) ) ;
#97062=CARTESIAN_POINT ( 'NONE',  ( -10.10343170205618968, 2.974000657016934390, -5.833219012919392377 ) ) ;
#97080=ADVANCED_FACE ( 'NONE', ( #207235 ), #208590, .T. ) ;
#97081=ORIENTED_EDGE ( 'NONE', *, *, #68964, .F. ) ;
#97096=ADVANCED_FACE ( 'NONE', ( #71880 ), #42639, .T. ) ;
#97172=EDGE_CURVE ( 'NONE', #105253, #72492, #188759, .T. ) ;
#97173=CARTESIAN_POINT ( 'NONE',  ( -9.488641820551102057, -8.233137084989836652, 0.4644097342743139234 ) ) ;
#97204=ADVANCED_FACE ( 'NONE', ( #6880 ), #120126, .T. ) ;
#97209=CARTESIAN_POINT ( 'NONE',  ( 7.777967379493318845, -9.999999999999994671, 7.744830294503448620 ) ) ;
#97233=FACE_BOUND ( 'NONE', #144787, .T. ) ;
#97266=CARTESIAN_POINT ( 'NONE',  ( 9.500232605408204023, -7.619382996155577459, 0.01181297548900739694 ) ) ;
#97288=EDGE_CURVE ( 'NONE', #76748, #135683, #95412, .T. ) ;
#97309=CARTESIAN_POINT ( 'NONE',  ( 0.1172869779874900348, -7.889939693150851419, -10.99948653685772726 ) ) ;
#97346=EDGE_CURVE ( 'NONE', #183546, #6442, #57339, .T. ) ;
#97410=CARTESIAN_POINT ( 'NONE',  ( -4.792515913634093623E-13, -7.868798029037626485, 9.500000000000001776 ) ) ;
#97413=CARTESIAN_POINT ( 'NONE',  ( -9.836090041150098884, -8.872041098393765424, 0.1716895903079178054 ) ) ;
#97511=( BOUNDED_SURFACE ( )  B_SPLINE_SURFACE ( 3, 2, ( 
 ( #136424, #152656, #6381 ),
 ( #202440, #4238, #135361 ),
 ( #56225, #3172, #19438 ),
 ( #54095, #37840, #118094 ),
 ( #39983, #103917, #151604 ),
 ( #155862, #201376, #72452 ),
 ( #137491, #85518, #169963 ),
 ( #36759, #153728, #5297 ) ),
 .UNSPECIFIED., .F., .F., .T. ) 
 B_SPLINE_SURFACE_WITH_KNOTS ( ( 4, 2, 2, 4 ),
 ( 3, 3 ),
 ( 0.000000000000000000, 0.0005109843281227174992, 0.0007664764921840762487, 0.001021968656245434998 ),
 ( 0.000000000000000000, 1.000000000000000000 ),
 .UNSPECIFIED. ) 
 GEOMETRIC_REPRESENTATION_ITEM ( )  RATIONAL_B_SPLINE_SURFACE ( (
 ( 1.000000000000000000, 0.7045118851637607316, 1.000000000000000000),
 ( 1.000000000000000000, 0.6478559580225851100, 1.000000000000000000),
 ( 1.000000000000000000, 0.5832506164441697560, 1.000000000000000000),
 ( 1.000000000000000000, 0.4879709628492566731, 1.000000000000000000),
 ( 1.000000000000000000, 0.4561823831825915221, 1.000000000000000000),
 ( 1.000000000000000000, 0.4039565156456190742, 1.000000000000000000),
 ( 1.000000000000000000, 0.3848936348729956602, 1.000000000000000000),
 ( 1.000000000000000000, 0.3826834323650904479, 1.000000000000000000) ) ) 
 REPRESENTATION_ITEM ( '' )  SURFACE ( )  );
#97526=CARTESIAN_POINT ( 'NONE',  ( 0.005636796283160772081, -9.933099634201859374, 9.579656484007951889 ) ) ;
#97527=CARTESIAN_POINT ( 'NONE',  ( 6.764644832403535979, -7.632775601084324180, -6.764644832400978025 ) ) ;
#97579=CARTESIAN_POINT ( 'NONE',  ( 10.99740610014205267, -6.654245765634905219, -0.2680151545361366128 ) ) ;
#97594=PRESENTATION_STYLE_ASSIGNMENT (( #80255 ) ) ;
#97602=ADVANCED_FACE ( 'NONE', ( #146548 ), #46905, .T. ) ;
#97633=CARTESIAN_POINT ( 'NONE',  ( 6.381095703207959602, -8.200000000000001066, 7.037870247915979149 ) ) ;
#97670=ORIENTED_EDGE ( 'NONE', *, *, #8812, .F. ) ;
#97726=LINE ( 'NONE', #75318, #83896 ) ;
#97728=CARTESIAN_POINT ( 'NONE',  ( -0.1000000000000028644, -9.999999999999994671, 0.000000000000000000 ) ) ;
#97765=LINE ( 'NONE', #132415, #66630 ) ;
#97791=COLOUR_RGB ( '', 0.66274510, 0.83137255, 0.94901961) ;
#97793=CARTESIAN_POINT ( 'NONE',  ( 6.773846765317306229, -7.246166700180828535, -6.773846765317331986 ) ) ;
#97798=VERTEX_POINT ( 'NONE', #102028 ) ;
#97830=CARTESIAN_POINT ( 'NONE',  ( 0.08044988649997392161, -9.906619926850268598, 9.499659352616927066 ) ) ;
#97846=CIRCLE ( 'NONE', #11382, 9.523431457505067144 ) ;
#97857=CARTESIAN_POINT ( 'NONE',  ( -9.500102690074733403, -7.891095720666440272, 0.004933703209202861852 ) ) ;
#97863=CIRCLE ( 'NONE', #122208, 11.99999999999999112 ) ;
#97868=CARTESIAN_POINT ( 'NONE',  ( -7.724608556409207516, -5.759585062615365736, -7.735357998705601368 ) ) ;
#97878=FACE_OUTER_BOUND ( 'NONE', #196698, .T. ) ;
#97893=CARTESIAN_POINT ( 'NONE',  ( 10.41509302999109110, 1.813436143228260855, -5.960384690635902594 ) ) ;
#97912=SURFACE_STYLE_FILL_AREA ( #149854 ) ;
#97941=AXIS2_PLACEMENT_3D ( 'NONE', #138624, #204648, #188418 ) ;
#98006=AXIS2_PLACEMENT_3D ( 'NONE', #69693, #155244, #23077 ) ;
#98059=FACE_OUTER_BOUND ( 'NONE', #157898, .T. ) ;
#98069=ORIENTED_EDGE ( 'NONE', *, *, #25801, .T. ) ;
#98091=COLOUR_RGB ( '', 0.08235294, 0.09019608, 0.10196078) ;
#98096=DIRECTION ( 'NONE',  ( 0.04267330865764863701, 0.000000000000000000, 0.9990890794760038940 ) ) ;
#98127=CARTESIAN_POINT ( 'NONE',  ( 10.99970480893081692, -5.907420853759282053, 0.08058608058608254798 ) ) ;
#98138=B_SPLINE_CURVE_WITH_KNOTS ( 'NONE', 3,
 ( #196425, #162868, #195361, #95751, #213701, #127248, #128321 ),
 .UNSPECIFIED., .F., .F.,
 ( 4, 3, 4 ),
 ( 0.0001788552925466893823, 0.0009000000022260270637, 0.002103779968145176940 ),
 .UNSPECIFIED. ) ;
#98152=EDGE_CURVE ( 'NONE', #45056, #31312, #144125, .T. ) ;
#98207=CARTESIAN_POINT ( 'NONE',  ( 10.36939107341407507, 1.813436143228259745, 6.039542801432597585 ) ) ;
#98210=LINE ( 'NONE', #644, #177723 ) ;
#98222=CARTESIAN_POINT ( 'NONE',  ( 9.584290747383175102, -7.189645481338100552, -0.001121896803057515716 ) ) ;
#98224=VERTEX_POINT ( 'NONE', #185395 ) ;
#98226=CARTESIAN_POINT ( 'NONE',  ( 7.884707905546932238, -7.003075417673650271, -7.228805602686596110 ) ) ;
#98234=DIRECTION ( 'NONE',  ( 0.000000000000000000, 1.000000000000000000, 0.000000000000000000 ) ) ;
#98236=CARTESIAN_POINT ( 'NONE',  ( -0.4655551865852154414, -8.176568542494919711, -9.512045263456256450 ) ) ;
#98271=CARTESIAN_POINT ( 'NONE',  ( 7.654042494670951690E-16, -13.99999999999999822, -6.249999999999995559 ) ) ;
#98278=ORIENTED_EDGE ( 'NONE', *, *, #158238, .T. ) ;
#98281=ORIENTED_EDGE ( 'NONE', *, *, #53503, .F. ) ;
#98312=ORIENTED_EDGE ( 'NONE', *, *, #169996, .T. ) ;
#98333=CARTESIAN_POINT ( 'NONE',  ( 6.717748655459634399, -7.246166700180800113, 6.717748655459616636 ) ) ;
#98359=CARTESIAN_POINT ( 'NONE',  ( 0.4382560683119228195, -7.666862915010161039, -10.99126615174918520 ) ) ;
#98366=CARTESIAN_POINT ( 'NONE',  ( 9.578245405452067374, -9.921948021430829101, -0.1647502191513116609 ) ) ;
#98413=DIRECTION ( 'NONE',  ( 0.000000000000000000, 0.000000000000000000, 1.000000000000000000 ) ) ;
#98431=DIRECTION ( 'NONE',  ( 0.000000000000000000, 1.000000000000000000, 0.000000000000000000 ) ) ;
#98487=COLOUR_RGB ( '', 0.66274510, 0.83137255, 0.94901961) ;
#98534=ORIENTED_EDGE ( 'NONE', *, *, #77512, .T. ) ;
#98575=CARTESIAN_POINT ( 'NONE',  ( -0.06258739273032881689, -9.383611379567486921, 9.609645335164882951 ) ) ;
#98614=ORIENTED_EDGE ( 'NONE', *, *, #128928, .F. ) ;
#98621=DIRECTION ( 'NONE',  ( 0.000000000000000000, 1.000000000000000000, 0.000000000000000000 ) ) ;
#98628=CARTESIAN_POINT ( 'NONE',  ( 10.99387514841223279, -6.699757570937918238, -0.3793797362573342880 ) ) ;
#98644=FACE_OUTER_BOUND ( 'NONE', #86731, .T. ) ;
#98657=CARTESIAN_POINT ( 'NONE',  ( -0.1981138333789616013, -9.280569609800540576, 9.498748750704498534 ) ) ;
#98682=CARTESIAN_POINT ( 'NONE',  ( 6.745710774231037377, -7.818797203689475950, 6.689804758640298665 ) ) ;
#98691=EDGE_CURVE ( 'NONE', #90168, #176780, #158543, .T. ) ;
#98698=ORIENTED_EDGE ( 'NONE', *, *, #188812, .F. ) ;
#98719=DIRECTION ( 'NONE',  ( -0.7384114592165696989, -9.626321597927967204E-15, 0.6743504407188123384 ) ) ;
#98775=( BOUNDED_SURFACE ( )  B_SPLINE_SURFACE ( 3, 2, ( 
 ( #208054, #126909, #75937 ),
 ( #29325, #191798, #124776 ),
 ( #76991, #144191, #125841 ),
 ( #43461, #41330, #142038 ),
 ( #91144, #59681, #145246 ),
 ( #158272, #11990, #211252 ),
 ( #175586, #140982, #107439 ),
 ( #8797, #173463, #93280 ) ),
 .UNSPECIFIED., .F., .F., .T. ) 
 B_SPLINE_SURFACE_WITH_KNOTS ( ( 4, 2, 2, 4 ),
 ( 3, 3 ),
 ( 2.710505431213761085E-20, 0.0002475938981900018118, 0.0004951877963800036236, 0.0009903755927600072471 ),
 ( 0.000000000000000000, 1.000000000000000000 ),
 .UNSPECIFIED. ) 
 GEOMETRIC_REPRESENTATION_ITEM ( )  RATIONAL_B_SPLINE_SURFACE ( (
 ( 1.000000000000000000, 0.9238795325112864054, 1.000000000000000000),
 ( 1.000000000000000000, 0.9248499699752872338, 1.000000000000000000),
 ( 1.000000000000000000, 0.9171047238584292272, 1.000000000000000000),
 ( 1.000000000000000000, 0.8907236462368525176, 1.000000000000000000),
 ( 1.000000000000000000, 0.8725411758597159118, 1.000000000000000000),
 ( 1.000000000000000000, 0.8105159241137848136, 1.000000000000000000),
 ( 1.000000000000000000, 0.7599483315144378581, 1.000000000000000000),
 ( 1.000000000000000000, 0.7045118851637622859, 1.000000000000000000) ) ) 
 REPRESENTATION_ITEM ( '' )  SURFACE ( )  );
#98780=CARTESIAN_POINT ( 'NONE',  ( 10.76345817711984409, -5.427673425445473043, -0.4370932794886462913 ) ) ;
#98787=SURFACE_SIDE_STYLE ('',( #80394 ) ) ;
#98803=CARTESIAN_POINT ( 'NONE',  ( 10.30245174296181254, 3.603753425775774843, 5.948123287112013102 ) ) ;
#98820=ORIENTED_EDGE ( 'NONE', *, *, #110343, .F. ) ;
#98846=ORIENTED_EDGE ( 'NONE', *, *, #133466, .F. ) ;
#98858=CARTESIAN_POINT ( 'NONE',  ( -6.588752024304622701, -8.074889850123406987, -6.844216539294235346 ) ) ;
#98878=B_SPLINE_CURVE_WITH_KNOTS ( 'NONE', 3,
 ( #204853, #40262, #170243, #71656 ),
 .UNSPECIFIED., .F., .F.,
 ( 4, 4 ),
 ( 0.000000000000000000, 9.170750102251441879E-05 ),
 .UNSPECIFIED. ) ;
#98913=CARTESIAN_POINT ( 'NONE',  ( -9.499065438569621378, -8.103879979615419060, 0.1510907968719145678 ) ) ;
#98916=ORIENTED_EDGE ( 'NONE', *, *, #52034, .T. ) ;
#98990=FACE_OUTER_BOUND ( 'NONE', #17061, .T. ) ;
#99005=CARTESIAN_POINT ( 'NONE',  ( -7.664830294503444996, -5.907420853759296264, 7.777967379493320621 ) ) ;
#99016=CARTESIAN_POINT ( 'NONE',  ( 0.000000000000000000, -9.331509131462439655, 0.000000000000000000 ) ) ;
#99062=AXIS2_PLACEMENT_3D ( 'NONE', #62398, #144766, #128562 ) ;
#99077=CARTESIAN_POINT ( 'NONE',  ( -10.99643026930483813, -5.229832900979425325, 0.2868663046952791285 ) ) ;
#99112=DIRECTION ( 'NONE',  ( 0.8660254037844399289, 0.000000000000000000, 0.4999999999999978906 ) ) ;
#99123=FACE_OUTER_BOUND ( 'NONE', #99191, .T. ) ;
#99136=ORIENTED_EDGE ( 'NONE', *, *, #169996, .F. ) ;
#99139=CARTESIAN_POINT ( 'NONE',  ( -0.1025498324992805826, -6.714092063936416999, -10.99981089498244202 ) ) ;
#99172=FILL_AREA_STYLE ('',( #212901 ) ) ;
#99191=EDGE_LOOP ( 'NONE', ( #179598, #208662, #35957, #180985, #87992 ) ) ;
#99199=CARTESIAN_POINT ( 'NONE',  ( 0.2435857797690321180, -7.709701271428945901, -10.99755231369147168 ) ) ;
#99205=ORIENTED_EDGE ( 'NONE', *, *, #25220, .T. ) ;
#99211=CARTESIAN_POINT ( 'NONE',  ( -6.389500218612176319, -8.186910008818838236, -7.047919418996370311 ) ) ;
#99299=CARTESIAN_POINT ( 'NONE',  ( -0.04234008746932169803, -7.776896528353619331, -9.555169238417182243 ) ) ;
#99318=EDGE_CURVE ( 'NONE', #27864, #155393, #147642, .T. ) ;
#99327=CARTESIAN_POINT ( 'NONE',  ( -7.834474503270852708, -6.459788825448645078, 7.722692672890439702 ) ) ;
#99329=EDGE_CURVE ( 'NONE', #121012, #29173, #127002, .T. ) ;
#99375=ORIENTED_EDGE ( 'NONE', *, *, #51127, .T. ) ;
#99391=EDGE_LOOP ( 'NONE', ( #159936, #52396, #48407, #66299 ) ) ;
#99435=DIRECTION ( 'NONE',  ( 0.000000000000000000, -1.000000000000000000, 0.000000000000000000 ) ) ;
#99436=FILL_AREA_STYLE_COLOUR ( '', #27385 ) ;
#99453=VERTEX_POINT ( 'NONE', #137483 ) ;
#99500=CARTESIAN_POINT ( 'NONE',  ( -6.776370306708066948, -7.161464053357560644, -6.781144757626046626 ) ) ;
#99520=CARTESIAN_POINT ( 'NONE',  ( 9.579764304849151202, -9.999999999999994671, -0.06720017513373727214 ) ) ;
#99580=DIRECTION ( 'NONE',  ( -0.06086575749407437119, 0.9962285034897238045, 0.06183953750876716726 ) ) ;
#99602=FILL_AREA_STYLE ('',( #68136 ) ) ;
#99603=ADVANCED_FACE ( 'NONE', ( #104984 ), #82720, .T. ) ;
#99636=LINE ( 'NONE', #82307, #51164 ) ;
#99711=ORIENTED_EDGE ( 'NONE', *, *, #117706, .T. ) ;
#99738=DIRECTION ( 'NONE',  ( -0.000000000000000000, 1.000000000000000000, -0.000000000000000000 ) ) ;
#99742=DIRECTION ( 'NONE',  ( 0.000000000000000000, 0.000000000000000000, 1.000000000000000000 ) ) ;
#99744=STYLED_ITEM ( 'NONE', ( #82512 ), #33195 ) ;
#99750=CARTESIAN_POINT ( 'NONE',  ( 10.40319425600960201, -5.787668213791926419, -0.4366904681731619831 ) ) ;
#99761=B_SPLINE_CURVE_WITH_KNOTS ( 'NONE', 3,
 ( #135093, #122114, #1838, #88472, #72181, #188079, #6111, #52747 ),
 .UNSPECIFIED., .F., .F.,
 ( 4, 2, 2, 4 ),
 ( 2.602085213965179827E-18, 0.0002461874215021541226, 0.0004923748430043056431, 0.0009847496860086130208 ),
 .UNSPECIFIED. ) ;
#99793=ORIENTED_EDGE ( 'NONE', *, *, #65255, .F. ) ;
#99837=CARTESIAN_POINT ( 'NONE',  ( 10.55905904256946215, -5.631911363926713321, -0.4368516432692077789 ) ) ;
#99853=CARTESIAN_POINT ( 'NONE',  ( 7.458876248284573407, -7.605490376493627025, -6.801849632070416263 ) ) ;
#99870=ORIENTED_EDGE ( 'NONE', *, *, #138683, .T. ) ;
#99881=CARTESIAN_POINT ( 'NONE',  ( -7.142181811248260459E-15, -5.907420853759270507, 10.91970695577495221 ) ) ;
#99912=CARTESIAN_POINT ( 'NONE',  ( 8.024744567526232331, -5.166862915010145052, -7.523999700038788596 ) ) ;
#99918=CARTESIAN_POINT ( 'NONE',  ( -6.496114076516063207, -8.169775483750591150, -6.932145363377419045 ) ) ;
#99938=CARTESIAN_POINT ( 'NONE',  ( 0.000000000000000000, -9.999999999999994671, 0.000000000000000000 ) ) ;
#99943=CARTESIAN_POINT ( 'NONE',  ( 0.09770433987276584686, -9.919999999999998153, 9.499497670693809681 ) ) ;
#99945=CARTESIAN_POINT ( 'NONE',  ( 10.99958311221863028, -9.919613946868095056, -0.09579086958120625050 ) ) ;
#99959=VECTOR ( 'NONE', #208388, 1000.000000000000000 ) ;
#100024=CARTESIAN_POINT ( 'NONE',  ( -0.07538891330675576152, -7.154544010627095219, 9.499700864329900796 ) ) ;
#100026=CARTESIAN_POINT ( 'NONE',  ( 0.000000000000000000, -2.079999999999998295, 0.000000000000000000 ) ) ;
#100027=LINE ( 'NONE', #39292, #13848 ) ;
#100046=CARTESIAN_POINT ( 'NONE',  ( 0.000000000000000000, -7.699999999999998401, 0.000000000000000000 ) ) ;
#100067=CARTESIAN_POINT ( 'NONE',  ( -6.549078289569726152, -6.948428148671506932, -6.549078289569697731 ) ) ;
#100129=CARTESIAN_POINT ( 'NONE',  ( -10.94526678918444951, -5.600264386820970941, 0.03132844593997358151 ) ) ;
#100153=ORIENTED_EDGE ( 'NONE', *, *, #203402, .T. ) ;
#100172=ORIENTED_EDGE ( 'NONE', *, *, #189732, .T. ) ;
#100173=CARTESIAN_POINT ( 'NONE',  ( 9.606148981167445200, -6.583980363594983842, -0.4355862708379997228 ) ) ;
#100189=CARTESIAN_POINT ( 'NONE',  ( -0.4363033266127427923, -8.563898737988809629, 10.12670668089736736 ) ) ;
#100224=CARTESIAN_POINT ( 'NONE',  ( 10.99948089704798271, -5.389012432655394313, -0.1178541238725870494 ) ) ;
#100250=ORIENTED_EDGE ( 'NONE', *, *, #42999, .T. ) ;
#100257=EDGE_CURVE ( 'NONE', #71638, #189856, #12770, .T. ) ;
#100318=EDGE_LOOP ( 'NONE', ( #40127, #57102, #21906, #109189 ) ) ;
#100331=CARTESIAN_POINT ( 'NONE',  ( 9.586610838029429260, -7.161464053357567749, -0.003376046620571108124 ) ) ;
#100335=UNCERTAINTY_MEASURE_WITH_UNIT (LENGTH_MEASURE( 1.000000000000000082E-05 ), #107185, 'distance_accuracy_value', 'NONE');
#100367=CARTESIAN_POINT ( 'NONE',  ( -10.15369940311292929, 1.000000000000000888, -6.195664267729944719 ) ) ;
#100370=CARTESIAN_POINT ( 'NONE',  ( -0.07933194154488934502, -7.609852571077998284, 9.499668754385634628 ) ) ;
#100379=CARTESIAN_POINT ( 'NONE',  ( -8.042162931142703641, -6.699677480914128402, 7.505515594164491766 ) ) ;
#100389=ADVANCED_FACE ( 'NONE', ( #171844 ), #102637, .T. ) ;
#100399=ADVANCED_FACE ( 'NONE', ( #153463 ), #136154, .T. ) ;
#100436=( BOUNDED_SURFACE ( )  B_SPLINE_SURFACE ( 3, 2, ( 
 ( #58233, #153607, #70184 ),
 ( #53968, #72325, #5178 ),
 ( #56103, #173066, #122260 ),
 ( #170909, #22504, #24647 ) ),
 .UNSPECIFIED., .F., .F., .F. ) 
 B_SPLINE_SURFACE_WITH_KNOTS ( ( 4, 4 ),
 ( 3, 3 ),
 ( 0.005025772024296196530, 0.008052159968022380709 ),
 ( 0.000000000000000000, 1.000000000000000000 ),
 .UNSPECIFIED. ) 
 GEOMETRIC_REPRESENTATION_ITEM ( )  RATIONAL_B_SPLINE_SURFACE ( (
 ( 1.000000000000000000, 0.7187737999613663664, 1.000000000000000000),
 ( 1.000000000000000000, 0.7186585579881031860, 1.000000000000000000),
 ( 1.000000000000000000, 0.7185467277397551422, 1.000000000000000000),
 ( 1.000000000000000000, 0.7184380228464064544, 1.000000000000000000) ) ) 
 REPRESENTATION_ITEM ( '' )  SURFACE ( )  );
#100462=EDGE_CURVE ( 'NONE', #41837, #170487, #213314, .T. ) ;
#100501=CIRCLE ( 'NONE', #211202, 0.08000000000000020983 ) ;
#100553=UNCERTAINTY_MEASURE_WITH_UNIT (LENGTH_MEASURE( 1.000000000000000082E-05 ), #108866, 'distance_accuracy_value', 'NONE');
#100558=CARTESIAN_POINT ( 'NONE',  ( -10.39230484541323740, 3.447199233515621408, 6.000000000000048850 ) ) ;
#100586=DIRECTION ( 'NONE',  ( 0.000000000000000000, 0.000000000000000000, 1.000000000000000000 ) ) ;
#100589=VERTEX_POINT ( 'NONE', #71111 ) ;
#100607=CARTESIAN_POINT ( 'NONE',  ( -1.734723475976807094E-15, -6.134628647623513231, -10.91970695577494332 ) ) ;
#100616=B_SPLINE_CURVE_WITH_KNOTS ( 'NONE', 3,
 ( #67365, #148662, #46911, #97793 ),
 .UNSPECIFIED., .F., .F.,
 ( 4, 4 ),
 ( 0.000000000000000000, 8.505390838612159954E-05 ),
 .UNSPECIFIED. ) ;
#100631=DIRECTION ( 'NONE',  ( 0.000000000000000000, 0.000000000000000000, 1.000000000000000000 ) ) ;
#100658=VECTOR ( 'NONE', #87099, 1000.000000000000000 ) ;
#100664=CARTESIAN_POINT ( 'NONE',  ( 2.494940289813108780, 3.447199233515649386, -11.73777120880564695 ) ) ;
#100696=CARTESIAN_POINT ( 'NONE',  ( 8.966533317356120136, 1.405705671057797090, 7.975201661134141418 ) ) ;
#100737=DIRECTION ( 'NONE',  ( 0.9998476951563912696, 0.000000000000000000, -0.01745240643728004568 ) ) ;
#100809=EDGE_CURVE ( 'NONE', #194999, #175582, #111182, .T. ) ;
#100812=ORIENTED_EDGE ( 'NONE', *, *, #2389, .T. ) ;
#100842=ORIENTED_EDGE ( 'NONE', *, *, #53099, .F. ) ;
#100848=ORIENTED_EDGE ( 'NONE', *, *, #136119, .T. ) ;
#100890=LINE ( 'NONE', #16426, #77099 ) ;
#100901=DIRECTION ( 'NONE',  ( 0.000000000000000000, 1.000000000000000000, 0.000000000000000000 ) ) ;
#100931=CARTESIAN_POINT ( 'NONE',  ( 0.000000000000000000, 1.000000000000000888, 0.000000000000000000 ) ) ;
#100951=VERTEX_POINT ( 'NONE', #91692 ) ;
#100964=CARTESIAN_POINT ( 'NONE',  ( -6.745710774231114648, -7.818797203689479502, -6.689804758640219617 ) ) ;
#100988=DIRECTION ( 'NONE',  ( 0.000000000000000000, 0.000000000000000000, 1.000000000000000000 ) ) ;
#100996=CARTESIAN_POINT ( 'NONE',  ( 10.99950989413227909, -9.915617157791128733, -0.1038368378055223862 ) ) ;
#101000=CARTESIAN_POINT ( 'NONE',  ( 7.011678565220082149, -6.606405293530973388, -6.580818069395332870 ) ) ;
#101032=DIRECTION ( 'NONE',  ( 0.000000000000000000, 0.000000000000000000, 1.000000000000000000 ) ) ;
#101034=DIRECTION ( 'NONE',  ( 0.000000000000000000, 1.000000000000000000, 0.000000000000000000 ) ) ;
#101038=AXIS2_PLACEMENT_3D ( 'NONE', #42112, #192579, #108224 ) ;
#101058=ADVANCED_FACE ( 'NONE', ( #158799 ), #61861, .T. ) ;
#101118=CARTESIAN_POINT ( 'NONE',  ( -7.362820735710029041, -5.796536394784445712, -7.362820735712818809 ) ) ;
#101127=CARTESIAN_POINT ( 'NONE',  ( 6.761669295867161367, -7.008190897455697232, 6.673079560224753237 ) ) ;
#101142=CARTESIAN_POINT ( 'NONE',  ( 10.38614328979755719, 3.507114751586604129, -5.996442624206805405 ) ) ;
#101175=EDGE_CURVE ( 'NONE', #72492, #49868, #199548, .T. ) ;
#101185=CARTESIAN_POINT ( 'NONE',  ( 0.07933194154487546723, -7.609852571077992067, -9.499668754385622194 ) ) ;
#101243=AXIS2_PLACEMENT_3D ( 'NONE', #3472, #181182, #100988 ) ;
#101248=CARTESIAN_POINT ( 'NONE',  ( -6.729185449012799580, -6.864242550357221972, -6.701130152864378076 ) ) ;
#101364=CARTESIAN_POINT ( 'NONE',  ( -0.2582262029270495085, -8.187798858731225593, -9.496816297611141877 ) ) ;
#101405=EDGE_CURVE ( 'NONE', #62943, #133392, #161645, .T. ) ;
#101406=STYLED_ITEM ( 'NONE', ( #156264 ), #179324 ) ;
#101447=CARTESIAN_POINT ( 'NONE',  ( -1.084202172485504434E-15, -6.124285368610756564, -10.93005900551661114 ) ) ;
#101463=ORIENTED_EDGE ( 'NONE', *, *, #184050, .T. ) ;
#101467=ORIENTED_EDGE ( 'NONE', *, *, #165594, .T. ) ;
#101473=CARTESIAN_POINT ( 'NONE',  ( 10.99943592164172657, -9.999999999999994671, -0.1113975120798811613 ) ) ;
#101480=FACE_OUTER_BOUND ( 'NONE', #173876, .T. ) ;
#101515=CARTESIAN_POINT ( 'NONE',  ( -6.830415307812264025, -7.473374494058229622, -6.717278222822378630 ) ) ;
#101554=CARTESIAN_POINT ( 'NONE',  ( -6.773376349083143566, -7.473374494058229622, -6.661184041420940005 ) ) ;
#101562=DIRECTION ( 'NONE',  ( 0.000000000000000000, 0.000000000000000000, -1.000000000000000000 ) ) ;
#101563=PRESENTATION_STYLE_ASSIGNMENT (( #117880 ) ) ;
#101618=ORIENTED_EDGE ( 'NONE', *, *, #184338, .T. ) ;
#101646=SURFACE_SIDE_STYLE ('',( #35565 ) ) ;
#101658=ORIENTED_EDGE ( 'NONE', *, *, #186479, .T. ) ;
#101678=AXIS2_PLACEMENT_3D ( 'NONE', #117114, #99738, #83477 ) ;
#101693=EDGE_CURVE ( 'NONE', #31452, #157630, #175475, .T. ) ;
#101708=CARTESIAN_POINT ( 'NONE',  ( 9.499668754385636404, 7.849261790823902629, 0.07933194154488391880 ) ) ;
#101732=CARTESIAN_POINT ( 'NONE',  ( 10.30923643716952576, 0.9706168436483885165, 5.952040432139194870 ) ) ;
#101760=ORIENTED_EDGE ( 'NONE', *, *, #203182, .T. ) ;
#101761=B_SPLINE_CURVE_WITH_KNOTS ( 'NONE', 3,
 ( #113625, #14956, #30172, #161244, #96261, #78905, #195874 ),
 .UNSPECIFIED., .F., .F.,
 ( 4, 3, 4 ),
 ( 3.315837474970529026E-05, 0.0009000000035470258212, 0.001929259801299062485 ),
 .UNSPECIFIED. ) ;
#101763=CARTESIAN_POINT ( 'NONE',  ( -0.07933194151890057833, -9.902237888914269703, -9.499668754386311420 ) ) ;
#101773=CARTESIAN_POINT ( 'NONE',  ( -7.228805602686602327, -7.003075417673644054, -7.884707905546937567 ) ) ;
#101779=CARTESIAN_POINT ( 'NONE',  ( 10.96314634606097016, -7.723163831703883986, -0.5532327639488858750 ) ) ;
#101790=CARTESIAN_POINT ( 'NONE',  ( -9.496912337248829772, -9.201070920843589462, 0.2456386449429323604 ) ) ;
#101797=DIRECTION ( 'NONE',  ( 0.000000000000000000, 0.000000000000000000, -1.000000000000000000 ) ) ;
#101812=ORIENTED_EDGE ( 'NONE', *, *, #11694, .T. ) ;
#101813=CARTESIAN_POINT ( 'NONE',  ( 9.242574560015899721, -9.438200158419393304, -0.5964493340168087743 ) ) ;
#101829=CIRCLE ( 'NONE', #198743, 9.499999999999992895 ) ;
#101868=MECHANICAL_DESIGN_GEOMETRIC_PRESENTATION_REPRESENTATION('',(#5044),#147352);
#101879=EDGE_CURVE ( 'NONE', #166808, #207703, #192753, .T. ) ;
#101887=AXIS2_PLACEMENT_3D ( 'NONE', #164517, #117961, #182888 ) ;
#101889=ORIENTED_EDGE ( 'NONE', *, *, #154559, .T. ) ;
#101909=CARTESIAN_POINT ( 'NONE',  ( 7.778383330260339790, -5.907420853759298041, -7.778383330260368211 ) ) ;
#101913=ORIENTED_EDGE ( 'NONE', *, *, #65438, .F. ) ;
#101925=VERTEX_POINT ( 'NONE', #162664 ) ;
#101966=DIRECTION ( 'NONE',  ( -0.000000000000000000, 1.000000000000000000, -0.000000000000000000 ) ) ;
#101994=CARTESIAN_POINT ( 'NONE',  ( -8.830779531597137577, 3.974415841077566292, -7.430925027917930414 ) ) ;
#101997=VERTEX_POINT ( 'NONE', #145383 ) ;
#102025=DIRECTION ( 'NONE',  ( 0.000000000000000000, 1.000000000000000000, 0.000000000000000000 ) ) ;
#102028=CARTESIAN_POINT ( 'NONE',  ( 6.381095703207991576, -8.233137084989849086, 7.037870247915948063 ) ) ;
#102042=CARTESIAN_POINT ( 'NONE',  ( -4.792515913634093623E-13, -7.868798029037626485, 9.500000000000001776 ) ) ;
#102049=EDGE_CURVE ( 'NONE', #177991, #91101, #57796, .T. ) ;
#102051=CARTESIAN_POINT ( 'NONE',  ( 1.270994156678442596E-16, -6.530144695498194096, -11.00000000000000178 ) ) ;
#102062=CARTESIAN_POINT ( 'NONE',  ( 10.79929312474867942, -8.526088927970997489, -0.1885023626713021039 ) ) ;
#102069=CARTESIAN_POINT ( 'NONE',  ( 0.1899713450103265033, -8.048696291100959854, 9.532262708098286907 ) ) ;
#102076=CARTESIAN_POINT ( 'NONE',  ( 0.3866937364864087567, 3.956598013261175772, -11.53692321988872926 ) ) ;
#102102=ORIENTED_EDGE ( 'NONE', *, *, #198854, .T. ) ;
#102111=B_SPLINE_CURVE_WITH_KNOTS ( 'NONE', 3,
 ( #129745, #180534, #32156, #162170, #66741, #213015, #81962, #164289, #148047, #214055 ),
 .UNSPECIFIED., .F., .F.,
 ( 4, 2, 2, 2, 4 ),
 ( 1.904249188897462635E-17, 0.0002021113321160430986, 0.0004042226642320671153, 0.0006063339963480911862, 0.0008084453284641152570 ),
 .UNSPECIFIED. ) ;
#102136=EDGE_CURVE ( 'NONE', #200016, #119366, #90615, .T. ) ;
#102156=CARTESIAN_POINT ( 'NONE',  ( -0.3870735955438814879, 1.000000000000000888, 11.88799243440809050 ) ) ;
#102177=ORIENTED_EDGE ( 'NONE', *, *, #117997, .T. ) ;
#102252=FACE_OUTER_BOUND ( 'NONE', #6255, .T. ) ;
#102260=CARTESIAN_POINT ( 'NONE',  ( 6.595517585942704208, -7.896420114628012854, 7.253242555595321051 ) ) ;
#102286=EDGE_CURVE ( 'NONE', #14247, #14615, #188803, .T. ) ;
#102304=EDGE_LOOP ( 'NONE', ( #94404, #142148, #115106, #85853 ) ) ;
#102317=CARTESIAN_POINT ( 'NONE',  ( -6.653311379900198830, -6.675176078274440705, -6.940534579975141227 ) ) ;
#102381=ORIENTED_EDGE ( 'NONE', *, *, #54983, .T. ) ;
#102388=CARTESIAN_POINT ( 'NONE',  ( 10.23203630735456393, -6.594478602028841507, -1.760317133499381158E-15 ) ) ;
#102407=B_SPLINE_CURVE_WITH_KNOTS ( 'NONE', 3,
 ( #31759, #99943, #128277, #29621, #50130, #33865, #12275, #78351, #178005, #132483, #114140, #162827, #97830, #163895, #144474, #148698 ),
 .UNSPECIFIED., .F., .F.,
 ( 4, 3, 3, 3, 3, 4 ),
 ( 0.000000000000000000, 4.381999914579370578E-06, 1.110488615493398738E-05, 1.784390311306881054E-05, 2.460054645147356366E-05, 3.136851507421863007E-05 ),
 .UNSPECIFIED. ) ;
#102414=CARTESIAN_POINT ( 'NONE',  ( 10.42995565840374184, 1.000000000000000888, -5.797106512947759249 ) ) ;
#102432=EDGE_CURVE ( 'NONE', #31312, #94484, #129432, .T. ) ;
#102475=VERTEX_POINT ( 'NONE', #139769 ) ;
#102514=CARTESIAN_POINT ( 'NONE',  ( -7.985752187169337546, -6.863172033215962031, 7.565242077046661073 ) ) ;
#102517=CARTESIAN_POINT ( 'NONE',  ( -10.34545848478754593, -8.336144560139965520, 0.6172425113790593887 ) ) ;
#102572=CARTESIAN_POINT ( 'NONE',  ( -8.044078759455166150, -6.893137084989842123, 7.385065802799744894 ) ) ;
#102605=DIRECTION ( 'NONE',  ( 0.000000000000000000, 0.000000000000000000, -1.000000000000000000 ) ) ;
#102637=TOROIDAL_SURFACE ( 'NONE', #61200, 9.580000000000001847, 0.08000000000000000167 ) ;
#102667=EDGE_CURVE ( 'NONE', #18903, #129023, #172061, .T. ) ;
#102670=CARTESIAN_POINT ( 'NONE',  ( 3.176185322659801230E-15, -5.758458176070770485, 10.93186801223271587 ) ) ;
#102720=SURFACE_SIDE_STYLE ('',( #132058 ) ) ;
#102804=CARTESIAN_POINT ( 'NONE',  ( 0.000000000000000000, 0.000000000000000000, 0.000000000000000000 ) ) ;
#102849=ADVANCED_FACE ( 'NONE', ( #12918 ), #111905, .F. ) ;
#102878=CARTESIAN_POINT ( 'NONE',  ( -10.99970480893081870, -6.134628647623513231, -0.08058608058607828750 ) ) ;
#102885=CARTESIAN_POINT ( 'NONE',  ( 10.98598255107576271, -7.721050908199750040, -0.1917610387292519314 ) ) ;
#102908=CYLINDRICAL_SURFACE ( 'NONE', #140889, 0.08000000000000020983 ) ;
#102911=CARTESIAN_POINT ( 'NONE',  ( -0.4294425147611471982, -9.006862915010142245, 9.490288674561782045 ) ) ;
#102912=EDGE_CURVE ( 'NONE', #204799, #169582, #23443, .T. ) ;
#102930=EDGE_CURVE ( 'NONE', #94234, #115982, #162405, .T. ) ;
#102951=CARTESIAN_POINT ( 'NONE',  ( 9.837588353260175111, -6.372041098633662415, -9.403289436706798103E-13 ) ) ;
#102997=B_SPLINE_CURVE_WITH_KNOTS ( 'NONE', 3,
 ( #71125, #137241, #205404, #203263 ),
 .UNSPECIFIED., .F., .F.,
 ( 4, 4 ),
 ( 0.000000000000000000, 6.033646489354907845E-05 ),
 .UNSPECIFIED. ) ;
#103014=ORIENTED_EDGE ( 'NONE', *, *, #64072, .T. ) ;
#103023=CARTESIAN_POINT ( 'NONE',  ( -1.048552960303294919E-14, -9.091017468556975345, -10.23550087314634993 ) ) ;
#103030=ORIENTED_EDGE ( 'NONE', *, *, #117446, .T. ) ;
#103036=CARTESIAN_POINT ( 'NONE',  ( 9.481348452320370157, -9.006862915010128035, -0.5950054837411730135 ) ) ;
#103041=CARTESIAN_POINT ( 'NONE',  ( -9.579665964948882007, -7.473374494045003757, 5.204170427930421283E-15 ) ) ;
#103043=DIRECTION ( 'NONE',  ( 0.000000000000000000, 1.000000000000000000, 0.000000000000000000 ) ) ;
#103068=( GEOMETRIC_REPRESENTATION_CONTEXT ( 3 ) GLOBAL_UNCERTAINTY_ASSIGNED_CONTEXT ( ( #174125 ) ) GLOBAL_UNIT_ASSIGNED_CONTEXT ( ( #67169, #162586, #199309 ) ) REPRESENTATION_CONTEXT ( 'NONE', 'WORKASPACE' ) );
#103086=CARTESIAN_POINT ( 'NONE',  ( 10.30245174296169175, 3.603753425775775288, -5.948123287112220936 ) ) ;
#103102=CARTESIAN_POINT ( 'NONE',  ( 1.697517146273963306E-12, -6.372041098632814204, 9.837588353259947738 ) ) ;
#103105=ORIENTED_EDGE ( 'NONE', *, *, #184735, .F. ) ;
#103109=CARTESIAN_POINT ( 'NONE',  ( 0.1963700886235890397, -6.681311647492909067, 9.612263720970508629 ) ) ;
#103110=CARTESIAN_POINT ( 'NONE',  ( 0.4644097342742965484, -8.233137084989849086, 9.488641820551103834 ) ) ;
#103117=CARTESIAN_POINT ( 'NONE',  ( -6.649736275991368295, -8.039737506397923283, -6.784764760059130317 ) ) ;
#103140=CARTESIAN_POINT ( 'NONE',  ( -10.91132967064557491, -5.166862915010145052, 0.4350687514514811616 ) ) ;
#103145=CARTESIAN_POINT ( 'NONE',  ( 10.99943592164171235, -9.901472394401615418, -0.1113975120799817059 ) ) ;
#103169=CARTESIAN_POINT ( 'NONE',  ( -0.009341296487041779104, -9.943660733012633202, -9.579650209538295158 ) ) ;
#103175=( BOUNDED_SURFACE ( )  B_SPLINE_SURFACE ( 3, 2, ( 
 ( #199632, #119536, #104297 ),
 ( #68561, #17675, #38224 ),
 ( #154111, #168223, #19822 ),
 ( #70688, #83761, #203894 ) ),
 .UNSPECIFIED., .F., .F., .T. ) 
 B_SPLINE_SURFACE_WITH_KNOTS ( ( 4, 4 ),
 ( 3, 3 ),
 ( 0.000000000000000000, 3.124373657233979538E-05 ),
 ( 0.000000000000000000, 1.000000000000000000 ),
 .UNSPECIFIED. ) 
 GEOMETRIC_REPRESENTATION_ITEM ( )  RATIONAL_B_SPLINE_SURFACE ( (
 ( 1.000000000000000000, 0.7045118851641305469, 1.000000000000000000),
 ( 1.000000000000000000, 0.7044892147945193139, 1.000000000000000000),
 ( 1.000000000000000000, 0.7053501046726611268, 1.000000000000000000),
 ( 1.000000000000000000, 0.7071067811869123920, 1.000000000000000000) ) ) 
 REPRESENTATION_ITEM ( '' )  SURFACE ( )  );
#103185=CARTESIAN_POINT ( 'NONE',  ( 0.000000000000000000, 4.000000000000003553, 6.450000000000003730 ) ) ;
#103227=CARTESIAN_POINT ( 'NONE',  ( -0.1945363205450327815, 1.000000000000000888, 11.93115981699678585 ) ) ;
#103237=ORIENTED_EDGE ( 'NONE', *, *, #93674, .F. ) ;
#103248=LINE ( 'NONE', #4635, #64264 ) ;
#103265=EDGE_CURVE ( 'NONE', #204799, #206986, #30282, .T. ) ;
#103280=CARTESIAN_POINT ( 'NONE',  ( 6.447267651612376582, -6.532648833121157850, 6.949925879317534694 ) ) ;
#103281=ORIENTED_EDGE ( 'NONE', *, *, #203182, .F. ) ;
#103298=VERTEX_POINT ( 'NONE', #192490 ) ;
#103363=CARTESIAN_POINT ( 'NONE',  ( -10.99370838174331055, -6.893137084989843011, 0.3821126922044791874 ) ) ;
#103392=CARTESIAN_POINT ( 'NONE',  ( -6.710127771514629025, -7.162053774861991684, -6.725445687907746439 ) ) ;
#103401=DIRECTION ( 'NONE',  ( 0.000000000000000000, 1.000000000000000000, 0.000000000000000000 ) ) ;
#103458=FACE_OUTER_BOUND ( 'NONE', #193774, .T. ) ;
#103623=EDGE_CURVE ( 'NONE', #21223, #51705, #139720, .T. ) ;
#103648=EDGE_LOOP ( 'NONE', ( #191698, #86737, #29677, #104129 ) ) ;
#103649=B_SPLINE_CURVE_WITH_KNOTS ( 'NONE', 3,
 ( #143040, #157131, #139824, #207981, #9788, #140906, #159240 ),
 .UNSPECIFIED., .F., .F.,
 ( 4, 3, 4 ),
 ( 0.000000000000000000, 0.0008000000000004422844, 0.002977368225425622381 ),
 .UNSPECIFIED. ) ;
#103651=DIRECTION ( 'NONE',  ( 0.7366372490352351976, 0.000000000000000000, -0.6762880771785058087 ) ) ;
#103654=ORIENTED_EDGE ( 'NONE', *, *, #43529, .F. ) ;
#103679=CARTESIAN_POINT ( 'NONE',  ( 0.000000000000000000, -7.666862915010147717, 0.000000000000000000 ) ) ;
#103712=CARTESIAN_POINT ( 'NONE',  ( 0.000000000000000000, -6.893137084989842123, 0.000000000000000000 ) ) ;
#103801=CARTESIAN_POINT ( 'NONE',  ( -9.499050059654539524, -8.104757123234332283, 0.1520312049661968479 ) ) ;
#103816=FILL_AREA_STYLE_COLOUR ( '', #74065 ) ;
#103833=CARTESIAN_POINT ( 'NONE',  ( -0.2039282260588116402, -6.674536912880628670, -9.612297698795913448 ) ) ;
#103846=CARTESIAN_POINT ( 'NONE',  ( -0.4373225248172925017, -7.723431457505085085, 10.96785329849814339 ) ) ;
#103866=EDGE_CURVE ( 'NONE', #119366, #90575, #62269, .T. ) ;
#103905=ORIENTED_EDGE ( 'NONE', *, *, #182674, .F. ) ;
#103907=CARTESIAN_POINT ( 'NONE',  ( 7.796438949605505542, -6.657020681837042986, -7.586009164902113078 ) ) ;
#103916=B_SPLINE_CURVE_WITH_KNOTS ( 'NONE', 3,
 ( #144123, #194951, #28187, #128972, #45525, #63883 ),
 .UNSPECIFIED., .F., .F.,
 ( 4, 2, 4 ),
 ( 0.000000000000000000, 0.001226111284895915884, 0.002452222569791831334 ),
 .UNSPECIFIED. ) ;
#103917=CARTESIAN_POINT ( 'NONE',  ( 0.2680151545362241539, -6.654245765634851928, 10.99740610014212550 ) ) ;
#103934=CARTESIAN_POINT ( 'NONE',  ( -10.93020303578476415, -8.258458176070773149, 0.1907874036681941887 ) ) ;
#103986=CARTESIAN_POINT ( 'NONE',  ( 0.000000000000000000, 0.000000000000000000, 0.000000000000000000 ) ) ;
#104018=CARTESIAN_POINT ( 'NONE',  ( 0.000000000000000000, -9.999999999999994671, 10.99999999999999112 ) ) ;
#104032=ORIENTED_EDGE ( 'NONE', *, *, #211265, .T. ) ;
#104050=CARTESIAN_POINT ( 'NONE',  ( -6.949550370341250449, -6.532648880269213088, 6.447678837262236229 ) ) ;
#104106=CARTESIAN_POINT ( 'NONE',  ( 11.41267819554179042, 4.000000000000003553, -3.708203932499494648 ) ) ;
#104123=DIRECTION ( 'NONE',  ( 0.000000000000000000, 0.000000000000000000, 1.000000000000000000 ) ) ;
#104129=ORIENTED_EDGE ( 'NONE', *, *, #49388, .F. ) ;
#104131=DIRECTION ( 'NONE',  ( -0.9983585005135560131, 0.000000000000000000, 0.05727394217551282085 ) ) ;
#104147=ORIENTED_EDGE ( 'NONE', *, *, #127031, .F. ) ;
#104166=DIRECTION ( 'NONE',  ( 0.000000000000000000, 1.000000000000000000, 0.000000000000000000 ) ) ;
#104174=CARTESIAN_POINT ( 'NONE',  ( 2.057629584373536602, 2.441452740530747789, -11.54123292161950687 ) ) ;
#104191=CARTESIAN_POINT ( 'NONE',  ( -10.99962150373186809, -9.919999999999998153, 0.09125116240079125807 ) ) ;
#104196=CARTESIAN_POINT ( 'NONE',  ( -9.500385102287573602, -7.162053774861992572, 0.01083140255525650089 ) ) ;
#104201=EDGE_CURVE ( 'NONE', #149524, #108531, #103649, .T. ) ;
#104217=DIRECTION ( 'NONE',  ( 0.9998476951563912696, 0.000000000000000000, -0.01745240643728004568 ) ) ;
#104244=CARTESIAN_POINT ( 'NONE',  ( -0.09263630470260257599, -10.00000000000047251, -9.579493439010613898 ) ) ;
#104249=VERTEX_POINT ( 'NONE', #41254 ) ;
#104297=CARTESIAN_POINT ( 'NONE',  ( 0.08058608058607380498, -9.900000000000005684, 10.99970480893082225 ) ) ;
#104306=DIRECTION ( 'NONE',  ( 0.000000000000000000, -1.000000000000000000, 0.000000000000000000 ) ) ;
#104423=CARTESIAN_POINT ( 'NONE',  ( -2.331034670843834533E-15, -9.756397064627583049, -9.569424307476229075 ) ) ;
#104440=EDGE_CURVE ( 'NONE', #19069, #44666, #64895, .T. ) ;
#104468=CARTESIAN_POINT ( 'NONE',  ( 10.98676690055266114, -7.666862915010303148, -0.5459353850038921596 ) ) ;
#104469=CARTESIAN_POINT ( 'NONE',  ( 0.000000000000000000, 1.000000000000000888, 0.000000000000000000 ) ) ;
#104478=CARTESIAN_POINT ( 'NONE',  ( 0.000000000000000000, 7.849261790823902629, 0.000000000000000000 ) ) ;
#104516=CARTESIAN_POINT ( 'NONE',  ( -0.1000000000000028644, -9.900000000000005684, 0.000000000000000000 ) ) ;
#104535=CARTESIAN_POINT ( 'NONE',  ( -10.89423718502888860, -6.453216945989406206, 0.03415196713902314551 ) ) ;
#104630=CARTESIAN_POINT ( 'NONE',  ( 10.99943592164172657, -8.407420853759269619, -0.1113975120798851026 ) ) ;
#104651=CARTESIAN_POINT ( 'NONE',  ( -9.602438852202270780, -9.449361760816694655, 0.1964824153909955906 ) ) ;
#104687=ORIENTED_EDGE ( 'NONE', *, *, #178265, .F. ) ;
#104691=CARTESIAN_POINT ( 'NONE',  ( -10.91944941500665678, -9.999999999999994671, 0.1017788107271379444 ) ) ;
#104695=CARTESIAN_POINT ( 'NONE',  ( 0.4359479416626659276, -6.334709917115469935, 9.855659161987908590 ) ) ;
#104698=ADVANCED_FACE ( 'NONE', ( #44388 ), #77934, .T. ) ;
#104724=DIRECTION ( 'NONE',  ( 0.6762880771785059197, 1.295290445962756284E-12, 0.7366372490352354196 ) ) ;
#104733=LINE ( 'NONE', #202181, #132088 ) ;
#104790=ORIENTED_EDGE ( 'NONE', *, *, #93999, .T. ) ;
#104801=CARTESIAN_POINT ( 'NONE',  ( -10.99962150373186631, -9.999999999999880984, 0.09125116240080800856 ) ) ;
#104828=AXIS2_PLACEMENT_3D ( 'NONE', #143397, #109860, #14399 ) ;
#104906=B_SPLINE_CURVE_WITH_KNOTS ( 'NONE', 3,
 ( #35114, #101185, #120729, #2601 ),
 .UNSPECIFIED., .F., .F.,
 ( 4, 4 ),
 ( 0.000000000000000000, 0.0004037790303856098246 ),
 .UNSPECIFIED. ) ;
#104912=CARTESIAN_POINT ( 'NONE',  ( 0.06269018847613376522, -7.008739397177144781, -9.499801640457381069 ) ) ;
#104921=CARTESIAN_POINT ( 'NONE',  ( 8.876521693626907350, 3.555461883994700756, 7.992456032239036112 ) ) ;
#104924=CARTESIAN_POINT ( 'NONE',  ( -0.1172869779874923940, -7.889939693150851419, 10.99948653685772548 ) ) ;
#104969=DIRECTION ( 'NONE',  ( -0.000000000000000000, -1.000000000000000000, -0.000000000000000000 ) ) ;
#104976=CARTESIAN_POINT ( 'NONE',  ( -3.672734859294646270E-15, -9.900000000000005684, -9.579665964948937074 ) ) ;
#104982=EDGE_LOOP ( 'NONE', ( #91397, #172478, #142590, #121455 ) ) ;
#104984=FACE_OUTER_BOUND ( 'NONE', #147347, .T. ) ;
#105000=ADVANCED_FACE ( 'NONE', ( #66987 ), #140970, .T. ) ;
#105026=CARTESIAN_POINT ( 'NONE',  ( -10.41272866534590591, -5.796408561411221072, -4.392600644672434268E-13 ) ) ;
#105039=CARTESIAN_POINT ( 'NONE',  ( -10.36939107341403776, 1.813436143228261521, -6.039542801432668639 ) ) ;
#105056=SURFACE_SIDE_STYLE ('',( #36819 ) ) ;
#105101=EDGE_CURVE ( 'NONE', #114840, #12663, #72334, .T. ) ;
#105103=CIRCLE ( 'NONE', #84200, 6.329999999999995630 ) ;
#105109=ORIENTED_EDGE ( 'NONE', *, *, #62295, .F. ) ;
#105133=ORIENTED_EDGE ( 'NONE', *, *, #201199, .T. ) ;
#105154=EDGE_CURVE ( 'NONE', #72609, #205917, #79822, .T. ) ;
#105171=PLANE ( 'NONE',  #109323 ) ;
#105174=CARTESIAN_POINT ( 'NONE',  ( -8.081892667527540652, -5.200000000000006395, 7.462104991928527831 ) ) ;
#105189=CARTESIAN_POINT ( 'NONE',  ( 9.532262708098283355, -8.048696291100949196, -0.1899713450103259760 ) ) ;
#105191=DIRECTION ( 'NONE',  ( -0.9999753971658824625, 0.000000000000000000, 0.007014632059889242682 ) ) ;
#105212=CARTESIAN_POINT ( 'NONE',  ( -6.849482339516217877, -6.938199013094648038, 6.234224025626350141 ) ) ;
#105213=DIRECTION ( 'NONE',  ( 0.000000000000000000, 1.000000000000000000, 0.000000000000000000 ) ) ;
#105215=CARTESIAN_POINT ( 'NONE',  ( -7.834948813059765094, -6.306565840633504116, -7.720982910014320133 ) ) ;
#105238=ADVANCED_FACE ( 'NONE', ( #148411 ), #199250, .T. ) ;
#105248=CARTESIAN_POINT ( 'NONE',  ( 6.980013479859856318, -8.233136965322191969, -6.444907381559382031 ) ) ;
#105250=CARTESIAN_POINT ( 'NONE',  ( 2.026920941591049630, 3.691791674785623201, -11.39597588158938990 ) ) ;
#105253=VERTEX_POINT ( 'NONE', #198193 ) ;
#105271=AXIS2_PLACEMENT_3D ( 'NONE', #71054, #68921, #133993 ) ;
#105282=B_SPLINE_CURVE_WITH_KNOTS ( 'NONE', 3,
 ( #133796, #119705, #199805, #2656 ),
 .UNSPECIFIED., .F., .F.,
 ( 4, 4 ),
 ( 0.000000000000000000, 6.033646489354555479E-05 ),
 .UNSPECIFIED. ) ;
#105285=EDGE_LOOP ( 'NONE', ( #104032, #93184, #94869, #136140 ) ) ;
#105291=CARTESIAN_POINT ( 'NONE',  ( 0.3602790413719210716, -9.063128419003717795, -9.630430012830139219 ) ) ;
#105319=B_SPLINE_CURVE_WITH_KNOTS ( 'NONE', 3,
 ( #54236, #34765, #4376, #68321 ),
 .UNSPECIFIED., .F., .F.,
 ( 4, 4 ),
 ( 0.000000000000000000, 8.505390838612172152E-05 ),
 .UNSPECIFIED. ) ;
#105331=EDGE_LOOP ( 'NONE', ( #147594, #93494, #86324, #153113 ) ) ;
#105383=ORIENTED_EDGE ( 'NONE', *, *, #189331, .F. ) ;
#105386=FILL_AREA_STYLE ('',( #7840 ) ) ;
#105396=CARTESIAN_POINT ( 'NONE',  ( -0.1980946632348522529, -8.057097448493959035, -9.531438498077047683 ) ) ;
#105422=AXIS2_PLACEMENT_3D ( 'NONE', #115197, #49077, #181190 ) ;
#105465=CARTESIAN_POINT ( 'NONE',  ( 6.770610912236886492, -7.154544010627095219, 6.663994888585879295 ) ) ;
#105538=CARTESIAN_POINT ( 'NONE',  ( 6.725445687907758874, -7.162053774861991684, -6.710127771514625472 ) ) ;
#105548=( BOUNDED_SURFACE ( )  B_SPLINE_SURFACE ( 3, 2, ( 
 ( #176838, #13262, #12190 ),
 ( #63083, #78261, #195223 ),
 ( #99853, #81469, #178985 ),
 ( #116157, #148605, #165915 ) ),
 .UNSPECIFIED., .F., .F., .T. ) 
 B_SPLINE_SURFACE_WITH_KNOTS ( ( 4, 4 ),
 ( 3, 3 ),
 ( 0.01090518310586315390, 0.01337341879808987347 ),
 ( 0.000000000000000000, 1.000000000000000000 ),
 .UNSPECIFIED. ) 
 GEOMETRIC_REPRESENTATION_ITEM ( )  RATIONAL_B_SPLINE_SURFACE ( (
 ( 1.000000000000000000, 0.6967468848055796693, 1.000000000000000000),
 ( 1.000000000000000000, 0.6961913616436852248, 1.000000000000000000),
 ( 1.000000000000000000, 0.6955505937921927506, 1.000000000000000000),
 ( 1.000000000000000000, 0.6947640035364115452, 1.000000000000000000) ) ) 
 REPRESENTATION_ITEM ( '' )  SURFACE ( )  );
#105559=CARTESIAN_POINT ( 'NONE',  ( 7.750016138724922676, -6.480061791515691283, -7.806764249273701495 ) ) ;
#105571=CARTESIAN_POINT ( 'NONE',  ( 0.09775709102116830751, -9.919835437265270173, 10.99956570265433697 ) ) ;
#105584=CARTESIAN_POINT ( 'NONE',  ( 9.000007961041747606, 1.000000000000000888, 7.937244906211794238 ) ) ;
#105601=CIRCLE ( 'NONE', #116155, 11.54340198673881979 ) ;
#105616=STYLED_ITEM ( 'NONE', ( #10624 ), #87466 ) ;
#105621=CARTESIAN_POINT ( 'NONE',  ( -10.86152993230177621, -6.808378554901812763, 0.3183146091066173522 ) ) ;
#105648=UNCERTAINTY_MEASURE_WITH_UNIT (LENGTH_MEASURE( 1.000000000000000082E-05 ), #70788, 'distance_accuracy_value', 'NONE');
#105685=ADVANCED_FACE ( 'NONE', ( #45316 ), #59315, .T. ) ;
#105698=ORIENTED_EDGE ( 'NONE', *, *, #83989, .F. ) ;
#105708=DIRECTION ( 'NONE',  ( 0.000000000000000000, 0.000000000000000000, -1.000000000000000000 ) ) ;
#105716=CARTESIAN_POINT ( 'NONE',  ( 10.98974895236967164, -7.729832900979586086, -0.4787367839867315844 ) ) ;
#105744=CARTESIAN_POINT ( 'NONE',  ( -9.578206935409053102, -9.746166700193986898, 0.1671882239534360770 ) ) ;
#105774=EDGE_CURVE ( 'NONE', #50087, #28024, #149658, .T. ) ;
#105787=CARTESIAN_POINT ( 'NONE',  ( -10.91804383151480806, -9.907361309732431565, 0.1905751639681794174 ) ) ;
#105800=CARTESIAN_POINT ( 'NONE',  ( 2.450294804891584022, 1.972237431424222809, -11.52773071619440692 ) ) ;
#105858=CARTESIAN_POINT ( 'NONE',  ( 10.93005900490892834, -6.124285369217931319, 9.269928574751062911E-15 ) ) ;
#105881=DIRECTION ( 'NONE',  ( -0.000000000000000000, -1.000000000000000000, -0.000000000000000000 ) ) ;
#105884=VERTEX_POINT ( 'NONE', #50626 ) ;
#105972=ORIENTED_EDGE ( 'NONE', *, *, #166038, .F. ) ;
#105978=CARTESIAN_POINT ( 'NONE',  ( -10.99931692196006949, -8.074346042903137288, 0.1488091642035881401 ) ) ;
#105983=EDGE_CURVE ( 'NONE', #113870, #118245, #113524, .T. ) ;
#105985=( LENGTH_UNIT ( ) NAMED_UNIT ( * ) SI_UNIT ( .MILLI., .METRE. ) );
#105990=PLANE ( 'NONE',  #34973 ) ;
#105994=( NAMED_UNIT ( * ) SI_UNIT ( $, .STERADIAN. ) SOLID_ANGLE_UNIT ( ) );
#106000=CARTESIAN_POINT ( 'NONE',  ( -6.901817408925782438, -6.554751161430547590, 6.500815859342965908 ) ) ;
#106081=ORIENTED_EDGE ( 'NONE', *, *, #11734, .T. ) ;
#106092=CARTESIAN_POINT ( 'NONE',  ( -6.794158526849257917, -7.616254850791395192, -7.451274665340245740 ) ) ;
#106099=CARTESIAN_POINT ( 'NONE',  ( 10.95855051086948251, -7.723431457505092190, -0.6286713519883923018 ) ) ;
#106109=DIRECTION ( 'NONE',  ( 0.000000000000000000, 1.000000000000000000, 0.000000000000000000 ) ) ;
#106193=CARTESIAN_POINT ( 'NONE',  ( -7.055228938194283650, -8.176568542494891290, 6.396834479292372144 ) ) ;
#106201=CIRCLE ( 'NONE', #192559, 9.500000000000001776 ) ;
#106224=DIRECTION ( 'NONE',  ( 0.9988044021632734859, 0.000000000000000000, -0.04888523518676873847 ) ) ;
#106268=CARTESIAN_POINT ( 'NONE',  ( 0.000000000000000000, 0.000000000000000000, 0.000000000000000000 ) ) ;
#106329=B_SPLINE_CURVE_WITH_KNOTS ( 'NONE', 3,
 ( #150748, #2309, #21188, #87291, #202065, #153360, #168540, #37468 ),
 .UNSPECIFIED., .F., .F.,
 ( 4, 2, 2, 4 ),
 ( 3.245370453949652856E-18, 0.0002034531274099211061, 0.0004069062548198396100, 0.0008138125096396765096 ),
 .UNSPECIFIED. ) ;
#106351=FACE_OUTER_BOUND ( 'NONE', #126934, .T. ) ;
#106383=ORIENTED_EDGE ( 'NONE', *, *, #167891, .T. ) ;
#106388=CARTESIAN_POINT ( 'NONE',  ( 0.000000000000000000, -7.473374494045017968, 9.579665964948883783 ) ) ;
#106413=EDGE_CURVE ( 'NONE', #36647, #108269, #173085, .T. ) ;
#106476=ORIENTED_EDGE ( 'NONE', *, *, #195653, .F. ) ;
#106484=FILL_AREA_STYLE ('',( #39297 ) ) ;
#106489=CARTESIAN_POINT ( 'NONE',  ( -0.4644097342743090384, -8.200000000000015277, -9.488641820551084294 ) ) ;
#106512=DIRECTION ( 'NONE',  ( 0.000000000000000000, 0.000000000000000000, 1.000000000000000000 ) ) ;
#106554=CARTESIAN_POINT ( 'NONE',  ( 7.721398836998401904, -6.134628647623499909, 7.721398836998376147 ) ) ;
#106561=ADVANCED_FACE ( 'NONE', ( #47332 ), #39578, .T. ) ;
#106597=CARTESIAN_POINT ( 'NONE',  ( 10.99861980075107937, -9.900000000000074962, -0.1919816227428264854 ) ) ;
#106642=CARTESIAN_POINT ( 'NONE',  ( 0.000000000000000000, -8.176568542494905500, 0.000000000000000000 ) ) ;
#106660=CIRCLE ( 'NONE', #47901, 0.08000000000000018208 ) ;
#106666=EDGE_CURVE ( 'NONE', #167216, #45056, #2298, .T. ) ;
#106713=CARTESIAN_POINT ( 'NONE',  ( -10.99917004716958857, -6.764708007038216842, 0.1531059978909550534 ) ) ;
#106716=CARTESIAN_POINT ( 'NONE',  ( -2.530224277154541124, 2.018041202053984406, 11.90376931803457872 ) ) ;
#106729=CARTESIAN_POINT ( 'NONE',  ( -9.584291988782265292, -7.189630408304557463, 0.001123102408834306858 ) ) ;
#106743=VECTOR ( 'NONE', #190395, 1000.000000000000000 ) ;
#106781=CARTESIAN_POINT ( 'NONE',  ( 0.000000000000000000, -8.176568542494905500, 0.000000000000000000 ) ) ;
#106804=AXIS2_PLACEMENT_3D ( 'NONE', #54137, #35739, #149505 ) ;
#106815=EDGE_CURVE ( 'NONE', #68781, #45420, #133924, .T. ) ;
#106821=CARTESIAN_POINT ( 'NONE',  ( 11.40591166468351503, 3.507114751586604129, -3.706005353348470255 ) ) ;
#106826=CARTESIAN_POINT ( 'NONE',  ( -11.00006988736403102, -9.999999999999994671, 0.09199170129444225741 ) ) ;
#106849=CARTESIAN_POINT ( 'NONE',  ( -7.834948825496938163, -9.999999999999994671, -7.720982897393569466 ) ) ;
#106876=CARTESIAN_POINT ( 'NONE',  ( 2.421437874748389341, 3.696394713403123866, -11.55257195323928876 ) ) ;
#106908=EDGE_CURVE ( 'NONE', #42950, #176800, #178047, .T. ) ;
#106912=CARTESIAN_POINT ( 'NONE',  ( 0.000000000000000000, -6.134628647623513231, 10.91970695577495931 ) ) ;
#106921=( NAMED_UNIT ( * ) PLANE_ANGLE_UNIT ( ) SI_UNIT ( $, .RADIAN. ) );
#106945=CARTESIAN_POINT ( 'NONE',  ( -6.903494779225470168, -6.732807188596399151, 6.688963559358022337 ) ) ;
#107056=B_SPLINE_CURVE_WITH_KNOTS ( 'NONE', 3,
 ( #30164, #62649, #148192, #147130 ),
 .UNSPECIFIED., .F., .F.,
 ( 4, 4 ),
 ( 0.000000000000000000, 6.033646489354524308E-05 ),
 .UNSPECIFIED. ) ;
#107059=SURFACE_SIDE_STYLE ('',( #186101 ) ) ;
#107072=MECHANICAL_DESIGN_GEOMETRIC_PRESENTATION_REPRESENTATION('',(#2753),#41329);
#107092=CARTESIAN_POINT ( 'NONE',  ( -0.05097232478516647985, -6.890735599540036560, -9.605899910213521409 ) ) ;
#107100=( LENGTH_UNIT ( ) NAMED_UNIT ( * ) SI_UNIT ( .MILLI., .METRE. ) );
#107103=CARTESIAN_POINT ( 'NONE',  ( -6.735605996566196296E-15, -8.407420853759283830, 10.91970695577496286 ) ) ;
#107108=CARTESIAN_POINT ( 'NONE',  ( -0.3617799047494653641, -7.723163706540470130, 10.97113338213672407 ) ) ;
#107143=EDGE_CURVE ( 'NONE', #93709, #209328, #82507, .T. ) ;
#107185=( LENGTH_UNIT ( ) NAMED_UNIT ( * ) SI_UNIT ( .MILLI., .METRE. ) );
#107193=CARTESIAN_POINT ( 'NONE',  ( -6.709229400515914321, -7.621055083280779741, 6.726126798027523002 ) ) ;
#107226=STYLED_ITEM ( 'NONE', ( #199747 ), #159239 ) ;
#107228=CARTESIAN_POINT ( 'NONE',  ( 9.498553103985692303, -9.900000000000005684, -0.1657978611541485181 ) ) ;
#107234=CARTESIAN_POINT ( 'NONE',  ( -11.32145367647657785, 0.9706168436483550988, 3.678563289475746068 ) ) ;
#107244=CARTESIAN_POINT ( 'NONE',  ( -10.96028113393447434, -5.411711732698798905, 0.1309013025973318201 ) ) ;
#107274=CARTESIAN_POINT ( 'NONE',  ( 7.842350841322883959, -5.412329794880678335, -7.657759090810039915 ) ) ;
#107307=ORIENTED_EDGE ( 'NONE', *, *, #198854, .F. ) ;
#107347=CARTESIAN_POINT ( 'NONE',  ( -2.331034670843834533E-15, -9.418601272600245267, -9.907592596884320812 ) ) ;
#107366=LINE ( 'NONE', #157133, #46199 ) ;
#107394=CARTESIAN_POINT ( 'NONE',  ( -8.794101853178666772, 3.696394713403118537, -7.873312689837527856 ) ) ;
#107396=CARTESIAN_POINT ( 'NONE',  ( 7.960263458454529761, -6.452016313277121107, 7.960263458454502228 ) ) ;
#107428=CARTESIAN_POINT ( 'NONE',  ( 0.4356160240586420263, -9.063431457505059186, -9.626717610576610795 ) ) ;
#107434=VERTEX_POINT ( 'NONE', #169059 ) ;
#107439=CARTESIAN_POINT ( 'NONE',  ( -10.93053916617011012, -8.254340240174407484, 0.1907932708458889848 ) ) ;
#107450=LINE ( 'NONE', #173477, #46501 ) ;
#107464=ORIENTED_EDGE ( 'NONE', *, *, #208716, .T. ) ;
#107467=VERTEX_POINT ( 'NONE', #40139 ) ;
#107472=LINE ( 'NONE', #149497, #76947 ) ;
#107493=EDGE_CURVE ( 'NONE', #89199, #180510, #162723, .T. ) ;
#107501=DIRECTION ( 'NONE',  ( 0.000000000000000000, 1.000000000000000000, 0.000000000000000000 ) ) ;
#107503=CARTESIAN_POINT ( 'NONE',  ( -0.03749947599225316591, -9.978860283170366330, -9.579600585153681180 ) ) ;
#107533=ORIENTED_EDGE ( 'NONE', *, *, #120547, .F. ) ;
#107564=CYLINDRICAL_SURFACE ( 'NONE', #205127, 11.99999999999999112 ) ;
#107610=CARTESIAN_POINT ( 'NONE',  ( 6.773846765307987461, -7.473374494058229622, 6.773846765307971474 ) ) ;
#107622=SURFACE_STYLE_FILL_AREA ( #190920 ) ;
#107631=B_SPLINE_CURVE_WITH_KNOTS ( 'NONE', 3,
 ( #139332, #37539, #205361, #168602, #135064, #123169 ),
 .UNSPECIFIED., .F., .F.,
 ( 4, 2, 4 ),
 ( 0.000000000000000000, 0.001226111284895901356, 0.002452222569791802712 ),
 .UNSPECIFIED. ) ;
#107653=EDGE_CURVE ( 'NONE', #80718, #164527, #136386, .T. ) ;
#107660=CARTESIAN_POINT ( 'NONE',  ( 7.698131257602417676, -5.543994141378494334, 7.787098537122152386 ) ) ;
#107662=( NAMED_UNIT ( * ) PLANE_ANGLE_UNIT ( ) SI_UNIT ( $, .RADIAN. ) );
#107724=VERTEX_POINT ( 'NONE', #1887 ) ;
#107728=CARTESIAN_POINT ( 'NONE',  ( -6.773846765317318663, -7.246166700180828535, 6.773846765317342644 ) ) ;
#107741=CARTESIAN_POINT ( 'NONE',  ( 0.05097232478520832832, -6.890735599539905110, 9.605899910213587134 ) ) ;
#107798=CARTESIAN_POINT ( 'NONE',  ( -10.98997987423604528, -6.700000000000002842, 0.4694063952341869794 ) ) ;
#107834=( LENGTH_UNIT ( ) NAMED_UNIT ( * ) SI_UNIT ( .MILLI., .METRE. ) );
#107850=EDGE_CURVE ( 'NONE', #72330, #53448, #64089, .T. ) ;
#107889=CARTESIAN_POINT ( 'NONE',  ( -0.08972248771637633680, -9.919998018256677597, -10.99963958991169477 ) ) ;
#107952=CIRCLE ( 'NONE', #201239, 6.329999999999995630 ) ;
#107958=CARTESIAN_POINT ( 'NONE',  ( 2.269535221382996681, 3.870433085555836428, -11.40607948006776340 ) ) ;
#107968=ORIENTED_EDGE ( 'NONE', *, *, #184338, .F. ) ;
#107978=EDGE_CURVE ( 'NONE', #150870, #165149, #149231, .T. ) ;
#107996=CARTESIAN_POINT ( 'NONE',  ( -3.469446951953614189E-15, 3.507114751586604129, 11.99288524841339054 ) ) ;
#108021=CARTESIAN_POINT ( 'NONE',  ( 0.4350687514514707255, -7.666862915010147717, -10.91132967064556070 ) ) ;
#108052=EDGE_CURVE ( 'NONE', #38980, #29585, #115691, .T. ) ;
#108075=CARTESIAN_POINT ( 'NONE',  ( 7.987977580929924493, -5.530730635397370420, 7.987977580929896071 ) ) ;
#108118=ADVANCED_FACE ( 'NONE', ( #208961 ), #157383, .T. ) ;
#108120=ORIENTED_EDGE ( 'NONE', *, *, #147025, .F. ) ;
#108135=CARTESIAN_POINT ( 'NONE',  ( 10.91805698906627242, -9.914767083041231999, -0.1897524941850662061 ) ) ;
#108138=VECTOR ( 'NONE', #89914, 1000.000000000000000 ) ;
#108140=EDGE_CURVE ( 'NONE', #206526, #27864, #132043, .T. ) ;
#108154=CARTESIAN_POINT ( 'NONE',  ( -6.999862025036992286, -6.532648833121171172, 6.392587740394332307 ) ) ;
#108174=DIRECTION ( 'NONE',  ( 0.000000000000000000, 0.000000000000000000, 1.000000000000000000 ) ) ;
#108224=DIRECTION ( 'NONE',  ( 0.000000000000000000, 0.000000000000000000, 1.000000000000000000 ) ) ;
#108247=CARTESIAN_POINT ( 'NONE',  ( 0.1363799957456746648, -9.242177669965688125, -9.620888806888808986 ) ) ;
#108249=STYLED_ITEM ( 'NONE', ( #122364 ), #79941 ) ;
#108267=CARTESIAN_POINT ( 'NONE',  ( -7.037870247915954280, -8.233137084989836652, 6.381095703207990688 ) ) ;
#108269=VERTEX_POINT ( 'NONE', #153318 ) ;
#108283=CIRCLE ( 'NONE', #21748, 0.08000000000000020983 ) ;
#108286=DIRECTION ( 'NONE',  ( -0.009157509157509154465, 0.000000000000000000, -0.9999580691339163829 ) ) ;
#108301=DIRECTION ( 'NONE',  ( 0.000000000000000000, 1.000000000000000000, 0.000000000000000000 ) ) ;
#108344=CIRCLE ( 'NONE', #59880, 0.07999999999999940492 ) ;
#108378=ORIENTED_EDGE ( 'NONE', *, *, #954, .F. ) ;
#108388=CIRCLE ( 'NONE', #42637, 10.99999999999999112 ) ;
#108408=MECHANICAL_DESIGN_GEOMETRIC_PRESENTATION_REPRESENTATION('',(#21865),#122189);
#108434=DIRECTION ( 'NONE',  ( 0.000000000000000000, -1.000000000000000000, 0.000000000000000000 ) ) ;
#108436=DIRECTION ( 'NONE',  ( 0.000000000000000000, 0.000000000000000000, -1.000000000000000000 ) ) ;
#108464=CARTESIAN_POINT ( 'NONE',  ( -7.257245574617336992, -6.363025497629771543, 6.640718169120116698 ) ) ;
#108499=DIRECTION ( 'NONE',  ( -0.000000000000000000, -1.000000000000000000, -0.000000000000000000 ) ) ;
#108504=CIRCLE ( 'NONE', #46141, 9.479622692290801567 ) ;
#108531=VERTEX_POINT ( 'NONE', #10806 ) ;
#108541=CARTESIAN_POINT ( 'NONE',  ( 10.99866081003787066, -6.614835951978784934, -0.2118258318330271950 ) ) ;
#108562=CIRCLE ( 'NONE', #15084, 0.07999999999999979350 ) ;
#108568=CARTESIAN_POINT ( 'NONE',  ( -7.694877102302403848, -5.389939693150834543, -7.860745937262087146 ) ) ;
#108627=( NAMED_UNIT ( * ) SI_UNIT ( $, .STERADIAN. ) SOLID_ANGLE_UNIT ( ) );
#108668=ADVANCED_FACE ( 'NONE', ( #172015 ), #195130, .T. ) ;
#108675=CARTESIAN_POINT ( 'NONE',  ( 1.347111479062087616E-15, -9.999999999999994671, -10.99999999999999112 ) ) ;
#108718=EDGE_CURVE ( 'NONE', #177991, #67059, #151941, .T. ) ;
#108719=CARTESIAN_POINT ( 'NONE',  ( -0.06712591543029376717, -9.995102890834049347, -10.91960056525075018 ) ) ;
#108766=CIRCLE ( 'NONE', #153693, 0.08000000000000020983 ) ;
#108784=ORIENTED_EDGE ( 'NONE', *, *, #121638, .T. ) ;
#108806=ADVANCED_FACE ( 'NONE', ( #111345 ), #59298, .F. ) ;
#108857=CIRCLE ( 'NONE', #122813, 9.499999999999992895 ) ;
#108866=( LENGTH_UNIT ( ) NAMED_UNIT ( * ) SI_UNIT ( .MILLI., .METRE. ) );
#108869=B_SPLINE_CURVE_WITH_KNOTS ( 'NONE', 3,
 ( #64834, #114725, #111530, #78946, #177536, #96301, #46472 ),
 .UNSPECIFIED., .F., .F.,
 ( 4, 3, 4 ),
 ( 3.315837474970778393E-05, 0.0009000000035470269054, 0.001929259801299067038 ),
 .UNSPECIFIED. ) ;
#108902=FILL_AREA_STYLE ('',( #75266 ) ) ;
#108921=AXIS2_PLACEMENT_3D ( 'NONE', #14226, #112897, #196215 ) ;
#108926=STYLED_ITEM ( 'NONE', ( #205368 ), #156054 ) ;
#108971=CARTESIAN_POINT ( 'NONE',  ( 11.06389876992412091, 3.829536045110819575, -3.713591040152774081 ) ) ;
#108992=TOROIDAL_SURFACE ( 'NONE', #157335, 9.580000000000001847, 0.08000000000000000167 ) ;
#109006=VERTEX_POINT ( 'NONE', #95047 ) ;
#109022=AXIS2_PLACEMENT_3D ( 'NONE', #129062, #148428, #195035 ) ;
#109058=VERTEX_POINT ( 'NONE', #59322 ) ;
#109078=AXIS2_PLACEMENT_3D ( 'NONE', #53050, #134345, #203540 ) ;
#109090=CARTESIAN_POINT ( 'NONE',  ( -7.011678565220742065, -6.606405293530505318, 6.580818069394644532 ) ) ;
#109121=AXIS2_PLACEMENT_3D ( 'NONE', #2238, #197265, #48905 ) ;
#109182=AXIS2_PLACEMENT_3D ( 'NONE', #171362, #22956, #155128 ) ;
#109189=ORIENTED_EDGE ( 'NONE', *, *, #103866, .F. ) ;
#109220=CARTESIAN_POINT ( 'NONE',  ( -6.534012848836717957, -6.583711766989042147, -7.055786748303233935 ) ) ;
#109249=CARTESIAN_POINT ( 'NONE',  ( -9.493819324367761325, -9.279866070759378971, 0.3645580569638187662 ) ) ;
#109271=ORIENTED_EDGE ( 'NONE', *, *, #124727, .F. ) ;
#109273=EDGE_CURVE ( 'NONE', #5447, #201551, #108766, .T. ) ;
#109315=CARTESIAN_POINT ( 'NONE',  ( 11.00023875073173762, -5.574346042903139953, 0.04317804960740431047 ) ) ;
#109318=CIRCLE ( 'NONE', #47123, 0.07999999999999993228 ) ;
#109323=AXIS2_PLACEMENT_3D ( 'NONE', #106268, #9771, #75844 ) ;
#109330=FILL_AREA_STYLE_COLOUR ( '', #60541 ) ;
#109333=CARTESIAN_POINT ( 'NONE',  ( -1.040834085586084257E-14, -7.473374494045017968, -9.579665964948867796 ) ) ;
#109338=CARTESIAN_POINT ( 'NONE',  ( -6.717748655458910534, -7.473374494057226869, 6.717748655460332508 ) ) ;
#109361=DIRECTION ( 'NONE',  ( 0.000000000000000000, 0.000000000000000000, -1.000000000000000000 ) ) ;
#109366=DIRECTION ( 'NONE',  ( 0.000000000000000000, 1.000000000000000000, 0.000000000000000000 ) ) ;
#109387=EDGE_CURVE ( 'NONE', #205391, #98224, #149632, .T. ) ;
#109428=CARTESIAN_POINT ( 'NONE',  ( -0.4382560683119312572, -5.200000000000007283, -10.99126615174919230 ) ) ;
#109429=EDGE_LOOP ( 'NONE', ( #82077, #65670, #92246, #120235, #175802, #8517, #183043, #142472, #199707, #34887, #62591, #152036, #140868, #129329, #174008, #205612, #61652, #727, #5557, #57064, #2907, #48961, #43452, #106383, #87678, #176161, #124131, #62352 ) ) ;
#109440=CARTESIAN_POINT ( 'NONE',  ( -6.775478006741587400, -7.217909409563576517, -6.775478006741549208 ) ) ;
#109479=AXIS2_PLACEMENT_3D ( 'NONE', #71599, #105213, #27130 ) ;
#109507=CARTESIAN_POINT ( 'NONE',  ( 0.000000000000000000, 0.000000000000000000, 0.000000000000000000 ) ) ;
#109539=CARTESIAN_POINT ( 'NONE',  ( -10.76345817711984587, -5.427673425445469491, 0.4370932794886463468 ) ) ;
#109591=LINE ( 'NONE', #126920, #143473 ) ;
#109628=CARTESIAN_POINT ( 'NONE',  ( 0.3870735955438693310, 1.000000000000000888, -11.88799243440807274 ) ) ;
#109647=EDGE_CURVE ( 'NONE', #73672, #160219, #208685, .T. ) ;
#109652=ADVANCED_FACE ( 'NONE', ( #170677 ), #135244, .T. ) ;
#109677=ORIENTED_EDGE ( 'NONE', *, *, #53503, .T. ) ;
#109724=VERTEX_POINT ( 'NONE', #185845 ) ;
#109755=ORIENTED_EDGE ( 'NONE', *, *, #3537, .F. ) ;
#109757=CARTESIAN_POINT ( 'NONE',  ( 0.000000000000000000, 15.50000000000019362, 0.000000000000000000 ) ) ;
#109787=ADVANCED_FACE ( 'NONE', ( #21197 ), #135006, .T. ) ;
#109839=AXIS2_PLACEMENT_3D ( 'NONE', #186274, #85584, #150609 ) ;
#109849=ORIENTED_EDGE ( 'NONE', *, *, #147025, .T. ) ;
#109850=CARTESIAN_POINT ( 'NONE',  ( 10.38614328979769041, 3.507114751586604129, 5.996442624206595795 ) ) ;
#109860=DIRECTION ( 'NONE',  ( 0.000000000000000000, 1.000000000000000000, 0.000000000000000000 ) ) ;
#109861=CARTESIAN_POINT ( 'NONE',  ( 4.593150236022219428E-15, -8.011313137147251240, -11.00000000000000178 ) ) ;
#109931=STYLED_ITEM ( 'NONE', ( #165783 ), #202122 ) ;
#109937=CARTESIAN_POINT ( 'NONE',  ( -2.019980081995991661, 3.974415841077574285, 11.36314192354172192 ) ) ;
#109989=CARTESIAN_POINT ( 'NONE',  ( -0.08814328694728679192, -9.915773547069447247, -10.99964701288570623 ) ) ;
#110020=CARTESIAN_POINT ( 'NONE',  ( -0.1007326007326104361, -9.919999999999998153, -10.99953876047306167 ) ) ;
#110057=LINE ( 'NONE', #96969, #72360 ) ;
#110073=ORIENTED_EDGE ( 'NONE', *, *, #187963, .F. ) ;
#110082=CARTESIAN_POINT ( 'NONE',  ( -10.23203630735456393, -6.594478602028840619, 1.760317133499380763E-15 ) ) ;
#110092=DIRECTION ( 'NONE',  ( 0.000000000000000000, 0.000000000000000000, 1.000000000000000000 ) ) ;
#110123=CARTESIAN_POINT ( 'NONE',  ( 9.620326184871647257, -9.190313392136383541, -0.3418113563954068290 ) ) ;
#110128=AXIS2_PLACEMENT_3D ( 'NONE', #153987, #5555, #172374 ) ;
#110139=CARTESIAN_POINT ( 'NONE',  ( -2.331034670843834533E-15, -6.465328379374287948, 10.58872653680447407 ) ) ;
#110154=FACE_OUTER_BOUND ( 'NONE', #105331, .T. ) ;
#110243=CIRCLE ( 'NONE', #203514, 0.07999999999999907185 ) ;
#110287=ADVANCED_FACE ( 'NONE', ( #129237 ), #163062, .T. ) ;
#110307=CARTESIAN_POINT ( 'NONE',  ( -9.590670562336521598, -9.593477663480378226, 0.1674057773689523465 ) ) ;
#110319=AXIS2_PLACEMENT_3D ( 'NONE', #6798, #154151, #106512 ) ;
#110324=B_SPLINE_CURVE_WITH_KNOTS ( 'NONE', 3,
 ( #166582, #51777, #117894, #124325, #10466, #159935, #141596, #190285, #125380, #77609, #76540, #191346, #9414, #139434, #59222, #44068 ),
 .UNSPECIFIED., .F., .F.,
 ( 4, 3, 3, 3, 3, 4 ),
 ( 0.000000000000000000, 2.209015272824978271E-05, 5.594181769345698359E-05, 8.979300607464787737E-05, 0.0001236442050441801050, 0.0001574956163004470730 ),
 .UNSPECIFIED. ) ;
#110329=ADVANCED_FACE ( 'NONE', ( #178972 ), #180028, .F. ) ;
#110343=EDGE_CURVE ( 'NONE', #58157, #192481, #97726, .T. ) ;
#110376=CARTESIAN_POINT ( 'NONE',  ( 8.064677165291193717, -5.223431457505076203, -7.446209719563348983 ) ) ;
#110379=CARTESIAN_POINT ( 'NONE',  ( -0.3870735955438814879, 1.000000000000000888, 11.88799243440809050 ) ) ;
#110390=FACE_BOUND ( 'NONE', #74488, .T. ) ;
#110438=VERTEX_POINT ( 'NONE', #76377 ) ;
#110478=( LENGTH_UNIT ( ) NAMED_UNIT ( * ) SI_UNIT ( .MILLI., .METRE. ) );
#110490=CARTESIAN_POINT ( 'NONE',  ( -0.1368885365587547698, -5.294776013890321487, -10.99935770452674610 ) ) ;
#110516=CARTESIAN_POINT ( 'NONE',  ( 0.1980946632348811465, -8.057097448493964365, 9.531438498077058341 ) ) ;
#110555=EDGE_CURVE ( 'NONE', #55041, #57699, #164835, .T. ) ;
#110566=DIRECTION ( 'NONE',  ( 0.000000000000000000, -1.000000000000000000, 0.000000000000000000 ) ) ;
#110607=DIRECTION ( 'NONE',  ( -0.04529798058948708572, 0.000000000000000000, -0.9989735196462988798 ) ) ;
#110609=EDGE_CURVE ( 'NONE', #50012, #94238, #28020, .T. ) ;
#110629=CARTESIAN_POINT ( 'NONE',  ( 7.712222144929244294, -6.293595771080967793, 7.712222144929218537 ) ) ;
#110630=CARTESIAN_POINT ( 'NONE',  ( 6.709229400517491726, -7.621055083280683817, -6.726126798030838572 ) ) ;
#110641=FILL_AREA_STYLE_COLOUR ( '', #90314 ) ;
#110643=AXIS2_PLACEMENT_3D ( 'NONE', #146823, #177165, #77521 ) ;
#110650=DIRECTION ( 'NONE',  ( 1.993562223070362833E-14, -1.000000000000000000, 2.190074022720978955E-12 ) ) ;
#110743=EDGE_CURVE ( 'NONE', #74942, #159480, #100890, .T. ) ;
#110808=ADVANCED_FACE ( 'NONE', ( #3370 ), #185161, .T. ) ;
#110815=CARTESIAN_POINT ( 'NONE',  ( 6.484567079770447329, -6.583980363594976737, 7.100579091573052004 ) ) ;
#110819=CARTESIAN_POINT ( 'NONE',  ( 6.650326532587140349, -8.038658175288279750, 6.784185045882107801 ) ) ;
#110825=( NAMED_UNIT ( * ) PLANE_ANGLE_UNIT ( ) SI_UNIT ( $, .RADIAN. ) );
#110828=B_SPLINE_CURVE_WITH_KNOTS ( 'NONE', 3,
 ( #118016, #104921, #85445, #201303, #134234, #151530, #52943, #204505, #119080, #185061 ),
 .UNSPECIFIED., .F., .F.,
 ( 4, 2, 2, 2, 4 ),
 ( 0.000000000000000000, 0.0002021113321160290582, 0.0004042226642320581164, 0.0006063339963480871746, 0.0008084453284641167749 ),
 .UNSPECIFIED. ) ;
#110845=FACE_OUTER_BOUND ( 'NONE', #162283, .T. ) ;
#110858=EDGE_CURVE ( 'NONE', #96195, #94484, #54288, .T. ) ;
#110859=CARTESIAN_POINT ( 'NONE',  ( 9.899039292889495911, 2.972657967447090321, 6.161878781005994732 ) ) ;
#110878=CARTESIAN_POINT ( 'NONE',  ( -6.773376348128482327, -7.215568602681039501, -6.661184042391679050 ) ) ;
#110882=ORIENTED_EDGE ( 'NONE', *, *, #117706, .F. ) ;
#110919=B_SPLINE_CURVE_WITH_KNOTS ( 'NONE', 3,
 ( #206949, #109539, #205883, #27132, #93239, #159271, #213329 ),
 .UNSPECIFIED., .F., .F.,
 ( 4, 3, 4 ),
 ( 3.314949680324100580E-05, 0.0009000000012044581665, 0.001958074173707502127 ),
 .UNSPECIFIED. ) ;
#110921=DIRECTION ( 'NONE',  ( 0.000000000000000000, 0.000000000000000000, 1.000000000000000000 ) ) ;
#110968=EDGE_CURVE ( 'NONE', #71109, #73672, #97846, .T. ) ;
#110989=ADVANCED_FACE ( 'NONE', ( #42319 ), #49439, .T. ) ;
#111083=DIRECTION ( 'NONE',  ( 0.000000000000000000, 0.000000000000000000, 1.000000000000000000 ) ) ;
#111122=DIRECTION ( 'NONE',  ( 0.000000000000000000, 0.000000000000000000, 1.000000000000000000 ) ) ;
#111182=LINE ( 'NONE', #41872, #68115 ) ;
#111188=CARTESIAN_POINT ( 'NONE',  ( 0.008173644115962452189, -6.287979527546275094, 10.90726532705803820 ) ) ;
#111207=DIRECTION ( 'NONE',  ( 0.000000000000000000, 1.000000000000000000, 0.000000000000000000 ) ) ;
#111224=SURFACE_STYLE_FILL_AREA ( #99172 ) ;
#111306=CARTESIAN_POINT ( 'NONE',  ( -0.4359507092143430351, -8.863025497813993070, 9.827344407697081508 ) ) ;
#111339=CARTESIAN_POINT ( 'NONE',  ( -10.25773349932952527, -6.796015482748905434, -2.597247770456278818E-17 ) ) ;
#111345=FACE_OUTER_BOUND ( 'NONE', #159573, .T. ) ;
#111346=VERTEX_POINT ( 'NONE', #11778 ) ;
#111356=MECHANICAL_DESIGN_GEOMETRIC_PRESENTATION_REPRESENTATION('',(#31820),#194305);
#111366=EDGE_CURVE ( 'NONE', #17507, #54631, #58702, .T. ) ;
#111402=( NAMED_UNIT ( * ) SI_UNIT ( $, .STERADIAN. ) SOLID_ANGLE_UNIT ( ) );
#111425=CARTESIAN_POINT ( 'NONE',  ( 7.720982897393571243, -6.134628647623485698, -7.834948825496923952 ) ) ;
#111433=CIRCLE ( 'NONE', #42127, 11.99999999999999112 ) ;
#111460=( BOUNDED_SURFACE ( )  B_SPLINE_SURFACE ( 3, 2, ( 
 ( #4774, #70852, #136966 ),
 ( #24245, #122938, #90346 ),
 ( #39450, #139102, #140186 ),
 ( #188895, #206207, #91430 ),
 ( #57835, #10143, #126123 ),
 ( #173753, #174819, #23175 ),
 ( #205129, #207280, #142327 ),
 ( #27466, #89289, #171580 ) ),
 .UNSPECIFIED., .F., .F., .T. ) 
 B_SPLINE_SURFACE_WITH_KNOTS ( ( 4, 2, 2, 4 ),
 ( 3, 3 ),
 ( 0.000000000000000000, 0.0004924884914732709533, 0.0007387327372099063757, 0.0009849769829465419065 ),
 ( 0.000000000000000000, 1.000000000000000000 ),
 .UNSPECIFIED. ) 
 GEOMETRIC_REPRESENTATION_ITEM ( )  RATIONAL_B_SPLINE_SURFACE ( (
 ( 1.000000000000000000, 0.7045118851637552915, 1.000000000000000000),
 ( 1.000000000000000000, 0.7593505504065475309, 1.000000000000000000),
 ( 1.000000000000000000, 0.8104906253031783914, 1.000000000000000000),
 ( 1.000000000000000000, 0.8722646935501797705, 1.000000000000000000),
 ( 1.000000000000000000, 0.8905178607894786991, 1.000000000000000000),
 ( 1.000000000000000000, 0.9170530604353607229, 1.000000000000000000),
 ( 1.000000000000000000, 0.9248184710077410609, 1.000000000000000000),
 ( 1.000000000000000000, 0.9238795325112870716, 1.000000000000000000) ) ) 
 REPRESENTATION_ITEM ( '' )  SURFACE ( )  );
#111530=CARTESIAN_POINT ( 'NONE',  ( 0.4648879685169841069, -7.768188185258929401, 9.920930332858635126 ) ) ;
#111563=FACE_OUTER_BOUND ( 'NONE', #205884, .T. ) ;
#111566=CARTESIAN_POINT ( 'NONE',  ( -1.338312056661794536E-15, 3.975933801733731787, 11.54759062144379023 ) ) ;
#111576=DIRECTION ( 'NONE',  ( 0.000000000000000000, -1.000000000000000000, 0.000000000000000000 ) ) ;
#111598=AXIS2_PLACEMENT_3D ( 'NONE', #34827, #100901, #18581 ) ;
#111631=EDGE_CURVE ( 'NONE', #157630, #50845, #57348, .T. ) ;
#111641=CARTESIAN_POINT ( 'NONE',  ( -6.643335646896348479, -7.986884274785886362, -6.845108005540228469 ) ) ;
#111661=COLOUR_RGB ( '', 0.72549020, 0.75294118, 0.79215686) ;
#111693=CARTESIAN_POINT ( 'NONE',  ( 7.834948825496932834, -6.134628647623485698, 7.720982897393583677 ) ) ;
#111697=CARTESIAN_POINT ( 'NONE',  ( 0.000000000000000000, -5.223431457505076203, 0.000000000000000000 ) ) ;
#111707=( LENGTH_UNIT ( ) NAMED_UNIT ( * ) SI_UNIT ( .MILLI., .METRE. ) );
#111732=B_SPLINE_CURVE_WITH_KNOTS ( 'NONE', 3,
 ( #201834, #119617, #189880, #20950, #39368, #37232, #53479, #106554 ),
 .UNSPECIFIED., .F., .F.,
 ( 4, 2, 2, 4 ),
 ( 6.586514544919025777E-16, 0.0002305131806121977036, 0.0004610263612237367544, 0.0009220527224468139885 ),
 .UNSPECIFIED. ) ;
#111763=ORIENTED_EDGE ( 'NONE', *, *, #156034, .T. ) ;
#111766=ORIENTED_EDGE ( 'NONE', *, *, #150154, .F. ) ;
#111769=CARTESIAN_POINT ( 'NONE',  ( -7.446209719563363194, -5.223431457505083308, -8.064677165291197269 ) ) ;
#111775=ORIENTED_EDGE ( 'NONE', *, *, #22536, .F. ) ;
#111835=CIRCLE ( 'NONE', #132516, 0.08000000000000020983 ) ;
#111842=ORIENTED_EDGE ( 'NONE', *, *, #103265, .T. ) ;
#111855=ORIENTED_EDGE ( 'NONE', *, *, #187677, .F. ) ;
#111898=CARTESIAN_POINT ( 'NONE',  ( 6.773376349081638104, -7.645986912801321367, 6.661184041422480107 ) ) ;
#111905=( BOUNDED_SURFACE ( )  B_SPLINE_SURFACE ( 3, 2, ( 
 ( #179719, #213251, #132067 ),
 ( #17182, #31336, #163468 ),
 ( #65920, #97413, #15048 ),
 ( #115834, #81141, #198078 ) ),
 .UNSPECIFIED., .F., .F., .F. ) 
 B_SPLINE_SURFACE_WITH_KNOTS ( ( 4, 4 ),
 ( 3, 3 ),
 ( 0.06089817005132014405, 0.06334004685008763624 ),
 ( 0.000000000000000000, 1.000000000000000000 ),
 .UNSPECIFIED. ) 
 GEOMETRIC_REPRESENTATION_ITEM ( )  RATIONAL_B_SPLINE_SURFACE ( (
 ( 1.000000000000000000, 0.7169883299104516938, 1.000000000000000000),
 ( 1.000000000000000000, 0.7174882367719587206, 1.000000000000000000),
 ( 1.000000000000000000, 0.7180609655865445307, 1.000000000000000000),
 ( 1.000000000000000000, 0.7187540731123146509, 1.000000000000000000) ) ) 
 REPRESENTATION_ITEM ( '' )  SURFACE ( )  );
#111928=CARTESIAN_POINT ( 'NONE',  ( 7.777967379493318845, -5.907420853759296264, 7.664830294503448549 ) ) ;
#111930=EDGE_LOOP ( 'NONE', ( #23712, #205121, #103905, #134462 ) ) ;
#111938=EDGE_CURVE ( 'NONE', #113870, #123257, #76707, .T. ) ;
#111958=( BOUNDED_SURFACE ( )  B_SPLINE_SURFACE ( 3, 2, ( 
 ( #201359, #168883, #104976 ),
 ( #171017, #154781, #20487 ),
 ( #204559, #3155, #56207 ),
 ( #136408, #69226, #35678 ) ),
 .UNSPECIFIED., .F., .F., .T. ) 
 B_SPLINE_SURFACE_WITH_KNOTS ( ( 4, 4 ),
 ( 3, 3 ),
 ( 0.000000000000000000, 3.124390133962058787E-05 ),
 ( 0.000000000000000000, 1.000000000000000000 ),
 .UNSPECIFIED. ) 
 GEOMETRIC_REPRESENTATION_ITEM ( )  RATIONAL_B_SPLINE_SURFACE ( (
 ( 1.000000000000000000, 0.7100530722023771224, 1.000000000000000000),
 ( 1.000000000000000000, 0.7100778649077736926, 1.000000000000000000),
 ( 1.000000000000000000, 0.7091082185075937572, 1.000000000000000000),
 ( 1.000000000000000000, 0.7071067811862440378, 1.000000000000000000) ) ) 
 REPRESENTATION_ITEM ( '' )  SURFACE ( )  );
#111960=ORIENTED_EDGE ( 'NONE', *, *, #12966, .T. ) ;
#112039=ADVANCED_BREP_SHAPE_REPRESENTATION ( '', ( #156054, #200407 ), #83064 ) ;
#112143=( BOUNDED_SURFACE ( )  B_SPLINE_SURFACE ( 3, 2, ( 
 ( #164178, #85038, #200892 ),
 ( #34154, #551, #18954 ),
 ( #66616, #86110, #50416 ),
 ( #132763, #116535, #197718 ),
 ( #82904, #100224, #20021 ),
 ( #81848, #166292, #3751 ),
 ( #115479, #17881, #83966 ),
 ( #98127, #152181, #147931 ) ),
 .UNSPECIFIED., .F., .F., .T. ) 
 B_SPLINE_SURFACE_WITH_KNOTS ( ( 4, 2, 2, 4 ),
 ( 3, 3 ),
 ( 0.000000000000000000, 0.0002475938981900030044, 0.0004951877963800060088, 0.0009903755927600120176 ),
 ( 0.000000000000000000, 1.000000000000000000 ),
 .UNSPECIFIED. ) 
 GEOMETRIC_REPRESENTATION_ITEM ( )  RATIONAL_B_SPLINE_SURFACE ( (
 ( 1.000000000000000000, 0.9238795325112901802, 1.000000000000000000),
 ( 1.000000000000000000, 0.9248499699755211578, 1.000000000000000000),
 ( 1.000000000000000000, 0.9171047238581211403, 1.000000000000000000),
 ( 1.000000000000000000, 0.8907236462371712626, 1.000000000000000000),
 ( 1.000000000000000000, 0.8725411758595091882, 1.000000000000000000),
 ( 1.000000000000000000, 0.8105159241142133597, 1.000000000000000000),
 ( 1.000000000000000000, 0.7599483315140991291, 1.000000000000000000),
 ( 1.000000000000000000, 0.7045118851637763857, 1.000000000000000000) ) ) 
 REPRESENTATION_ITEM ( '' )  SURFACE ( )  );
#112238=CARTESIAN_POINT ( 'NONE',  ( -2.057629584373543707, 2.441452740530747789, 11.54123292161952641 ) ) ;
#112256=CARTESIAN_POINT ( 'NONE',  ( 0.4635785636673654952, -6.836568542495036205, 10.85353573482952250 ) ) ;
#112265=CIRCLE ( 'NONE', #195236, 0.07999999999999951594 ) ;
#112325=CARTESIAN_POINT ( 'NONE',  ( -7.137427454244817504, -7.616807780282264240, -7.137427454241226599 ) ) ;
#112370=( NAMED_UNIT ( * ) PLANE_ANGLE_UNIT ( ) SI_UNIT ( $, .RADIAN. ) );
#112394=ORIENTED_EDGE ( 'NONE', *, *, #167891, .F. ) ;
#112408=FILL_AREA_STYLE_COLOUR ( '', #30948 ) ;
#112474=( LENGTH_UNIT ( ) NAMED_UNIT ( * ) SI_UNIT ( .MILLI., .METRE. ) );
#112496=CARTESIAN_POINT ( 'NONE',  ( 9.554207839743581232, -7.792803924024971352, -0.03436587256738153628 ) ) ;
#112499=FILL_AREA_STYLE_COLOUR ( '', #16457 ) ;
#112514=DIRECTION ( 'NONE',  ( 0.000000000000000000, -1.000000000000000000, 0.000000000000000000 ) ) ;
#112543=CARTESIAN_POINT ( 'NONE',  ( 10.91970695577495754, -9.999999999999994671, 0.08000000000000194456 ) ) ;
#112620=CARTESIAN_POINT ( 'NONE',  ( 0.000000000000000000, 1.000000000000000888, 0.000000000000000000 ) ) ;
#112632=CARTESIAN_POINT ( 'NONE',  ( -0.3199376857465079937, -8.148349307653480977, -9.520891725236014125 ) ) ;
#112633=CARTESIAN_POINT ( 'NONE',  ( -6.773846765317340868, -7.246166700180801001, -6.773846765317301788 ) ) ;
#112645=CARTESIAN_POINT ( 'NONE',  ( 0.000000000000000000, 0.000000000000000000, 0.000000000000000000 ) ) ;
#112646=ORIENTED_EDGE ( 'NONE', *, *, #130897, .F. ) ;
#112725=COLOUR_RGB ( '', 0.08235294, 0.09019608, 0.10196078) ;
#112760=CARTESIAN_POINT ( 'NONE',  ( 6.661184041420942670, -7.473374494058216300, -6.773376349083130243 ) ) ;
#112782=AXIS2_PLACEMENT_3D ( 'NONE', #83417, #19474, #201412 ) ;
#112796=ORIENTED_EDGE ( 'NONE', *, *, #102912, .T. ) ;
#112838=CARTESIAN_POINT ( 'NONE',  ( -7.642790800258748294E-15, -9.595263517168229228, 9.591985693221618092 ) ) ;
#112840=DIRECTION ( 'NONE',  ( -0.000000000000000000, -0.000000000000000000, -1.000000000000000000 ) ) ;
#112857=CARTESIAN_POINT ( 'NONE',  ( -9.495347311156809411, -6.857257212219918685, 3.422217897015904270E-15 ) ) ;
#112881=AXIS2_PLACEMENT_3D ( 'NONE', #210810, #62435, #46210 ) ;
#112897=DIRECTION ( 'NONE',  ( -0.000000000000000000, -1.000000000000000000, -0.000000000000000000 ) ) ;
#112973=CARTESIAN_POINT ( 'NONE',  ( -10.98194350564911659, -7.666862915010147717, 0.6300133639306291222 ) ) ;
#113056=VERTEX_POINT ( 'NONE', #208367 ) ;
#113062=ORIENTED_EDGE ( 'NONE', *, *, #102667, .F. ) ;
#113075=DIRECTION ( 'NONE',  ( 0.000000000000000000, 1.000000000000000000, 0.000000000000000000 ) ) ;
#113085=CARTESIAN_POINT ( 'NONE',  ( 7.687279255399376694E-16, -0.02379966007286238305, 6.277139874739035896 ) ) ;
#113153=( BOUNDED_SURFACE ( )  B_SPLINE_SURFACE ( 3, 2, ( 
 ( #64047, #97633, #178881 ),
 ( #44619, #81359, #144287 ),
 ( #177809, #65087, #160482 ),
 ( #30493, #61920, #96577 ),
 ( #164738, #130192, #14200 ),
 ( #69, #12089, #98682 ),
 ( #196185, #79229, #162624 ),
 ( #80293, #147439, #146391 ) ),
 .UNSPECIFIED., .F., .F., .T. ) 
 B_SPLINE_SURFACE_WITH_KNOTS ( ( 4, 2, 2, 4 ),
 ( 3, 3 ),
 ( -6.505213034913026604E-19, 0.0002575597274893380085, 0.0005151194549786766675, 0.001030238909957353986 ),
 ( 0.000000000000000000, 1.000000000000000000 ),
 .UNSPECIFIED. ) 
 GEOMETRIC_REPRESENTATION_ITEM ( )  RATIONAL_B_SPLINE_SURFACE ( (
 ( 1.000000000000000000, 0.9238795325112806323, 1.000000000000000000),
 ( 1.000000000000000000, 0.9228594682463592269, 1.000000000000000000),
 ( 1.000000000000000000, 0.9150875845227820493, 1.000000000000000000),
 ( 1.000000000000000000, 0.8905471774192091905, 1.000000000000000000),
 ( 1.000000000000000000, 0.8740340839248708082, 1.000000000000000000),
 ( 1.000000000000000000, 0.8160099319845808274, 1.000000000000000000),
 ( 1.000000000000000000, 0.7673743911479409263, 1.000000000000000000),
 ( 1.000000000000000000, 0.7100530722070714784, 1.000000000000000000) ) ) 
 REPRESENTATION_ITEM ( '' )  SURFACE ( )  );
#113158=AXIS2_PLACEMENT_3D ( 'NONE', #71635, #72716, #6637 ) ;
#113192=( GEOMETRIC_REPRESENTATION_CONTEXT ( 3 ) GLOBAL_UNCERTAINTY_ASSIGNED_CONTEXT ( ( #204428 ) ) GLOBAL_UNIT_ASSIGNED_CONTEXT ( ( #33353, #195864, #31239 ) ) REPRESENTATION_CONTEXT ( 'NONE', 'WORKASPACE' ) );
#113228=EDGE_CURVE ( 'NONE', #73672, #144836, #143899, .T. ) ;
#113243=CARTESIAN_POINT ( 'NONE',  ( 10.87634538855762401, 3.956598013261174884, -3.867819554622535350 ) ) ;
#113279=VERTEX_POINT ( 'NONE', #174846 ) ;
#113325=CARTESIAN_POINT ( 'NONE',  ( -8.917737905728749581, 3.447199233515649386, -8.029567276306266876 ) ) ;
#113340=CIRCLE ( 'NONE', #206784, 6.449999999999992184 ) ;
#113360=CARTESIAN_POINT ( 'NONE',  ( -9.796090618744084821, 3.974415841077576950, -6.102288299938490646 ) ) ;
#113395=CARTESIAN_POINT ( 'NONE',  ( -7.728718841140393536, -6.124285369217662200, -7.728718841140358897 ) ) ;
#113421=CARTESIAN_POINT ( 'NONE',  ( 0.07999999999999327094, -9.999999999999994671, 10.91970695577496286 ) ) ;
#113439=CARTESIAN_POINT ( 'NONE',  ( -1.192622389734054877E-15, -8.605993949662202880, 10.72098668450195369 ) ) ;
#113450=CARTESIAN_POINT ( 'NONE',  ( 8.064677165291197269, -5.223431457505083308, -7.446209719563361418 ) ) ;
#113469=CARTESIAN_POINT ( 'NONE',  ( 0.000000000000000000, 1.000000000000000888, 0.000000000000000000 ) ) ;
#113474=CARTESIAN_POINT ( 'NONE',  ( -9.695354081530210166, -7.357813805514500594, 1.138412281109779656E-15 ) ) ;
#113478=CARTESIAN_POINT ( 'NONE',  ( 9.093502852636627054, 1.000000000000000888, 7.666967846417570343 ) ) ;
#113509=CARTESIAN_POINT ( 'NONE',  ( 7.721398836998350390, -5.907420853759296264, -7.721398836998385917 ) ) ;
#113524=CIRCLE ( 'NONE', #172373, 11.89429233241351902 ) ;
#113534=DIRECTION ( 'NONE',  ( 0.000000000000000000, -1.000000000000000000, 0.000000000000000000 ) ) ;
#113569=CARTESIAN_POINT ( 'NONE',  ( 9.579665964948885559, -7.473374494045003757, -1.531435568635775013E-15 ) ) ;
#113576=CARTESIAN_POINT ( 'NONE',  ( 10.99681319029664728, -5.196788179137230124, -0.2733121965684300325 ) ) ;
#113595=EDGE_LOOP ( 'NONE', ( #143671, #168774 ) ) ;
#113616=ADVANCED_FACE ( 'NONE', ( #96801 ), #48051, .F. ) ;
#113625=CARTESIAN_POINT ( 'NONE',  ( 9.512045263456263555, -8.176568542494905500, -0.4655551865852067817 ) ) ;
#113630=MECHANICAL_DESIGN_GEOMETRIC_PRESENTATION_REPRESENTATION('',(#137711),#103068);
#113631=CIRCLE ( 'NONE', #188542, 0.08000000000000020983 ) ;
#113687=EDGE_CURVE ( 'NONE', #40132, #201589, #4702, .T. ) ;
#113711=CARTESIAN_POINT ( 'NONE',  ( -10.38614328979761403, 3.507114751586604129, 5.996442624206741456 ) ) ;
#113758=EDGE_CURVE ( 'NONE', #139509, #74995, #105103, .T. ) ;
#113794=CARTESIAN_POINT ( 'NONE',  ( 6.999862025036645008, -6.532648833121171172, -6.392587740394702678 ) ) ;
#113806=ORIENTED_EDGE ( 'NONE', *, *, #210461, .F. ) ;
#113828=CARTESIAN_POINT ( 'NONE',  ( -7.667935170093251429, -6.766388843766943495, -7.887197531381546334 ) ) ;
#113849=CIRCLE ( 'NONE', #131152, 11.99999999999999112 ) ;
#113870=VERTEX_POINT ( 'NONE', #15494 ) ;
#113879=CARTESIAN_POINT ( 'NONE',  ( 9.093502852636627054, 1.000000000000000888, 7.666967846417570343 ) ) ;
#113886=CARTESIAN_POINT ( 'NONE',  ( 10.85353573482940526, -6.836568542494932288, -0.4635785636673656063 ) ) ;
#113910=CARTESIAN_POINT ( 'NONE',  ( -0.4635785636673758758, -6.836568542495036205, -10.85353573482950829 ) ) ;
#113912=ORIENTED_EDGE ( 'NONE', *, *, #20338, .T. ) ;
#113939=CARTESIAN_POINT ( 'NONE',  ( -9.578206935422358015, -9.907361015872668375, 0.1671882239541429838 ) ) ;
#113976=VERTEX_POINT ( 'NONE', #51221 ) ;
#114037=CARTESIAN_POINT ( 'NONE',  ( -7.047919420689663816, -8.186910006423165242, 6.389500220311202128 ) ) ;
#114039=AXIS2_PLACEMENT_3D ( 'NONE', #181584, #96114, #196786 ) ;
#114053=CARTESIAN_POINT ( 'NONE',  ( -9.499606442108964544, -9.900000000000005684, 0.08647222121513538362 ) ) ;
#114066=CARTESIAN_POINT ( 'NONE',  ( 0.000000000000000000, 7.849261790823902629, 0.000000000000000000 ) ) ;
#114068=VERTEX_POINT ( 'NONE', #186540 ) ;
#114095=CARTESIAN_POINT ( 'NONE',  ( -6.710127771514629025, -7.162053774861991684, -6.725445687907746439 ) ) ;
#114100=VERTEX_POINT ( 'NONE', #171360 ) ;
#114111=CYLINDRICAL_SURFACE ( 'NONE', #76587, 10.99999999999999112 ) ;
#114129=ORIENTED_EDGE ( 'NONE', *, *, #154365, .F. ) ;
#114140=CARTESIAN_POINT ( 'NONE',  ( 0.08228926980217896037, -9.910743320677063650, 9.499643698783458490 ) ) ;
#114174=CARTESIAN_POINT ( 'NONE',  ( -7.721398836998398352, -5.907420853759296264, -7.721398836998357496 ) ) ;
#114229=EDGE_LOOP ( 'NONE', ( #21617, #143982, #133460, #112646, #8403 ) ) ;
#114328=DIRECTION ( 'NONE',  ( 0.6123724356957896964, 0.7071067811865539010, 0.3535533905932691789 ) ) ;
#114330=EDGE_CURVE ( 'NONE', #58795, #144319, #22193, .T. ) ;
#114344=ORIENTED_EDGE ( 'NONE', *, *, #37148, .F. ) ;
#114356=CARTESIAN_POINT ( 'NONE',  ( 9.606148981167590861, -6.583980363595129504, -0.4355862708379804604 ) ) ;
#114367=DIRECTION ( 'NONE',  ( -0.04888523518676873847, 0.000000000000000000, -0.9988044021632734859 ) ) ;
#114370=CARTESIAN_POINT ( 'NONE',  ( -2.039928227386959669, 3.162178953954597471, 11.45750328113832062 ) ) ;
#114412=ORIENTED_EDGE ( 'NONE', *, *, #199113, .T. ) ;
#114435=CARTESIAN_POINT ( 'NONE',  ( 6.661184041420942670, -7.246166700180828535, -6.773376349083129355 ) ) ;
#114443=CARTESIAN_POINT ( 'NONE',  ( -0.4373225248172993851, -5.223431457505089526, -10.96785329849811497 ) ) ;
#114503=FACE_OUTER_BOUND ( 'NONE', #67363, .T. ) ;
#114510=EDGE_CURVE ( 'NONE', #107434, #144331, #125904, .T. ) ;
#114513=CARTESIAN_POINT ( 'NONE',  ( 10.91804383151479740, -8.407420853759283830, -0.1905751639681655396 ) ) ;
#114541=( NAMED_UNIT ( * ) PLANE_ANGLE_UNIT ( ) SI_UNIT ( $, .RADIAN. ) );
#114598=DIRECTION ( 'NONE',  ( 0.000000000000000000, 0.000000000000000000, -1.000000000000000000 ) ) ;
#114648=CARTESIAN_POINT ( 'NONE',  ( 6.716119544743627934, -7.217450603038206403, 6.719405205104847845 ) ) ;
#114653=DIRECTION ( 'NONE',  ( 0.0006885664517736132502, 0.9962285034897219171, -0.08676574618402704830 ) ) ;
#114679=CYLINDRICAL_SURFACE ( 'NONE', #158118, 11.99999999999999112 ) ;
#114725=CARTESIAN_POINT ( 'NONE',  ( 0.4652101495396396280, -7.972382850425330680, 9.716492259128738596 ) ) ;
#114731=VERTEX_POINT ( 'NONE', #212373 ) ;
#114768=CARTESIAN_POINT ( 'NONE',  ( -8.043940816608023070, -6.893137084989708008, 7.503508839934920793 ) ) ;
#114772=ORIENTED_EDGE ( 'NONE', *, *, #106908, .T. ) ;
#114775=CARTESIAN_POINT ( 'NONE',  ( 0.3846410972798547934, -8.199730735666078019, 9.492545994384032682 ) ) ;
#114781=COLOUR_RGB ( '', 0.72549020, 0.75294118, 0.79215686) ;
#114840=VERTEX_POINT ( 'NONE', #201192 ) ;
#114847=FILL_AREA_STYLE_COLOUR ( '', #197695 ) ;
#114856=ORIENTED_EDGE ( 'NONE', *, *, #165594, .F. ) ;
#114880=CARTESIAN_POINT ( 'NONE',  ( -2.632154883592737318E-16, -9.671843677217918156, 9.585733692702627096 ) ) ;
#114901=STYLED_ITEM ( 'NONE', ( #136384 ), #75064 ) ;
#114958=CARTESIAN_POINT ( 'NONE',  ( -6.735605996566196296E-15, -9.746166700180788567, 9.579665964948873125 ) ) ;
#115043=CARTESIAN_POINT ( 'NONE',  ( 9.946057155611644163, 2.515145635913765609, 6.189092007093160319 ) ) ;
#115084=CARTESIAN_POINT ( 'NONE',  ( 9.499606441938663437, -9.580980486002390606, -0.08647223992350253075 ) ) ;
#115086=CARTESIAN_POINT ( 'NONE',  ( 6.506745451169511085, -8.202869699938540649, 6.922231005658569636 ) ) ;
#115087=CARTESIAN_POINT ( 'NONE',  ( -6.493979435825336211, -7.868711954889216820, 6.493979435825359303 ) ) ;
#115094=( BOUNDED_SURFACE ( )  B_SPLINE_SURFACE ( 3, 2, ( 
 ( #132914, #18041, #164319 ),
 ( #36439, #181616, #84128 ),
 ( #102514, #100379, #214085 ),
 ( #150214, #151277, #86264 ),
 ( #33245, #168576, #135038 ),
 ( #51645, #99327, #2849 ),
 ( #201051, #20177, #117769 ),
 ( #16971, #68918, #149127 ) ),
 .UNSPECIFIED., .F., .F., .T. ) 
 B_SPLINE_SURFACE_WITH_KNOTS ( ( 4, 2, 2, 4 ),
 ( 3, 3 ),
 ( 1.016439536705160407E-16, 0.0002568729646054561692, 0.0005137459292108107487, 0.001027491858421519799 ),
 ( 0.000000000000000000, 1.000000000000000000 ),
 .UNSPECIFIED. ) 
 GEOMETRIC_REPRESENTATION_ITEM ( )  RATIONAL_B_SPLINE_SURFACE ( (
 ( 1.000000000000000000, 0.3826834323651128189, 1.000000000000000000),
 ( 1.000000000000000000, 0.3847114443836955888, 1.000000000000000000),
 ( 1.000000000000000000, 0.4039255759072543084, 1.000000000000000000),
 ( 1.000000000000000000, 0.4557194474498772463, 1.000000000000000000),
 ( 1.000000000000000000, 0.4874388927526764892, 1.000000000000000000),
 ( 1.000000000000000000, 0.5833547384511119649, 1.000000000000000000),
 ( 1.000000000000000000, 0.6470545345841089979, 1.000000000000000000),
 ( 1.000000000000000000, 0.7045118851637771629, 1.000000000000000000) ) ) 
 REPRESENTATION_ITEM ( '' )  SURFACE ( )  );
#115106=ORIENTED_EDGE ( 'NONE', *, *, #207247, .F. ) ;
#115123=DIRECTION ( 'NONE',  ( -0.7384114592157855483, 0.000000000000000000, 0.6743504407196708739 ) ) ;
#115124=VERTEX_POINT ( 'NONE', #127008 ) ;
#115127=ADVANCED_FACE ( 'NONE', ( #194036 ), #46755, .T. ) ;
#115128=CARTESIAN_POINT ( 'NONE',  ( 0.1368885365587524383, -5.294776013890285959, 10.99935770452674610 ) ) ;
#115154=CARTESIAN_POINT ( 'NONE',  ( 7.019253602638862333, -7.126685749119995528, -7.019253602638886314 ) ) ;
#115187=DIRECTION ( 'NONE',  ( 0.9992060137953822085, 0.000000000000000000, -0.03984146075563027578 ) ) ;
#115197=CARTESIAN_POINT ( 'NONE',  ( 0.000000000000000000, 1.000000000000000888, 0.000000000000000000 ) ) ;
#115211=DIRECTION ( 'NONE',  ( 1.000000000000000000, -2.168404344971003188E-14, 0.000000000000000000 ) ) ;
#115223=ADVANCED_FACE ( 'NONE', ( #94443 ), #113153, .T. ) ;
#115224=CIRCLE ( 'NONE', #142866, 0.08000000000000020983 ) ;
#115232=CARTESIAN_POINT ( 'NONE',  ( -10.88266508516670150, 3.691791674785632082, 3.942622913914227922 ) ) ;
#115247=ORIENTED_EDGE ( 'NONE', *, *, #205822, .T. ) ;
#115265=EDGE_CURVE ( 'NONE', #164527, #163622, #50606, .T. ) ;
#115364=( BOUNDED_SURFACE ( )  B_SPLINE_SURFACE ( 3, 2, ( 
 ( #57316, #207812, #108267 ),
 ( #191557, #174288, #11743 ),
 ( #160146, #23733, #155887 ),
 ( #26928, #25863, #61573 ),
 ( #24797, #59440, #141809 ),
 ( #58381, #123480, #205679 ),
 ( #159078, #107193, #156962 ),
 ( #192624, #109338, #125597 ) ),
 .UNSPECIFIED., .F., .F., .T. ) 
 B_SPLINE_SURFACE_WITH_KNOTS ( ( 4, 2, 2, 4 ),
 ( 3, 3 ),
 ( 0.000000000000000000, 0.0002575597274893397974, 0.0005151194549786795949, 0.001030238909957359190 ),
 ( 0.000000000000000000, 1.000000000000000000 ),
 .UNSPECIFIED. ) 
 GEOMETRIC_REPRESENTATION_ITEM ( )  RATIONAL_B_SPLINE_SURFACE ( (
 ( 1.000000000000000000, 0.9238795325112786339, 1.000000000000000000),
 ( 1.000000000000000000, 0.9228594682463818755, 1.000000000000000000),
 ( 1.000000000000000000, 0.9150875845227504080, 1.000000000000000000),
 ( 1.000000000000000000, 0.8905471774192377232, 1.000000000000000000),
 ( 1.000000000000000000, 0.8740340839248615934, 1.000000000000000000),
 ( 1.000000000000000000, 0.8160099319846065846, 1.000000000000000000),
 ( 1.000000000000000000, 0.7673743911479209423, 1.000000000000000000),
 ( 1.000000000000000000, 0.7100530722070742540, 1.000000000000000000) ) ) 
 REPRESENTATION_ITEM ( '' )  SURFACE ( )  );
#115386=FACE_OUTER_BOUND ( 'NONE', #123666, .T. ) ;
#115399=DIRECTION ( 'NONE',  ( 0.000000000000000000, 0.000000000000000000, 1.000000000000000000 ) ) ;
#115431=CARTESIAN_POINT ( 'NONE',  ( -2.331034670843834533E-15, -6.705807707623487879, 10.34804402329814010 ) ) ;
#115437=EDGE_LOOP ( 'NONE', ( #204579, #138954, #202443, #165392 ) ) ;
#115453=CARTESIAN_POINT ( 'NONE',  ( 0.3525790917594442964, -6.713792789267425398, 9.484899655072640101 ) ) ;
#115470=ORIENTED_EDGE ( 'NONE', *, *, #51769, .F. ) ;
#115475=CARTESIAN_POINT ( 'NONE',  ( -10.00198841339046041, 1.970899860167807605, -6.221464951633984164 ) ) ;
#115479=CARTESIAN_POINT ( 'NONE',  ( 10.99970480906932657, -5.741816521215535651, 0.08058606168009173343 ) ) ;
#115508=AXIS2_PLACEMENT_3D ( 'NONE', #109507, #192794, #77994 ) ;
#115577=ORIENTED_EDGE ( 'NONE', *, *, #124727, .T. ) ;
#115581=CARTESIAN_POINT ( 'NONE',  ( 2.020417662918754687, 3.956598013261175772, -11.36521191596581737 ) ) ;
#115590=CARTESIAN_POINT ( 'NONE',  ( 8.966186108929086629, 2.441452740530747345, 7.552575952455595321 ) ) ;
#115604=AXIS2_PLACEMENT_3D ( 'NONE', #156031, #38016, #169072 ) ;
#115638=ORIENTED_EDGE ( 'NONE', *, *, #6898, .F. ) ;
#115639=ADVANCED_FACE ( 'NONE', ( #202541 ), #139744, .T. ) ;
#115642=AXIS2_PLACEMENT_3D ( 'NONE', #19540, #133343, #118187 ) ;
#115658=B_SPLINE_CURVE_WITH_KNOTS ( 'NONE', 3,
 ( #150918, #2480, #52337, #213219, #126744, #62712 ),
 .UNSPECIFIED., .F., .F.,
 ( 4, 2, 4 ),
 ( 2.168404344970997553E-19, 0.001225895755212360813, 0.002451791510424720759 ),
 .UNSPECIFIED. ) ;
#115686=ORIENTED_EDGE ( 'NONE', *, *, #3792, .T. ) ;
#115691=CIRCLE ( 'NONE', #56747, 11.69999999999999041 ) ;
#115695=EDGE_CURVE ( 'NONE', #172181, #78601, #143322, .T. ) ;
#115704=CARTESIAN_POINT ( 'NONE',  ( 10.48884024596648601, 1.000000000000000888, -5.608780650328974104 ) ) ;
#115731=SURFACE_STYLE_USAGE ( .BOTH. , #65821 ) ;
#115776=EDGE_CURVE ( 'NONE', #31452, #121557, #15232, .T. ) ;
#115814=CIRCLE ( 'NONE', #91503, 0.07999999999999984901 ) ;
#115824=PRESENTATION_STYLE_ASSIGNMENT (( #49696 ) ) ;
#115832=CARTESIAN_POINT ( 'NONE',  ( -9.566809970446467304, -7.630846356335648117, 9.989423754102837008E-15 ) ) ;
#115834=CARTESIAN_POINT ( 'NONE',  ( -9.242574560015905050, -9.438200158419387975, 0.5964493340168121049 ) ) ;
#115899=EDGE_CURVE ( 'NONE', #71638, #101997, #120531, .T. ) ;
#115907=CARTESIAN_POINT ( 'NONE',  ( 6.949925879317214950, -6.532648833121268872, -6.447267651612722084 ) ) ;
#115960=COLOUR_RGB ( '', 0.09019608, 0.27058824, 0.51372549) ;
#115982=VERTEX_POINT ( 'NONE', #57389 ) ;
#116011=CARTESIAN_POINT ( 'NONE',  ( 0.000000000000000000, -9.999999999999994671, 0.000000000000000000 ) ) ;
#116013=FILL_AREA_STYLE_COLOUR ( '', #117030 ) ;
#116020=FILL_AREA_STYLE_COLOUR ( '', #151464 ) ;
#116055=CARTESIAN_POINT ( 'NONE',  ( 0.000000000000000000, -0.02379966007286238305, 0.000000000000000000 ) ) ;
#116084=UNCERTAINTY_MEASURE_WITH_UNIT (LENGTH_MEASURE( 1.000000000000000082E-05 ), #11767, 'distance_accuracy_value', 'NONE');
#116115=DIRECTION ( 'NONE',  ( 0.7384114592165702540, -8.251132798224216436E-15, -0.6743504407188115612 ) ) ;
#116155=AXIS2_PLACEMENT_3D ( 'NONE', #57548, #123706, #8785 ) ;
#116157=CARTESIAN_POINT ( 'NONE',  ( 7.047919420689662040, -8.186910006423167019, -6.389500220311202128 ) ) ;
#116162=DIRECTION ( 'NONE',  ( -0.000000000000000000, 1.000000000000000000, -0.000000000000000000 ) ) ;
#116223=CARTESIAN_POINT ( 'NONE',  ( -6.598949805828081772, -8.057948861126607909, -6.880414557363810246 ) ) ;
#116244=CARTESIAN_POINT ( 'NONE',  ( -3.659182332138577465E-15, -7.246166700193014343, 9.579665964947889023 ) ) ;
#116257=PLANE ( 'NONE',  #191803 ) ;
#116269=AXIS2_PLACEMENT_3D ( 'NONE', #53411, #116342, #119548 ) ;
#116305=ORIENTED_EDGE ( 'NONE', *, *, #196046, .F. ) ;
#116313=VECTOR ( 'NONE', #163621, 1000.000000000000000 ) ;
#116342=DIRECTION ( 'NONE',  ( 0.000000000000000000, 1.000000000000000000, 0.000000000000000000 ) ) ;
#116385=VERTEX_POINT ( 'NONE', #142945 ) ;
#116390=MECHANICAL_DESIGN_GEOMETRIC_PRESENTATION_REPRESENTATION('',(#154368),#60985);
#116439=DIRECTION ( 'NONE',  ( 0.000000000000000000, -1.000000000000000000, 0.000000000000000000 ) ) ;
#116474=VECTOR ( 'NONE', #194562, 1000.000000000000000 ) ;
#116526=ORIENTED_EDGE ( 'NONE', *, *, #89254, .T. ) ;
#116535=CARTESIAN_POINT ( 'NONE',  ( 10.99896775280371131, -5.324706741106397523, -0.1653080603930866532 ) ) ;
#116618=CIRCLE ( 'NONE', #182250, 0.07999999999999993228 ) ;
#116629=ORIENTED_EDGE ( 'NONE', *, *, #186483, .F. ) ;
#116636=EDGE_CURVE ( 'NONE', #55414, #170100, #108857, .T. ) ;
#116642=CARTESIAN_POINT ( 'NONE',  ( 9.499679971350916574, -7.185026885903947225, 0.07802162204196347317 ) ) ;
#116666=CARTESIAN_POINT ( 'NONE',  ( 0.08832626591284459261, -9.919998018383680005, 9.499595568239961096 ) ) ;
#116674=CARTESIAN_POINT ( 'NONE',  ( -10.32992389895503393, 1.000000000000000888, -6.106772653521458594 ) ) ;
#116714=CARTESIAN_POINT ( 'NONE',  ( 0.4365953560983709680, -5.836144560139977955, 10.35465518852992339 ) ) ;
#116756=VECTOR ( 'NONE', #207174, 1000.000000000000000 ) ;
#116802=CARTESIAN_POINT ( 'NONE',  ( 9.578539647746881158, -9.962495449538966596, -0.1460552299441071622 ) ) ;
#116819=EDGE_LOOP ( 'NONE', ( #52365, #65335, #98281 ) ) ;
#116857=VERTEX_POINT ( 'NONE', #8011 ) ;
#116873=CONICAL_SURFACE ( 'NONE', #179134, 10.99999999999999112, 0.7853981633974479459 ) ;
#116874=AXIS2_PLACEMENT_3D ( 'NONE', #206222, #158559, #207294 ) ;
#116889=( NAMED_UNIT ( * ) SI_UNIT ( $, .STERADIAN. ) SOLID_ANGLE_UNIT ( ) );
#116901=ORIENTED_EDGE ( 'NONE', *, *, #113228, .F. ) ;
#116921=CARTESIAN_POINT ( 'NONE',  ( -1.734723475976807094E-15, -6.054403199333757257, -10.91970695577494332 ) ) ;
#116949=B_SPLINE_CURVE_WITH_KNOTS ( 'NONE', 3,
 ( #191280, #175072, #26659, #90624, #110123, #158807, #192346, #44004 ),
 .UNSPECIFIED., .F., .F.,
 ( 4, 2, 2, 4 ),
 ( 1.068270986634163351E-15, 0.0004443203323512407137, 0.0006664804985263248242, 0.0008886406647014088262 ),
 .UNSPECIFIED. ) ;
#116959=( BOUNDED_SURFACE ( )  B_SPLINE_SURFACE ( 3, 2, ( 
 ( #202956, #56733, #25290 ),
 ( #71885, #157451, #9045 ),
 ( #40497, #120745, #37277 ),
 ( #104423, #170471, #5809 ) ),
 .UNSPECIFIED., .F., .F., .T. ) 
 B_SPLINE_SURFACE_WITH_KNOTS ( ( 4, 4 ),
 ( 3, 3 ),
 ( 0.06089844177390838637, 0.06334004522945697879 ),
 ( 0.000000000000000000, 1.000000000000000000 ),
 .UNSPECIFIED. ) 
 GEOMETRIC_REPRESENTATION_ITEM ( )  RATIONAL_B_SPLINE_SURFACE ( (
 ( 1.000000000000000000, 0.7169884966214686850, 1.000000000000000000),
 ( 1.000000000000000000, 0.7174883642159506358, 1.000000000000000000),
 ( 1.000000000000000000, 0.7180610417775397103, 1.000000000000000000),
 ( 1.000000000000000000, 0.7187540717311186045, 1.000000000000000000) ) ) 
 REPRESENTATION_ITEM ( '' )  SURFACE ( )  );
#117015=( BOUNDED_SURFACE ( )  B_SPLINE_SURFACE ( 3, 2, ( 
 ( #162663, #14232, #146428 ),
 ( #212442, #136556, #21682 ),
 ( #125447, #169035, #201509 ),
 ( #141657, #185272, #207669 ),
 ( #3309, #167974, #36895 ),
 ( #69379, #37977, #175200 ),
 ( #184208, #121444, #104050 ),
 ( #135487, #134446, #118222 ) ),
 .UNSPECIFIED., .F., .F., .T. ) 
 B_SPLINE_SURFACE_WITH_KNOTS ( ( 4, 2, 2, 4 ),
 ( 3, 3 ),
 ( -5.421010862427522170E-20, 0.0004401918256853618126, 0.0006602877385280428273, 0.0008803836513707237335 ),
 ( 0.000000000000000000, 1.000000000000000000 ),
 .UNSPECIFIED. ) 
 GEOMETRIC_REPRESENTATION_ITEM ( )  RATIONAL_B_SPLINE_SURFACE ( (
 ( 1.000000000000000000, 0.6787756258918289376, 1.000000000000000000),
 ( 1.000000000000000000, 0.6284487096095630054, 1.000000000000000000),
 ( 1.000000000000000000, 0.5704014816688967038, 1.000000000000000000),
 ( 1.000000000000000000, 0.4882303283126627758, 1.000000000000000000),
 ( 1.000000000000000000, 0.4617370933882599671, 1.000000000000000000),
 ( 1.000000000000000000, 0.4222438920368223325, 1.000000000000000000),
 ( 1.000000000000000000, 0.4105126989449003894, 1.000000000000000000),
 ( 1.000000000000000000, 0.4127341956165074266, 1.000000000000000000) ) ) 
 REPRESENTATION_ITEM ( '' )  SURFACE ( )  );
#117025=EDGE_LOOP ( 'NONE', ( #108784, #194334, #81257, #25201 ) ) ;
#117030=COLOUR_RGB ( '', 0.08235294, 0.09019608, 0.10196078) ;
#117031=MECHANICAL_DESIGN_GEOMETRIC_PRESENTATION_REPRESENTATION('',(#23569),#134319);
#117046=ORIENTED_EDGE ( 'NONE', *, *, #190633, .F. ) ;
#117048=ORIENTED_EDGE ( 'NONE', *, *, #101175, .F. ) ;
#117106=CARTESIAN_POINT ( 'NONE',  ( 9.499771308870721853, -7.644320505141724453, 0.06917019444585296994 ) ) ;
#117114=CARTESIAN_POINT ( 'NONE',  ( 0.000000000000000000, -0.02379966007286238305, 0.000000000000000000 ) ) ;
#117115=DIRECTION ( 'NONE',  ( -0.6762880771785059197, 1.295290445962756284E-12, -0.7366372490352354196 ) ) ;
#117117=CARTESIAN_POINT ( 'NONE',  ( -5.204170427930421283E-15, 3.447199233515649386, -11.99999999999998224 ) ) ;
#117148=( BOUNDED_SURFACE ( )  B_SPLINE_SURFACE ( 3, 2, ( 
 ( #38951, #102885, #168943 ),
 ( #155904, #23749, #20545 ),
 ( #21589, #89853, #35738 ),
 ( #101813, #85556, #151646 ) ),
 .UNSPECIFIED., .F., .F., .T. ) 
 B_SPLINE_SURFACE_WITH_KNOTS ( ( 4, 4 ),
 ( 3, 3 ),
 ( 0.06089817005132014405, 0.06334004685008763624 ),
 ( 0.000000000000000000, 1.000000000000000000 ),
 .UNSPECIFIED. ) 
 GEOMETRIC_REPRESENTATION_ITEM ( )  RATIONAL_B_SPLINE_SURFACE ( (
 ( 1.000000000000000000, 0.7169883299104515828, 1.000000000000000000),
 ( 1.000000000000000000, 0.7174882367719609411, 1.000000000000000000),
 ( 1.000000000000000000, 0.7180609655865438645, 1.000000000000000000),
 ( 1.000000000000000000, 0.7187540731123145399, 1.000000000000000000) ) ) 
 REPRESENTATION_ITEM ( '' )  SURFACE ( )  );
#117156=ORIENTED_EDGE ( 'NONE', *, *, #63645, .F. ) ;
#117167=ORIENTED_EDGE ( 'NONE', *, *, #41532, .F. ) ;
#117192=ADVANCED_FACE ( 'NONE', ( #194244 ), #167539, .T. ) ;
#117209=LINE ( 'NONE', #66225, #152712 ) ;
#117213=CARTESIAN_POINT ( 'NONE',  ( -2.088542702721619460, 3.956598013261175772, 11.35310118413588931 ) ) ;
#117217=( NAMED_UNIT ( * ) SI_UNIT ( $, .STERADIAN. ) SOLID_ANGLE_UNIT ( ) );
#117228=CARTESIAN_POINT ( 'NONE',  ( 0.1305260785387470923, -7.912329794880671230, -10.96023284214814986 ) ) ;
#117238=CARTESIAN_POINT ( 'NONE',  ( -8.919266336782142091, 2.972657967447086769, -7.510420563958255968 ) ) ;
#117290=CARTESIAN_POINT ( 'NONE',  ( -6.731761806397366321, -7.792646766724930174, -6.779954559072856490 ) ) ;
#117381=DIRECTION ( 'NONE',  ( 0.000000000000000000, -1.000000000000000000, 0.000000000000000000 ) ) ;
#117404=PRESENTATION_STYLE_ASSIGNMENT (( #82694 ) ) ;
#117446=EDGE_CURVE ( 'NONE', #196061, #109058, #70725, .T. ) ;
#117457=DIRECTION ( 'NONE',  ( 0.000000000000000000, 0.000000000000000000, -1.000000000000000000 ) ) ;
#117468=CARTESIAN_POINT ( 'NONE',  ( -1.040834085586084257E-14, 0.000000000000000000, -9.579665964948867796 ) ) ;
#117476=CARTESIAN_POINT ( 'NONE',  ( -2.373851744317279522, 1.000000000000000888, 11.76285798163022100 ) ) ;
#117513=CARTESIAN_POINT ( 'NONE',  ( 0.4694063952341808177, -6.893137084989842123, 10.98997987423603995 ) ) ;
#117514=CARTESIAN_POINT ( 'NONE',  ( 7.346809171966453889, -6.836568542494980250, 8.002408263930263388 ) ) ;
#117553=CARTESIAN_POINT ( 'NONE',  ( 9.496663239506002441, -6.863887327018314721, 0.01979922387980803319 ) ) ;
#117570=CARTESIAN_POINT ( 'NONE',  ( -6.692370362267773487, -7.020359948792200377, -6.743487189266383908 ) ) ;
#117578=ADVANCED_FACE ( 'NONE', ( #33871 ), #116257, .F. ) ;
#117622=FACE_OUTER_BOUND ( 'NONE', #40670, .T. ) ;
#117641=DIRECTION ( 'NONE',  ( 0.000000000000000000, 1.000000000000000000, 0.000000000000000000 ) ) ;
#117706=EDGE_CURVE ( 'NONE', #43490, #15455, #112265, .T. ) ;
#117720=CARTESIAN_POINT ( 'NONE',  ( 9.500370076773496208, -7.189371949516623950, -0.005973655271256667759 ) ) ;
#117726=DIRECTION ( 'NONE',  ( 0.000000000000000000, 0.000000000000000000, 1.000000000000000000 ) ) ;
#117731=DIRECTION ( 'NONE',  ( -0.9992060137953822085, -3.484297484817962848E-16, 0.03984146075563036599 ) ) ;
#117769=CARTESIAN_POINT ( 'NONE',  ( -7.712222144929068435, -6.293595771080859436, 7.712222144929100409 ) ) ;
#117772=CARTESIAN_POINT ( 'NONE',  ( -9.860259297219579722, -8.821010173593817782, 0.6081441828345716116 ) ) ;
#117786=EDGE_LOOP ( 'NONE', ( #194070, #138965, #172234, #97081, #29257 ) ) ;
#117833=DIRECTION ( 'NONE',  ( 0.000000000000000000, 0.000000000000000000, 1.000000000000000000 ) ) ;
#117856=VERTEX_POINT ( 'NONE', #52264 ) ;
#117872=CARTESIAN_POINT ( 'NONE',  ( -6.445605026751819899, -8.233137084989717636, -6.979380938965669579 ) ) ;
#117880=SURFACE_STYLE_USAGE ( .BOTH. , #150329 ) ;
#117894=CARTESIAN_POINT ( 'NONE',  ( 0.08522875510948167699, -9.999176759342304877, 10.91956886450205033 ) ) ;
#117897=ORIENTED_EDGE ( 'NONE', *, *, #63311, .F. ) ;
#117960=CARTESIAN_POINT ( 'NONE',  ( -7.446209719563359641, -5.223431457505076203, -8.064677165291183059 ) ) ;
#117961=DIRECTION ( 'NONE',  ( 0.000000000000000000, -1.000000000000000000, 0.000000000000000000 ) ) ;
#117967=EDGE_CURVE ( 'NONE', #83638, #200016, #101829, .T. ) ;
#117997=EDGE_CURVE ( 'NONE', #114100, #186393, #22326, .T. ) ;
#118002=B_SPLINE_CURVE_WITH_KNOTS ( 'NONE', 3,
 ( #196441, #149833, #63235, #97893, #166070, #145604 ),
 .UNSPECIFIED., .F., .F.,
 ( 4, 2, 4 ),
 ( 0.000000000000000000, 0.001226111284895915667, 0.002452222569791831334 ),
 .UNSPECIFIED. ) ;
#118016=CARTESIAN_POINT ( 'NONE',  ( 8.912450614902654777, 3.507114751586604129, 8.024806578262976942 ) ) ;
#118027=DIRECTION ( 'NONE',  ( -0.000000000000000000, -1.000000000000000000, -0.000000000000000000 ) ) ;
#118052=CARTESIAN_POINT ( 'NONE',  ( 0.000000000000000000, 4.006659545634088992, 0.000000000000000000 ) ) ;
#118081=CARTESIAN_POINT ( 'NONE',  ( -0.08118383494907006892, -9.908729948657656550, -9.499653137018302829 ) ) ;
#118094=CARTESIAN_POINT ( 'NONE',  ( 0.1480828224388863745, -6.655928102866957907, 10.87712779691740117 ) ) ;
#118097=ORIENTED_EDGE ( 'NONE', *, *, #51127, .F. ) ;
#118098=EDGE_CURVE ( 'NONE', #69637, #110438, #120120, .T. ) ;
#118116=DIRECTION ( 'NONE',  ( -1.000000000000000000, 0.000000000000000000, 0.000000000000000000 ) ) ;
#118150=DIRECTION ( 'NONE',  ( 0.000000000000000000, 1.000000000000000000, 0.000000000000000000 ) ) ;
#118160=CARTESIAN_POINT ( 'NONE',  ( -5.204170427930421283E-15, -6.268611901546719878, 10.55819884875827519 ) ) ;
#118169=ORIENTED_EDGE ( 'NONE', *, *, #9358, .T. ) ;
#118178=LINE ( 'NONE', #183107, #160304 ) ;
#118185=ORIENTED_EDGE ( 'NONE', *, *, #72448, .T. ) ;
#118186=FILL_AREA_STYLE_COLOUR ( '', #171933 ) ;
#118187=DIRECTION ( 'NONE',  ( 0.000000000000000000, 0.000000000000000000, -1.000000000000000000 ) ) ;
#118222=CARTESIAN_POINT ( 'NONE',  ( -6.999862025036994062, -6.532648833121176501, 6.392587740394330531 ) ) ;
#118245=VERTEX_POINT ( 'NONE', #109628 ) ;
#118273=VERTEX_POINT ( 'NONE', #26154 ) ;
#118296=CARTESIAN_POINT ( 'NONE',  ( 0.000000000000000000, 3.000000000000002665, 0.000000000000000000 ) ) ;
#118361=CARTESIAN_POINT ( 'NONE',  ( -10.99949329275129450, -9.914220445327725173, 0.1055954338740902887 ) ) ;
#118371=CARTESIAN_POINT ( 'NONE',  ( 9.906083622534509914, -9.418601272609043562, -0.1729113328156559048 ) ) ;
#118378=CARTESIAN_POINT ( 'NONE',  ( 0.04234008746931722245, -7.776896528353615778, 9.555169238417180466 ) ) ;
#118387=CARTESIAN_POINT ( 'NONE',  ( 0.2534910766302467255, 3.934660213246443661, -11.56267633880226775 ) ) ;
#118391=DIRECTION ( 'NONE',  ( -0.000000000000000000, 1.000000000000000000, -0.000000000000000000 ) ) ;
#118406=EDGE_CURVE ( 'NONE', #54210, #159016, #160742, .T. ) ;
#118422=CARTESIAN_POINT ( 'NONE',  ( -0.08058608058608696112, -5.907420853759267843, 10.99970480893081870 ) ) ;
#118428=CARTESIAN_POINT ( 'NONE',  ( -11.10517813317449054, 1.720726420432414860, 4.015189785735357120 ) ) ;
#118470=CARTESIAN_POINT ( 'NONE',  ( -0.01979919457417661857, -6.863887352872468206, 9.496663240426189034 ) ) ;
#118471=FILL_AREA_STYLE_COLOUR ( '', #204094 ) ;
#118493=ORIENTED_EDGE ( 'NONE', *, *, #178012, .T. ) ;
#118522=LINE ( 'NONE', #67540, #78167 ) ;
#118553=EDGE_CURVE ( 'NONE', #93109, #195316, #136479, .T. ) ;
#118577=CARTESIAN_POINT ( 'NONE',  ( 6.396834479292349052, -8.176568542494905500, 7.055228938194280985 ) ) ;
#118591=ORIENTED_EDGE ( 'NONE', *, *, #34900, .F. ) ;
#118598=MECHANICAL_DESIGN_GEOMETRIC_PRESENTATION_REPRESENTATION('',(#108249),#156595);
#118601=AXIS2_PLACEMENT_3D ( 'NONE', #59060, #158704, #30586 ) ;
#118624=CARTESIAN_POINT ( 'NONE',  ( 6.940534579974978691, -6.675176078274695612, -6.653311379900283207 ) ) ;
#118685=CARTESIAN_POINT ( 'NONE',  ( 6.777910281175842044, -7.189645481333912791, -6.776323679500925401 ) ) ;
#118687=ORIENTED_EDGE ( 'NONE', *, *, #134985, .T. ) ;
#118774=ORIENTED_EDGE ( 'NONE', *, *, #122755, .T. ) ;
#118785=CONICAL_SURFACE ( 'NONE', #191373, 8.368490868537556082, 0.7853981633974479459 ) ;
#118812=CARTESIAN_POINT ( 'NONE',  ( -9.622669940282571943, -9.063128755109497448, 0.5283818209470610983 ) ) ;
#118844=ORIENTED_EDGE ( 'NONE', *, *, #89525, .T. ) ;
#118875=ORIENTED_EDGE ( 'NONE', *, *, #158609, .F. ) ;
#118882=DIRECTION ( 'NONE',  ( 0.000000000000000000, 0.000000000000000000, 1.000000000000000000 ) ) ;
#118898=FACE_OUTER_BOUND ( 'NONE', #163880, .T. ) ;
#118902=AXIS2_PLACEMENT_3D ( 'NONE', #46993, #96819, #28595 ) ;
#118916=EDGE_CURVE ( 'NONE', #9078, #161735, #152702, .T. ) ;
#118922=EDGE_LOOP ( 'NONE', ( #126546, #2972, #44508 ) ) ;
#118961=CARTESIAN_POINT ( 'NONE',  ( -10.91804383151493241, -9.900000000000074962, 0.1905751639682748966 ) ) ;
#118963=ORIENTED_EDGE ( 'NONE', *, *, #182421, .F. ) ;
#119000=ORIENTED_EDGE ( 'NONE', *, *, #39457, .F. ) ;
#119003=VERTEX_POINT ( 'NONE', #69290 ) ;
#119033=CARTESIAN_POINT ( 'NONE',  ( -7.720982897393577460, -6.307829212974239042, 7.834948825496934610 ) ) ;
#119034=CARTESIAN_POINT ( 'NONE',  ( -9.499668754586236830, -7.643695121331953501, -0.07933191752404977759 ) ) ;
#119057=EDGE_CURVE ( 'NONE', #172976, #186393, #88983, .T. ) ;
#119080=CARTESIAN_POINT ( 'NONE',  ( 8.787802685836132000, 3.956598013261175772, 7.485281629513396595 ) ) ;
#119092=SPHERICAL_SURFACE ( 'NONE', #208240, 9.500000000000001776 ) ;
#119111=CARTESIAN_POINT ( 'NONE',  ( 8.955454528940892445, 3.019799309333439652, 8.063527476383637094 ) ) ;
#119127=DIRECTION ( 'NONE',  ( 0.000000000000000000, 0.000000000000000000, -1.000000000000000000 ) ) ;
#119140=ORIENTED_EDGE ( 'NONE', *, *, #48296, .F. ) ;
#119158=CARTESIAN_POINT ( 'NONE',  ( 7.636191794455555737, -6.027819618361855092, 7.636191794455528203 ) ) ;
#119164=CARTESIAN_POINT ( 'NONE',  ( -9.573337995800486055, -7.550885189219930460, 5.228734383400795993E-15 ) ) ;
#119166=EDGE_CURVE ( 'NONE', #15288, #31452, #164301, .T. ) ;
#119183=FACE_OUTER_BOUND ( 'NONE', #180784, .T. ) ;
#119214=EDGE_LOOP ( 'NONE', ( #101658, #208553, #25316, #66132 ) ) ;
#119249=SURFACE_STYLE_FILL_AREA ( #35794 ) ;
#119250=CARTESIAN_POINT ( 'NONE',  ( -0.08000000000000714873, -5.907420853759267843, 10.91970695577494865 ) ) ;
#119254=DIRECTION ( 'NONE',  ( -0.9992060137953822085, 0.000000000000000000, 0.03984146075563027578 ) ) ;
#119259=CARTESIAN_POINT ( 'NONE',  ( 10.41272866534396435, -5.796408561409281290, 1.485228241937698088E-12 ) ) ;
#119293=CARTESIAN_POINT ( 'NONE',  ( 7.385065802799687162, -6.893137084989842123, 8.044078759455205230 ) ) ;
#119296=ORIENTED_EDGE ( 'NONE', *, *, #92379, .F. ) ;
#119302=VERTEX_POINT ( 'NONE', #10699 ) ;
#119332=CARTESIAN_POINT ( 'NONE',  ( -7.882977371601947780, -5.341768514962232040, 7.624693973552358450 ) ) ;
#119360=DIRECTION ( 'NONE',  ( 0.000000000000000000, 0.000000000000000000, 1.000000000000000000 ) ) ;
#119366=VERTEX_POINT ( 'NONE', #126684 ) ;
#119372=AXIS2_PLACEMENT_3D ( 'NONE', #54433, #170299, #134641 ) ;
#119379=CIRCLE ( 'NONE', #25901, 10.97656854249491332 ) ;
#119396=CARTESIAN_POINT ( 'NONE',  ( 10.18461545817735470, 3.956598013261175772, -5.433575010662928584 ) ) ;
#119420=CARTESIAN_POINT ( 'NONE',  ( 0.003376046620571365731, -7.161464053357560644, 9.586610838029431036 ) ) ;
#119421=CARTESIAN_POINT ( 'NONE',  ( -6.392587740394328755, -6.532648833121157850, -6.999862025036979851 ) ) ;
#119429=CARTESIAN_POINT ( 'NONE',  ( 9.499623061593991835, -9.908700546396012498, -0.08463495275094053139 ) ) ;
#119440=CARTESIAN_POINT ( 'NONE',  ( 0.000000000000000000, 7.849261790823902629, 0.000000000000000000 ) ) ;
#119447=CARTESIAN_POINT ( 'NONE',  ( 6.710127771514622808, -7.162053774861990796, 6.725445687907760650 ) ) ;
#119448=EDGE_CURVE ( 'NONE', #16465, #129112, #153949, .T. ) ;
#119459=DIRECTION ( 'NONE',  ( 1.776356839400250465E-15, 0.000000000000000000, -1.000000000000000000 ) ) ;
#119469=AXIS2_PLACEMENT_3D ( 'NONE', #72367, #153644, #170946 ) ;
#119482=CARTESIAN_POINT ( 'NONE',  ( 7.721398836998367265, -6.134628647623499909, -7.721398836998390358 ) ) ;
#119490=DIRECTION ( 'NONE',  ( 0.9998476951563912696, 0.000000000000000000, -0.01745240643728004568 ) ) ;
#119525=AXIS2_PLACEMENT_3D ( 'NONE', #172130, #106109, #23725 ) ;
#119533=B_SPLINE_CURVE_WITH_KNOTS ( 'NONE', 3,
 ( #23924, #90029, #156085, #107394, #179796, #128991, #15131, #143068, #159269, #30351 ),
 .UNSPECIFIED., .F., .F.,
 ( 4, 2, 2, 2, 4 ),
 ( 3.274218758650651739E-18, 0.0002021113321160316874, 0.0004042226642320600680, 0.0006063339963480846809, 0.0008084453284641086434 ),
 .UNSPECIFIED. ) ;
#119536=CARTESIAN_POINT ( 'NONE',  ( 7.714278451735655587E-14, -9.900000000000003908, 11.00029519899101160 ) ) ;
#119548=DIRECTION ( 'NONE',  ( 0.000000000000000000, 0.000000000000000000, 1.000000000000000000 ) ) ;
#119592=FACE_OUTER_BOUND ( 'NONE', #194742, .T. ) ;
#119616=EDGE_CURVE ( 'NONE', #194102, #184826, #107056, .T. ) ;
#119617=CARTESIAN_POINT ( 'NONE',  ( 7.404765023120892131, -6.836271202499960786, 7.949604103952387035 ) ) ;
#119639=DIRECTION ( 'NONE',  ( 0.000000000000000000, 0.000000000000000000, -1.000000000000000000 ) ) ;
#119655=CARTESIAN_POINT ( 'NONE',  ( 0.1025498324992813182, -6.714092063936424992, 10.99981089498244380 ) ) ;
#119661=ORIENTED_EDGE ( 'NONE', *, *, #200299, .F. ) ;
#119665=LINE ( 'NONE', #154244, #79923 ) ;
#119694=CARTESIAN_POINT ( 'NONE',  ( 6.895452369244176261, -6.747656629766812131, -6.524021554744646956 ) ) ;
#119705=CARTESIAN_POINT ( 'NONE',  ( -8.673617379884035472E-15, 3.487142912321097299, -11.99525683304594281 ) ) ;
#119730=CIRCLE ( 'NONE', #53965, 0.08000000000000080658 ) ;
#119756=VERTEX_POINT ( 'NONE', #79970 ) ;
#119763=DIRECTION ( 'NONE',  ( -0.8660254037844399289, 0.000000000000000000, -0.4999999999999978351 ) ) ;
#119773=CARTESIAN_POINT ( 'NONE',  ( 9.905860218026550257, -6.920331743278818948, 9.269928574751062911E-15 ) ) ;
#119796=CARTESIAN_POINT ( 'NONE',  ( -6.781144757626059061, -7.161464053357560644, 6.776370306708066948 ) ) ;
#119825=( GEOMETRIC_REPRESENTATION_CONTEXT ( 3 ) GLOBAL_UNCERTAINTY_ASSIGNED_CONTEXT ( ( #191672 ) ) GLOBAL_UNIT_ASSIGNED_CONTEXT ( ( #196303, #178999, #47949 ) ) REPRESENTATION_CONTEXT ( 'NONE', 'WORKASPACE' ) );
#119841=ORIENTED_EDGE ( 'NONE', *, *, #60250, .T. ) ;
#119851=CARTESIAN_POINT ( 'NONE',  ( -10.49201538390856037, 0.9691415390508770766, 5.610609371109086752 ) ) ;
#119865=DIRECTION ( 'NONE',  ( 0.000000000000000000, -1.000000000000000000, 0.000000000000000000 ) ) ;
#119896=ORIENTED_EDGE ( 'NONE', *, *, #42077, .F. ) ;
#119906=DIRECTION ( 'NONE',  ( -0.000000000000000000, 1.000000000000000000, -0.000000000000000000 ) ) ;
#119978=ADVANCED_FACE ( 'NONE', ( #95186 ), #95197, .T. ) ;
#120011=CARTESIAN_POINT ( 'NONE',  ( -6.506745451169519079, -8.202869699938538872, -6.922231005658564307 ) ) ;
#120025=EDGE_LOOP ( 'NONE', ( #87913, #2329, #77704, #125909 ) ) ;
#120038=EDGE_LOOP ( 'NONE', ( #9853, #213762, #11630, #69396, #103030, #131280 ) ) ;
#120104=ADVANCED_FACE ( 'NONE', ( #183871 ), #122955, .T. ) ;
#120120=B_SPLINE_CURVE_WITH_KNOTS ( 'NONE', 3,
 ( #184379, #37067, #101000, #168147, #151906, #20800, #152963, #54403 ),
 .UNSPECIFIED., .F., .F.,
 ( 4, 2, 2, 4 ),
 ( 6.054694391546165775E-16, 0.0001985720215092564753, 0.0003971440430179074780, 0.0007942880860352082364 ),
 .UNSPECIFIED. ) ;
#120126=( BOUNDED_SURFACE ( )  B_SPLINE_SURFACE ( 3, 2, ( 
 ( #89246, #155297, #139060 ),
 ( #205088, #162779, #110878 ),
 ( #65237, #43701, #80447 ),
 ( #45834, #114095, #93518 ) ),
 .UNSPECIFIED., .F., .F., .F. ) 
 B_SPLINE_SURFACE_WITH_KNOTS ( ( 4, 4 ),
 ( 3, 3 ),
 ( 0.000000000000000000, 9.170893476602526924E-05 ),
 ( 0.000000000000000000, 1.000000000000000000 ),
 .UNSPECIFIED. ) 
 GEOMETRIC_REPRESENTATION_ITEM ( )  RATIONAL_B_SPLINE_SURFACE ( (
 ( 1.000000000000000000, 0.7100530722026773267, 1.000000000000000000),
 ( 1.000000000000000000, 0.6998898451682588062, 1.000000000000000000),
 ( 1.000000000000000000, 0.6894756946157454269, 1.000000000000000000),
 ( 1.000000000000000000, 0.6787756258918318242, 1.000000000000000000) ) ) 
 REPRESENTATION_ITEM ( '' )  SURFACE ( )  );
#120183=CARTESIAN_POINT ( 'NONE',  ( 8.912450614902654777, 3.507114751586604129, 8.024806578262976942 ) ) ;
#120191=( LENGTH_UNIT ( ) NAMED_UNIT ( * ) SI_UNIT ( .MILLI., .METRE. ) );
#120207=( LENGTH_UNIT ( ) NAMED_UNIT ( * ) SI_UNIT ( .MILLI., .METRE. ) );
#120222=CARTESIAN_POINT ( 'NONE',  ( 8.042162931142705418, -6.699677480914211891, -7.505515594164287485 ) ) ;
#120223=CARTESIAN_POINT ( 'NONE',  ( -0.08865135991733066878, -9.916958638733639475, -9.499586356067535320 ) ) ;
#120235=ORIENTED_EDGE ( 'NONE', *, *, #187696, .T. ) ;
#120239=CARTESIAN_POINT ( 'NONE',  ( 7.465774003072967346, -6.268611901546719878, 7.465774003072962017 ) ) ;
#120253=( NAMED_UNIT ( * ) PLANE_ANGLE_UNIT ( ) SI_UNIT ( $, .RADIAN. ) );
#120261=AXIS2_PLACEMENT_3D ( 'NONE', #12884, #177551, #129942 ) ;
#120273=CARTESIAN_POINT ( 'NONE',  ( 2.179728514415657799E-12, -5.796408561409501559, -10.41272866534444752 ) ) ;
#120291=CIRCLE ( 'NONE', #85744, 0.08000000000000020983 ) ;
#120296=ORIENTED_EDGE ( 'NONE', *, *, #173466, .F. ) ;
#120367=CARTESIAN_POINT ( 'NONE',  ( 7.721398836998361048, -5.907420853759298041, -7.721398836998386805 ) ) ;
#120392=DIRECTION ( 'NONE',  ( 0.000000000000000000, 1.000000000000000000, 0.000000000000000000 ) ) ;
#120411=CARTESIAN_POINT ( 'NONE',  ( -7.847520364415487393, -5.402328468025377362, 7.653681110113387476 ) ) ;
#120425=DIRECTION ( 'NONE',  ( 0.000000000000000000, -1.000000000000000000, 0.000000000000000000 ) ) ;
#120494=VERTEX_POINT ( 'NONE', #151933 ) ;
#120509=CARTESIAN_POINT ( 'NONE',  ( -6.608557002163582439, -8.105676417795779187, -6.825099317097834017 ) ) ;
#120524=ORIENTED_EDGE ( 'NONE', *, *, #131051, .T. ) ;
#120525=CARTESIAN_POINT ( 'NONE',  ( -0.1000000000000028644, -9.919999999999998153, -9.579478065113972818 ) ) ;
#120531=B_SPLINE_CURVE_WITH_KNOTS ( 'NONE', 3,
 ( #72558, #74709, #71479, #22727, #171134, #75773, #106193 ),
 .UNSPECIFIED., .F., .F.,
 ( 4, 3, 4 ),
 ( 0.0001932293135873497478, 0.0009000000018422023643, 0.002089330742406760120 ),
 .UNSPECIFIED. ) ;
#120537=CARTESIAN_POINT ( 'NONE',  ( 0.000000000000000000, 0.000000000000000000, 0.000000000000000000 ) ) ;
#120539=CARTESIAN_POINT ( 'NONE',  ( 10.99960280095051779, -9.919999999999998153, -0.09350563796401789585 ) ) ;
#120547=EDGE_CURVE ( 'NONE', #87461, #159016, #184995, .T. ) ;
#120563=B_SPLINE_CURVE_WITH_KNOTS ( 'NONE', 3,
 ( #182153, #197348, #147556, #183231, #84669, #33783, #98803, #213578 ),
 .UNSPECIFIED., .F., .F.,
 ( 4, 2, 2, 4 ),
 ( 4.982613841084584701E-18, 0.0002034531274099235997, 0.0004069062548198428084, 0.0008138125096396765096 ),
 .UNSPECIFIED. ) ;
#120604=CARTESIAN_POINT ( 'NONE',  ( -11.41267819554183127, 3.447199233515635619, 3.708203932499423150 ) ) ;
#120653=CIRCLE ( 'NONE', #151656, 0.2000000000000005107 ) ;
#120690=PRESENTATION_STYLE_ASSIGNMENT (( #55609 ) ) ;
#120729=CARTESIAN_POINT ( 'NONE',  ( 0.05425791151749740499, -7.744511198441856870, -9.500000000000131450 ) ) ;
#120731=DIRECTION ( 'NONE',  ( 0.6716942845482062330, -1.762391939599642519E-12, 0.7408284471490506062 ) ) ;
#120745=CARTESIAN_POINT ( 'NONE',  ( 8.596335327489152242E-14, -8.872104535001083647, -9.837524982414047159 ) ) ;
#120750=CARTESIAN_POINT ( 'NONE',  ( -10.39230484541323740, 4.000000000000003553, 6.000000000000048850 ) ) ;
#120755=AXIS2_PLACEMENT_3D ( 'NONE', #104516, #121904, #57885 ) ;
#120758=CARTESIAN_POINT ( 'NONE',  ( -10.99998664267163662, -6.472053282365751059, -0.02741317976723587138 ) ) ;
#120794=CARTESIAN_POINT ( 'NONE',  ( 0.2167848519283288866, -6.775781654326520353, 9.491250020638730689 ) ) ;
#120823=MECHANICAL_DESIGN_GEOMETRIC_PRESENTATION_REPRESENTATION('',(#82712),#162349);
#120931=CARTESIAN_POINT ( 'NONE',  ( -10.28586320583439395, 2.972657967447029037, 5.491880110203110732 ) ) ;
#120934=ORIENTED_EDGE ( 'NONE', *, *, #152831, .T. ) ;
#120950=CARTESIAN_POINT ( 'NONE',  ( -9.499606442108964544, -9.901472054505708442, 0.08647222121513538362 ) ) ;
#120951=CARTESIAN_POINT ( 'NONE',  ( 10.96287206819929594, -7.723179855898520962, -0.5577339983718512251 ) ) ;
#120974=B_SPLINE_CURVE_WITH_KNOTS ( 'NONE', 3,
 ( #149853, #5681, #35004, #54475, #67485, #118470, #121693, #100024 ),
 .UNSPECIFIED., .F., .F.,
 ( 4, 2, 2, 4 ),
 ( 0.000000000000000000, 0.0002185754043082790087, 0.0004371508086165580174, 0.0008743016172331179864 ),
 .UNSPECIFIED. ) ;
#121004=ORIENTED_EDGE ( 'NONE', *, *, #66712, .T. ) ;
#121012=VERTEX_POINT ( 'NONE', #86927 ) ;
#121013=MECHANICAL_DESIGN_GEOMETRIC_PRESENTATION_REPRESENTATION('',(#20712),#3393);
#121014=ADVANCED_FACE ( 'NONE', ( #125916 ), #167847, .T. ) ;
#121016=CARTESIAN_POINT ( 'NONE',  ( -10.91850271852025500, -9.971093637360025852, 0.1617895344457901952 ) ) ;
#121058=EDGE_LOOP ( 'NONE', ( #28692, #60210, #191306, #161473 ) ) ;
#121059=CARTESIAN_POINT ( 'NONE',  ( 9.499690612162391190, -9.919996481418243306, -0.07742489488623274796 ) ) ;
#121080=VERTEX_POINT ( 'NONE', #192946 ) ;
#121122=CARTESIAN_POINT ( 'NONE',  ( -10.99943592164173012, -9.900000000000019895, 0.1113975120799794716 ) ) ;
#121202=FILL_AREA_STYLE ('',( #123347 ) ) ;
#121203=DIRECTION ( 'NONE',  ( 0.000000000000000000, 0.000000000000000000, -1.000000000000000000 ) ) ;
#121218=CARTESIAN_POINT ( 'NONE',  ( -5.204170427930421283E-15, -6.796015482748915204, -10.25773349932950929 ) ) ;
#121230=CARTESIAN_POINT ( 'NONE',  ( -0.1062647697984078210, -6.683951901172095589, -9.488025208946956113 ) ) ;
#121297=CARTESIAN_POINT ( 'NONE',  ( 7.886602582589865129, -6.765616048178569208, -7.668547801473498460 ) ) ;
#121320=CARTESIAN_POINT ( 'NONE',  ( 0.000000000000000000, 3.799999999999998046, 6.249999999999995559 ) ) ;
#121340=CARTESIAN_POINT ( 'NONE',  ( -11.29689844398643572, -5.530538574611986391, 1.138412281109779656E-15 ) ) ;
#121366=( LENGTH_UNIT ( ) NAMED_UNIT ( * ) SI_UNIT ( .MILLI., .METRE. ) );
#121369=ORIENTED_EDGE ( 'NONE', *, *, #140872, .T. ) ;
#121377=CARTESIAN_POINT ( 'NONE',  ( -10.94445979172680694, -5.609732095436336330, 0.02903434592766030581 ) ) ;
#121419=STYLED_ITEM ( 'NONE', ( #92346 ), #85507 ) ;
#121444=CARTESIAN_POINT ( 'NONE',  ( -6.981856502303775969, -6.709867743870995049, 6.429544252029575802 ) ) ;
#121455=ORIENTED_EDGE ( 'NONE', *, *, #130804, .F. ) ;
#121466=ORIENTED_EDGE ( 'NONE', *, *, #126196, .F. ) ;
#121470=CARTESIAN_POINT ( 'NONE',  ( 2.493461049780987260, 3.507114751586604129, -11.73081193161139169 ) ) ;
#121503=DIRECTION ( 'NONE',  ( -0.000000000000000000, -1.000000000000000000, -0.000000000000000000 ) ) ;
#121515=AXIS2_PLACEMENT_3D ( 'NONE', #20435, #17226, #166708 ) ;
#121533=CARTESIAN_POINT ( 'NONE',  ( -7.586009164902065116, -6.657020681837092724, -7.796438949605414948 ) ) ;
#121557=VERTEX_POINT ( 'NONE', #41340 ) ;
#121583=CARTESIAN_POINT ( 'NONE',  ( 9.499606442108964544, -9.900000000000005684, -0.08647222121513538362 ) ) ;
#121593=CARTESIAN_POINT ( 'NONE',  ( 10.68054077891637377, -8.644755361503010604, -0.1864295327644151512 ) ) ;
#121602=CARTESIAN_POINT ( 'NONE',  ( 6.634380621478824125, -6.684699875907186062, 6.783773251375872171 ) ) ;
#121638=EDGE_CURVE ( 'NONE', #206352, #163559, #161058, .T. ) ;
#121671=AXIS2_PLACEMENT_3D ( 'NONE', #185413, #2376, #134583 ) ;
#121693=CARTESIAN_POINT ( 'NONE',  ( -0.06263693352612853538, -7.008128100062068988, 9.499802063084667125 ) ) ;
#121698=CARTESIAN_POINT ( 'NONE',  ( -5.126981680758313876E-15, -9.091017468556977121, 10.23550087314637302 ) ) ;
#121708=CARTESIAN_POINT ( 'NONE',  ( 0.03919461954074245080, -7.818966704647666965, -9.500338091956020747 ) ) ;
#121733=CONICAL_SURFACE ( 'NONE', #142394, 11.53746066217573940, 0.1181278931043537039 ) ;
#121771=CARTESIAN_POINT ( 'NONE',  ( -6.663994888585890841, -7.154544010626969985, 6.770610912236882939 ) ) ;
#121786=CARTESIAN_POINT ( 'NONE',  ( -0.09263662810812897663, -9.999999999999994671, -10.91955560153696148 ) ) ;
#121813=CARTESIAN_POINT ( 'NONE',  ( -10.45358220256320436, 1.000000000000000888, 5.892590188894342162 ) ) ;
#121821=CARTESIAN_POINT ( 'NONE',  ( -0.4635785636673758758, -6.836568542495036205, -10.85353573482950829 ) ) ;
#121837=ADVANCED_FACE ( 'NONE', ( #95429 ), #33026, .T. ) ;
#121850=ORIENTED_EDGE ( 'NONE', *, *, #110858, .F. ) ;
#121857=CARTESIAN_POINT ( 'NONE',  ( -6.500815856195037767, -6.554751173179672818, -6.901817412891865011 ) ) ;
#121878=CARTESIAN_POINT ( 'NONE',  ( -0.4655551865852154414, -8.176568542494919711, -9.512045263456256450 ) ) ;
#121904=DIRECTION ( 'NONE',  ( 0.000000000000000000, 0.000000000000000000, 1.000000000000000000 ) ) ;
#121910=ORIENTED_EDGE ( 'NONE', *, *, #53099, .T. ) ;
#121954=DIRECTION ( 'NONE',  ( 0.000000000000000000, -1.000000000000000000, 0.000000000000000000 ) ) ;
#121962=DIRECTION ( 'NONE',  ( 0.000000000000000000, 0.000000000000000000, 1.000000000000000000 ) ) ;
#121971=EDGE_CURVE ( 'NONE', #75305, #82411, #140637, .T. ) ;
#122020=CARTESIAN_POINT ( 'NONE',  ( 10.99861980075107581, -8.407420853759273172, -0.1919816227428499389 ) ) ;
#122042=DIRECTION ( 'NONE',  ( -0.000000000000000000, 1.000000000000000000, -0.000000000000000000 ) ) ;
#122059=CARTESIAN_POINT ( 'NONE',  ( 1.897353801849633006E-16, -6.452016312669676346, -11.25751254361623843 ) ) ;
#122091=FILL_AREA_STYLE ('',( #158775 ) ) ;
#122114=CARTESIAN_POINT ( 'NONE',  ( 9.486581398170528701, -9.006862915010220405, -0.5116190538792210196 ) ) ;
#122125=CARTESIAN_POINT ( 'NONE',  ( -5.204170427930421283E-15, 3.499999999999989342, -11.99999999999997868 ) ) ;
#122128=ORIENTED_EDGE ( 'NONE', *, *, #205728, .T. ) ;
#122189=( GEOMETRIC_REPRESENTATION_CONTEXT ( 3 ) GLOBAL_UNCERTAINTY_ASSIGNED_CONTEXT ( ( #25927 ) ) GLOBAL_UNIT_ASSIGNED_CONTEXT ( ( #94783, #95855, #12423 ) ) REPRESENTATION_CONTEXT ( 'NONE', 'WORKASPACE' ) );
#122194=ORIENTED_EDGE ( 'NONE', *, *, #134348, .F. ) ;
#122208=AXIS2_PLACEMENT_3D ( 'NONE', #139265, #207440, #124159 ) ;
#122221=( GEOMETRIC_REPRESENTATION_CONTEXT ( 3 ) GLOBAL_UNCERTAINTY_ASSIGNED_CONTEXT ( ( #132872 ) ) GLOBAL_UNIT_ASSIGNED_CONTEXT ( ( #140026, #21939, #123843 ) ) REPRESENTATION_CONTEXT ( 'NONE', 'WORKASPACE' ) );
#122260=CARTESIAN_POINT ( 'NONE',  ( 0.3869524901765013514, 1.970899860167981910, -11.77270853017065200 ) ) ;
#122267=( BOUNDED_SURFACE ( )  B_SPLINE_SURFACE ( 3, 2, ( 
 ( #186468, #7710, #38103 ),
 ( #56485, #19702, #20753 ),
 ( #85781, #103102, #169160 ),
 ( #86848, #4491, #21808 ) ),
 .UNSPECIFIED., .F., .F., .T. ) 
 B_SPLINE_SURFACE_WITH_KNOTS ( ( 4, 4 ),
 ( 3, 3 ),
 ( 0.01133669335851669041, 0.01377857026255017818 ),
 ( 0.000000000000000000, 1.000000000000000000 ),
 .UNSPECIFIED. ) 
 GEOMETRIC_REPRESENTATION_ITEM ( )  RATIONAL_B_SPLINE_SURFACE ( (
 ( 1.000000000000000000, 0.7169883299103929630, 1.000000000000000000),
 ( 1.000000000000000000, 0.7174882367753923074, 1.000000000000000000),
 ( 1.000000000000000000, 0.7180609655871061925, 1.000000000000000000),
 ( 1.000000000000000000, 0.7187540731122933346, 1.000000000000000000) ) ) 
 REPRESENTATION_ITEM ( '' )  SURFACE ( )  );
#122277=CARTESIAN_POINT ( 'NONE',  ( 10.91877977293360047, -9.985078020775006280, -0.1443118549625480029 ) ) ;
#122295=DIRECTION ( 'NONE',  ( 0.000000000000000000, 1.000000000000000000, 0.000000000000000000 ) ) ;
#122317=CARTESIAN_POINT ( 'NONE',  ( -7.949604103952364831, -6.836271202499947464, 7.404765023120916112 ) ) ;
#122328=DIRECTION ( 'NONE',  ( 0.000000000000000000, -0.000000000000000000, 1.000000000000000000 ) ) ;
#122337=ADVANCED_FACE ( 'NONE', ( #174925 ), #212977, .T. ) ;
#122342=ORIENTED_EDGE ( 'NONE', *, *, #148379, .T. ) ;
#122362=CIRCLE ( 'NONE', #153346, 9.523431457505068920 ) ;
#122364=PRESENTATION_STYLE_ASSIGNMENT (( #23684 ) ) ;
#122387=CARTESIAN_POINT ( 'NONE',  ( -9.479415819240319507, -6.570271182191716797, 0.2417854191286431531 ) ) ;
#122409=EDGE_LOOP ( 'NONE', ( #69919, #114856, #84782, #198444 ) ) ;
#122447=DIRECTION ( 'NONE',  ( 0.000000000000000000, 0.000000000000000000, 1.000000000000000000 ) ) ;
#122525=ORIENTED_EDGE ( 'NONE', *, *, #168972, .T. ) ;
#122555=CARTESIAN_POINT ( 'NONE',  ( 10.39230484541330313, 3.499999999999989342, 5.999999999999906741 ) ) ;
#122565=CARTESIAN_POINT ( 'NONE',  ( -8.024185963717894055, -5.166862990899638852, 7.524604700374177391 ) ) ;
#122579=DIRECTION ( 'NONE',  ( 0.000000000000000000, 0.000000000000000000, -1.000000000000000000 ) ) ;
#122581=CARTESIAN_POINT ( 'NONE',  ( 9.516228778038653857, -8.176227079964613509, -0.3870642018030908682 ) ) ;
#122586=DIRECTION ( 'NONE',  ( 0.000000000000000000, -1.000000000000000000, 0.000000000000000000 ) ) ;
#122609=CARTESIAN_POINT ( 'NONE',  ( -7.626802973668077357, -6.615717645447081630, -7.927630635717592078 ) ) ;
#122643=CARTESIAN_POINT ( 'NONE',  ( 2.039928227386953008, 3.162178953954597471, -11.45750328113830108 ) ) ;
#122645=CARTESIAN_POINT ( 'NONE',  ( 9.499700864329909678, -7.154544010627095219, 0.07538891330675402680 ) ) ;
#122653=CARTESIAN_POINT ( 'NONE',  ( -8.023115266309158500, -5.166862915010145052, 7.407835137441773021 ) ) ;
#122684=CARTESIAN_POINT ( 'NONE',  ( 0.2883962233416060283, -9.094943692057521289, -9.630124952822544770 ) ) ;
#122707=VECTOR ( 'NONE', #53699, 1000.000000000000000 ) ;
#122722=AXIS2_PLACEMENT_3D ( 'NONE', #164113, #11438, #195545 ) ;
#122755=EDGE_CURVE ( 'NONE', #58812, #1871, #109318, .T. ) ;
#122813=AXIS2_PLACEMENT_3D ( 'NONE', #34478, #52870, #200165 ) ;
#122828=CARTESIAN_POINT ( 'NONE',  ( 7.253312916980332758, -6.796015482748900105, 7.253312916980308778 ) ) ;
#122848=FILL_AREA_STYLE_COLOUR ( '', #98091 ) ;
#122857=CARTESIAN_POINT ( 'NONE',  ( -6.661184041420952440, -7.246166700180828535, 6.773376349083141790 ) ) ;
#122897=CARTESIAN_POINT ( 'NONE',  ( 10.91804381884011121, -9.954640477432047163, -0.1905751637469971504 ) ) ;
#122907=CARTESIAN_POINT ( 'NONE',  ( -0.1888596022590736112, -6.708723052947947352, -10.87247189006428272 ) ) ;
#122938=CARTESIAN_POINT ( 'NONE',  ( 7.786489011997303145, -5.767087321559190016, 7.770158002572460809 ) ) ;
#122955=TOROIDAL_SURFACE ( 'NONE', #29489, 9.580000000000001847, 0.08000000000000000167 ) ;
#122979=DIRECTION ( 'NONE',  ( 0.000000000000000000, -1.000000000000000000, 0.000000000000000000 ) ) ;
#122997=ORIENTED_EDGE ( 'NONE', *, *, #153215, .F. ) ;
#123001=EDGE_CURVE ( 'NONE', #207703, #162811, #103248, .T. ) ;
#123071=CARTESIAN_POINT ( 'NONE',  ( -0.09005296632882617280, -9.916958724994124452, -10.99963137851696082 ) ) ;
#123083=DIRECTION ( 'NONE',  ( 0.000000000000000000, 0.06195440338563660415, 0.9980789807931683688 ) ) ;
#123106=CARTESIAN_POINT ( 'NONE',  ( -9.499615238232420822, -9.906571760739462107, 0.08550182772145856203 ) ) ;
#123144=ADVANCED_FACE ( 'NONE', ( #98990 ), #143920, .T. ) ;
#123153=CARTESIAN_POINT ( 'NONE',  ( 0.000000000000000000, 1.000000000000000888, -11.49999999999998934 ) ) ;
#123159=ORIENTED_EDGE ( 'NONE', *, *, #127553, .F. ) ;
#123169=CARTESIAN_POINT ( 'NONE',  ( -10.45358220256320436, 1.000000000000000888, 5.892590188894342162 ) ) ;
#123171=DIRECTION ( 'NONE',  ( 0.000000000000000000, 0.000000000000000000, -1.000000000000000000 ) ) ;
#123174=( NAMED_UNIT ( * ) PLANE_ANGLE_UNIT ( ) SI_UNIT ( $, .RADIAN. ) );
#123205=CARTESIAN_POINT ( 'NONE',  ( 0.07999999999999327094, -8.407420853759283830, 10.99970695577496294 ) ) ;
#123234=CARTESIAN_POINT ( 'NONE',  ( -6.781144757626059061, -7.161464053357560644, 6.776370306708066948 ) ) ;
#123257=VERTEX_POINT ( 'NONE', #17695 ) ;
#123265=AXIS2_PLACEMENT_3D ( 'NONE', #68913, #150209, #182680 ) ;
#123270=( GEOMETRIC_REPRESENTATION_CONTEXT ( 3 ) GLOBAL_UNCERTAINTY_ASSIGNED_CONTEXT ( ( #886 ) ) GLOBAL_UNIT_ASSIGNED_CONTEXT ( ( #29913, #16816, #211832 ) ) REPRESENTATION_CONTEXT ( 'NONE', 'WORKASPACE' ) );
#123302=DIRECTION ( 'NONE',  ( 0.000000000000000000, 0.000000000000000000, -1.000000000000000000 ) ) ;
#123340=CARTESIAN_POINT ( 'NONE',  ( 9.495347311156807635, -6.857257212219900921, -1.861063089699362494E-15 ) ) ;
#123347=FILL_AREA_STYLE_COLOUR ( '', #27315 ) ;
#123384=( NAMED_UNIT ( * ) SI_UNIT ( $, .STERADIAN. ) SOLID_ANGLE_UNIT ( ) );
#123407=CARTESIAN_POINT ( 'NONE',  ( -10.91970695577495754, -5.907420853759267843, -0.07999999999999847511 ) ) ;
#123446=CARTESIAN_POINT ( 'NONE',  ( 7.985752187169497418, -6.863172033215938050, -7.565242077046494096 ) ) ;
#123462=CARTESIAN_POINT ( 'NONE',  ( -3.672734859294646270E-15, -9.746166700180790343, -9.579665964948869572 ) ) ;
#123473=SURFACE_STYLE_USAGE ( .BOTH. , #173210 ) ;
#123480=CARTESIAN_POINT ( 'NONE',  ( -6.725651841507101381, -7.791858861492833910, 6.710064404886642464 ) ) ;
#123503=CARTESIAN_POINT ( 'NONE',  ( 0.000000000000000000, 0.03624871340549007392, 6.250000000000000000 ) ) ;
#123515=CYLINDRICAL_SURFACE ( 'NONE', #162134, 0.07999999999999993228 ) ;
#123542=CARTESIAN_POINT ( 'NONE',  ( -9.920930332858638678, -7.768188185258915190, 0.4648879685169945430 ) ) ;
#123551=ORIENTED_EDGE ( 'NONE', *, *, #175718, .T. ) ;
#123568=ORIENTED_EDGE ( 'NONE', *, *, #202457, .F. ) ;
#123631=CARTESIAN_POINT ( 'NONE',  ( -0.04765083308772119497, -6.900199406649610623, -9.605391220871888791 ) ) ;
#123666=EDGE_LOOP ( 'NONE', ( #40534, #189743, #160496, #163807, #123159 ) ) ;
#123676=ORIENTED_EDGE ( 'NONE', *, *, #182811, .F. ) ;
#123701=ORIENTED_EDGE ( 'NONE', *, *, #65889, .F. ) ;
#123706=DIRECTION ( 'NONE',  ( 0.000000000000000000, 1.000000000000000000, 0.000000000000000000 ) ) ;
#123729=DIRECTION ( 'NONE',  ( 0.000000000000000000, 1.000000000000000000, 0.000000000000000000 ) ) ;
#123813=ORIENTED_EDGE ( 'NONE', *, *, #166279, .F. ) ;
#123843=( NAMED_UNIT ( * ) SI_UNIT ( $, .STERADIAN. ) SOLID_ANGLE_UNIT ( ) );
#123958=FACE_OUTER_BOUND ( 'NONE', #46101, .T. ) ;
#123965=ORIENTED_EDGE ( 'NONE', *, *, #164350, .T. ) ;
#123997=DIRECTION ( 'NONE',  ( 1.224646799147353207E-16, 0.000000000000000000, -1.000000000000000000 ) ) ;
#124008=CARTESIAN_POINT ( 'NONE',  ( -0.01979922387982912396, -6.863887327018224127, 9.496663239505998888 ) ) ;
#124016=VECTOR ( 'NONE', #17227, 1000.000000000000000 ) ;
#124042=CARTESIAN_POINT ( 'NONE',  ( 0.000000000000000000, 7.849261790823902629, 10.24999999999998934 ) ) ;
#124055=ORIENTED_EDGE ( 'NONE', *, *, #166016, .T. ) ;
#124131=ORIENTED_EDGE ( 'NONE', *, *, #36008, .T. ) ;
#124138=DIRECTION ( 'NONE',  ( 0.000000000000000000, -1.000000000000000000, 0.000000000000000000 ) ) ;
#124159=DIRECTION ( 'NONE',  ( 0.000000000000000000, 0.000000000000000000, 1.000000000000000000 ) ) ;
#124160=CARTESIAN_POINT ( 'NONE',  ( -8.581735480930626505E-14, -9.900000000000005684, -11.00029519899099739 ) ) ;
#124175=MECHANICAL_DESIGN_GEOMETRIC_PRESENTATION_REPRESENTATION('',(#92881),#182816);
#124204=CARTESIAN_POINT ( 'NONE',  ( -6.662120174140259365, -7.184999792969698262, 6.772456105771886392 ) ) ;
#124205=EDGE_CURVE ( 'NONE', #142909, #159583, #68039, .T. ) ;
#124254=CARTESIAN_POINT ( 'NONE',  ( 0.04006801626470013478, -6.479296433800355359, -11.00029612940780410 ) ) ;
#124268=CARTESIAN_POINT ( 'NONE',  ( 9.499606442108968096, -9.900000000000019895, -0.08647222121521722094 ) ) ;
#124293=CARTESIAN_POINT ( 'NONE',  ( 10.34804403480040236, -6.705807696128828432, 9.269928574751062911E-15 ) ) ;
#124301=ORIENTED_EDGE ( 'NONE', *, *, #143273, .T. ) ;
#124325=CARTESIAN_POINT ( 'NONE',  ( 0.07804503809599044883, -9.997560133496188328, 10.91958144425262311 ) ) ;
#124333=EDGE_CURVE ( 'NONE', #66793, #89199, #118522, .T. ) ;
#124338=EDGE_CURVE ( 'NONE', #51191, #82895, #124939, .T. ) ;
#124349=CARTESIAN_POINT ( 'NONE',  ( -0.07801928546529091069, -7.184999792974072541, 9.499679989893808241 ) ) ;
#124390=( NAMED_UNIT ( * ) SI_UNIT ( $, .STERADIAN. ) SOLID_ANGLE_UNIT ( ) );
#124400=CARTESIAN_POINT ( 'NONE',  ( -10.99036836684472540, -7.696788179137225683, 0.4651914231089842033 ) ) ;
#124407=DIRECTION ( 'NONE',  ( 0.000000000000000000, -1.000000000000000000, 0.000000000000000000 ) ) ;
#124420=CIRCLE ( 'NONE', #30959, 0.08000000000000018208 ) ;
#124443=EDGE_CURVE ( 'NONE', #125480, #31312, #191962, .T. ) ;
#124473=ORIENTED_EDGE ( 'NONE', *, *, #48815, .F. ) ;
#124487=FACE_OUTER_BOUND ( 'NONE', #176274, .T. ) ;
#124488=FILL_AREA_STYLE ('',( #87636 ) ) ;
#124502=CARTESIAN_POINT ( 'NONE',  ( 8.074422843257124782, -6.701288531902056533, -7.470306724222344208 ) ) ;
#124517=FACE_OUTER_BOUND ( 'NONE', #114229, .T. ) ;
#124520=( BOUNDED_SURFACE ( )  B_SPLINE_SURFACE ( 3, 2, ( 
 ( #161010, #49390, #99211 ),
 ( #585, #112325, #47283 ),
 ( #145863, #195647, #165260 ),
 ( #113395, #80827, #82936 ) ),
 .UNSPECIFIED., .F., .F., .T. ) 
 B_SPLINE_SURFACE_WITH_KNOTS ( ( 4, 4 ),
 ( 3, 3 ),
 ( 0.01127358803094579559, 0.01374177962974961961 ),
 ( 0.000000000000000000, 1.000000000000000000 ),
 .UNSPECIFIED. ) 
 GEOMETRIC_REPRESENTATION_ITEM ( )  RATIONAL_B_SPLINE_SURFACE ( (
 ( 1.000000000000000000, 0.6947640035331676955, 1.000000000000000000),
 ( 1.000000000000000000, 0.6955505939615566069, 1.000000000000000000),
 ( 1.000000000000000000, 0.6961913616428424545, 1.000000000000000000),
 ( 1.000000000000000000, 0.6967468848049996888, 1.000000000000000000) ) ) 
 REPRESENTATION_ITEM ( '' )  SURFACE ( )  );
#124572=CARTESIAN_POINT ( 'NONE',  ( -10.91970695577495398, -9.999999999999994671, -0.07999999999999153621 ) ) ;
#124591=ORIENTED_EDGE ( 'NONE', *, *, #14312, .T. ) ;
#124618=CARTESIAN_POINT ( 'NONE',  ( 8.023115266309142513, -5.166862915010145052, -7.407835137441765916 ) ) ;
#124627=CARTESIAN_POINT ( 'NONE',  ( -0.1653080603930669190, -5.324706741106404628, -10.99896775280364025 ) ) ;
#124639=CARTESIAN_POINT ( 'NONE',  ( -6.776323704810612192, -7.189630408300039299, -6.777912011469588549 ) ) ;
#124677=CARTESIAN_POINT ( 'NONE',  ( -10.91970695577495931, -6.134628647623513231, 0.000000000000000000 ) ) ;
#124713=B_SPLINE_CURVE_WITH_KNOTS ( 'NONE', 3,
 ( #141978, #93218, #27109, #146232, #30332, #212249, #143049 ),
 .UNSPECIFIED., .F., .F.,
 ( 4, 3, 4 ),
 ( 0.0001135037246152898908, 0.0006245292469112882598, 0.002007692286193825740 ),
 .UNSPECIFIED. ) ;
#124718=CARTESIAN_POINT ( 'NONE',  ( 0.04570195657714280074, 1.813436143228261743, -11.99992749206847975 ) ) ;
#124727=EDGE_CURVE ( 'NONE', #45587, #55041, #2059, .T. ) ;
#124731=CARTESIAN_POINT ( 'NONE',  ( -8.072398248062487625, -5.212532583863426439, 7.453913518772579572 ) ) ;
#124760=ORIENTED_EDGE ( 'NONE', *, *, #46509, .T. ) ;
#124771=ORIENTED_EDGE ( 'NONE', *, *, #162539, .T. ) ;
#124776=CARTESIAN_POINT ( 'NONE',  ( -10.96287206819832605, -7.723179855899500623, 0.5577339983718334615 ) ) ;
#124811=CARTESIAN_POINT ( 'NONE',  ( 10.99968117833243042, -6.698521824825881765, -0.09510031644102620585 ) ) ;
#124833=CARTESIAN_POINT ( 'NONE',  ( -7.661067326845563130, -5.325441678136415113, -7.893838479094846150 ) ) ;
#124877=B_SPLINE_CURVE_WITH_KNOTS ( 'NONE', 3,
 ( #73084, #90439, #106729, #141358 ),
 .UNSPECIFIED., .F., .F.,
 ( 4, 4 ),
 ( 1.113895128243735996E-15, 8.505390839970735750E-05 ),
 .UNSPECIFIED. ) ;
#124896=DIRECTION ( 'NONE',  ( 0.000000000000000000, 0.000000000000000000, 1.000000000000000000 ) ) ;
#124903=ORIENTED_EDGE ( 'NONE', *, *, #39920, .T. ) ;
#124918=CIRCLE ( 'NONE', #183727, 11.99999999999999112 ) ;
#124939=B_SPLINE_CURVE_WITH_KNOTS ( 'NONE', 3,
 ( #201811, #101127, #17725, #2539, #185576, #184507, #103280, #36125 ),
 .UNSPECIFIED., .F., .F.,
 ( 4, 2, 2, 4 ),
 ( 0.000000000000000000, 0.0004365159022975833875, 0.0006547738534463757318, 0.0008730318045951679677 ),
 .UNSPECIFIED. ) ;
#124958=( LENGTH_UNIT ( ) NAMED_UNIT ( * ) SI_UNIT ( .MILLI., .METRE. ) );
#124965=SURFACE_STYLE_FILL_AREA ( #8989 ) ;
#124996=PRODUCT_DEFINITION_SHAPE ( 'NONE', 'NONE',  #135165 ) ;
#125016=CARTESIAN_POINT ( 'NONE',  ( 10.99861993420630135, -9.955063214563365293, -0.1919715503784026334 ) ) ;
#125036=CARTESIAN_POINT ( 'NONE',  ( -10.25877837909746937, 3.235871879154613051, 5.476282928277060869 ) ) ;
#125049=ORIENTED_EDGE ( 'NONE', *, *, #41997, .F. ) ;
#125054=ORIENTED_EDGE ( 'NONE', *, *, #206395, .T. ) ;
#125086=CARTESIAN_POINT ( 'NONE',  ( 0.08359363160202464005, -9.910747646673584654, 10.99968245379461607 ) ) ;
#125193=DIRECTION ( 'NONE',  ( 0.000000000000000000, 0.000000000000000000, 1.000000000000000000 ) ) ;
#125204=ORIENTED_EDGE ( 'NONE', *, *, #15332, .T. ) ;
#125218=DIRECTION ( 'NONE',  ( 5.551115123125783935E-17, 0.7071067811865536790, -0.7071067811865413555 ) ) ;
#125238=CARTESIAN_POINT ( 'NONE',  ( 11.35993080936262345, 3.555461883994698979, -3.691065267805079042 ) ) ;
#125272=ORIENTED_EDGE ( 'NONE', *, *, #115265, .F. ) ;
#125304=VERTEX_POINT ( 'NONE', #78273 ) ;
#125349=CARTESIAN_POINT ( 'NONE',  ( -7.055786748303249922, -6.583711766989059910, 6.534012848836718845 ) ) ;
#125380=CARTESIAN_POINT ( 'NONE',  ( 0.02890330888917177696, -9.971207602185762298, 10.91966316483287613 ) ) ;
#125409=CIRCLE ( 'NONE', #163367, 11.89429233241351902 ) ;
#125431=ADVANCED_FACE ( 'NONE', ( #110845 ), #139921, .F. ) ;
#125447=CARTESIAN_POINT ( 'NONE',  ( -6.828399852920244761, -6.891066458783222437, 6.756361134959175452 ) ) ;
#125459=CARTESIAN_POINT ( 'NONE',  ( -9.488641820551103834, -8.200000000000001066, 0.4644097342743105372 ) ) ;
#125480=VERTEX_POINT ( 'NONE', #52181 ) ;
#125505=SURFACE_STYLE_USAGE ( .BOTH. , #157940 ) ;
#125508=CARTESIAN_POINT ( 'NONE',  ( -0.2972806740312780582, -7.751137252134800093, 10.97067717498812200 ) ) ;
#125524=CIRCLE ( 'NONE', #132443, 10.99999999999999112 ) ;
#125572=CARTESIAN_POINT ( 'NONE',  ( 9.536979704252619428, -7.995840219786838787, -0.1489494290324772929 ) ) ;
#125576=CARTESIAN_POINT ( 'NONE',  ( 0.1817359287054975125, -9.181675805132181623, -9.625413980971190497 ) ) ;
#125578=CARTESIAN_POINT ( 'NONE',  ( -7.721398836998378812, -6.134628647623499909, 7.721398836998403681 ) ) ;
#125580=AXIS2_PLACEMENT_3D ( 'NONE', #153923, #108434, #5492 ) ;
#125589=( NAMED_UNIT ( * ) PLANE_ANGLE_UNIT ( ) SI_UNIT ( $, .RADIAN. ) );
#125597=CARTESIAN_POINT ( 'NONE',  ( -6.661184041420952440, -7.473374494058216300, 6.773376349083141790 ) ) ;
#125620=CARTESIAN_POINT ( 'NONE',  ( 6.604641253243924481, -6.414086731524403007, 7.221001870987142190 ) ) ;
#125680=CARTESIAN_POINT ( 'NONE',  ( 9.499668754385636404, -7.473374494045003757, 0.07933194154488391880 ) ) ;
#125686=CARTESIAN_POINT ( 'NONE',  ( -8.879134602965971013, 3.426985321572576737, -7.474367077670519777 ) ) ;
#125699=EDGE_CURVE ( 'NONE', #159480, #99453, #2212, .T. ) ;
#125700=CARTESIAN_POINT ( 'NONE',  ( -0.3869524901764175295, 1.970899860167975914, 11.77270853017065377 ) ) ;
#125717=ORIENTED_EDGE ( 'NONE', *, *, #78734, .T. ) ;
#125737=DIRECTION ( 'NONE',  ( 0.000000000000000000, 0.000000000000000000, -1.000000000000000000 ) ) ;
#125749=CARTESIAN_POINT ( 'NONE',  ( -0.4355862708379995563, -6.583980363595115293, -9.606148981167580203 ) ) ;
#125793=CARTESIAN_POINT ( 'NONE',  ( -6.956180625285975694, -6.372104534813817445, 6.956180625285645291 ) ) ;
#125805=CARTESIAN_POINT ( 'NONE',  ( 7.439168848973994663, -6.893137084989842123, 8.103009739378013165 ) ) ;
#125827=CARTESIAN_POINT ( 'NONE',  ( -7.834948825496944380, -6.307829212974244371, -7.720982897393569466 ) ) ;
#125841=CARTESIAN_POINT ( 'NONE',  ( -10.96381302404150482, -7.750949308401941629, 0.4891431138945980250 ) ) ;
#125852=CARTESIAN_POINT ( 'NONE',  ( -10.99943592164173012, -9.901472394401615418, 0.1113975120799921142 ) ) ;
#125879=CARTESIAN_POINT ( 'NONE',  ( 10.99970480893081692, -6.134628647623513231, 0.08058608058608254798 ) ) ;
#125900=ORIENTED_EDGE ( 'NONE', *, *, #135617, .T. ) ;
#125904=LINE ( 'NONE', #8856, #139592 ) ;
#125909=ORIENTED_EDGE ( 'NONE', *, *, #60148, .F. ) ;
#125916=FACE_OUTER_BOUND ( 'NONE', #72246, .T. ) ;
#125936=EDGE_LOOP ( 'NONE', ( #16675, #45810, #124771, #23859, #102381, #142215, #19286, #129191 ) ) ;
#125993=CARTESIAN_POINT ( 'NONE',  ( -0.07602376731355095507, -7.154544010627095219, 9.579698345292692707 ) ) ;
#126047=DIRECTION ( 'NONE',  ( -0.7366372490351829061, 1.218064704987765655E-12, 0.6762880771785629852 ) ) ;
#126050=ORIENTED_EDGE ( 'NONE', *, *, #36008, .F. ) ;
#126057=CARTESIAN_POINT ( 'NONE',  ( 7.724608556409205740, -5.759585062615360407, 7.735357998705606697 ) ) ;
#126069=EDGE_CURVE ( 'NONE', #156791, #193127, #23934, .T. ) ;
#126081=CARTESIAN_POINT ( 'NONE',  ( 0.2442642247113699094, -5.209160580580716626, 10.99754090108938342 ) ) ;
#126097=AXIS2_PLACEMENT_3D ( 'NONE', #135263, #203407, #71276 ) ;
#126111=CARTESIAN_POINT ( 'NONE',  ( 9.469892045836674654, -6.532648833121171172, -0.4294077647110511320 ) ) ;
#126123=CARTESIAN_POINT ( 'NONE',  ( 7.624693973552425952, -5.341768514962141445, 7.882977371602010841 ) ) ;
#126146=CARTESIAN_POINT ( 'NONE',  ( 0.09196683552161016850, -9.918146503183461249, 10.99961570984664583 ) ) ;
#126186=EDGE_CURVE ( 'NONE', #26009, #74902, #209980, .T. ) ;
#126189=AXIS2_PLACEMENT_3D ( 'NONE', #126954, #192913, #40289 ) ;
#126196=EDGE_CURVE ( 'NONE', #144319, #150870, #119533, .T. ) ;
#126198=CARTESIAN_POINT ( 'NONE',  ( -2.400879090975684971, 3.975933801733733564, 11.29524806062143760 ) ) ;
#126261=AXIS2_PLACEMENT_3D ( 'NONE', #181408, #78578, #99112 ) ;
#126320=CARTESIAN_POINT ( 'NONE',  ( 10.43625799253445408, 3.019799309333367265, -6.025376361322313024 ) ) ;
#126380=CARTESIAN_POINT ( 'NONE',  ( -0.03415196713899504993, -6.453216945989382225, -10.89423718502886373 ) ) ;
#126396=MECHANICAL_DESIGN_GEOMETRIC_PRESENTATION_REPRESENTATION('',(#105616),#212733);
#126418=CARTESIAN_POINT ( 'NONE',  ( 9.501690547401153708, -8.186910008819950235, -0.4655726814551008896 ) ) ;
#126425=ORIENTED_EDGE ( 'NONE', *, *, #169231, .T. ) ;
#126499=CARTESIAN_POINT ( 'NONE',  ( 10.88266508516665532, 3.691791674785631194, -3.942622913914296312 ) ) ;
#126529=DIRECTION ( 'NONE',  ( -0.04520447523801534445, 0.000000000000000000, 0.9989777552170296948 ) ) ;
#126546=ORIENTED_EDGE ( 'NONE', *, *, #43966, .T. ) ;
#126547=CIRCLE ( 'NONE', #60739, 0.07999999999999907185 ) ;
#126573=DIRECTION ( 'NONE',  ( -0.9988044021632734859, 0.000000000000000000, 0.04888523518676873847 ) ) ;
#126610=CARTESIAN_POINT ( 'NONE',  ( 0.4635785636673654952, -6.836568542495036205, 10.85353573482952250 ) ) ;
#126622=EDGE_LOOP ( 'NONE', ( #197732, #186269, #146430, #99136, #141572 ) ) ;
#126633=CARTESIAN_POINT ( 'NONE',  ( 9.512045263456261779, -8.176568542494926817, -0.4655551865852028404 ) ) ;
#126677=EDGE_CURVE ( 'NONE', #130349, #15288, #106201, .T. ) ;
#126684=CARTESIAN_POINT ( 'NONE',  ( 6.661184041420940005, -7.473374494058216300, -6.773376349083132908 ) ) ;
#126701=ORIENTED_EDGE ( 'NONE', *, *, #4201, .F. ) ;
#126709=CIRCLE ( 'NONE', #60922, 0.08000000000000001554 ) ;
#126742=( NAMED_UNIT ( * ) SI_UNIT ( $, .STERADIAN. ) SOLID_ANGLE_UNIT ( ) );
#126744=CARTESIAN_POINT ( 'NONE',  ( -2.494940289813118994, 3.038492715500545227, 11.73777120880565583 ) ) ;
#126752=CARTESIAN_POINT ( 'NONE',  ( -0.1376292675369459595, -5.401429653175759071, -10.96107445065240249 ) ) ;
#126778=CIRCLE ( 'NONE', #195796, 10.97656854249491509 ) ;
#126875=CIRCLE ( 'NONE', #16045, 0.07999999999999993228 ) ;
#126896=LINE ( 'NONE', #192853, #200218 ) ;
#126897=CARTESIAN_POINT ( 'NONE',  ( 6.849430810391395674, -7.996947095390812166, -6.637758778446690933 ) ) ;
#126909=CARTESIAN_POINT ( 'NONE',  ( -10.98194350564911481, -7.699999999999996625, 0.6300133639306312316 ) ) ;
#126917=CARTESIAN_POINT ( 'NONE',  ( 6.830415307812257808, 7.849261790823902629, 6.717278222822394618 ) ) ;
#126920=CARTESIAN_POINT ( 'NONE',  ( 0.000000000000000000, 3.799999999999998046, 6.249999999999995559 ) ) ;
#126934=EDGE_LOOP ( 'NONE', ( #99793, #197426, #28183, #191077, #205737 ) ) ;
#126943=CARTESIAN_POINT ( 'NONE',  ( -7.523999700038797478, -5.166862915010145940, -8.024744567526228778 ) ) ;
#126954=CARTESIAN_POINT ( 'NONE',  ( 0.000000000000000000, 1.000000000000000888, 0.000000000000000000 ) ) ;
#126974=CARTESIAN_POINT ( 'NONE',  ( -7.547231044119362409, -5.251137252134767230, -7.967649405165816212 ) ) ;
#127002=CIRCLE ( 'NONE', #137286, 6.249999999999995559 ) ;
#127008=CARTESIAN_POINT ( 'NONE',  ( 6.663994888585877518, -7.154544010627095219, -6.770610912236881163 ) ) ;
#127031=EDGE_CURVE ( 'NONE', #8301, #75305, #213275, .T. ) ;
#127032=DIRECTION ( 'NONE',  ( 0.000000000000000000, 0.000000000000000000, 1.000000000000000000 ) ) ;
#127072=ORIENTED_EDGE ( 'NONE', *, *, #129019, .F. ) ;
#127089=VERTEX_POINT ( 'NONE', #68613 ) ;
#127131=CARTESIAN_POINT ( 'NONE',  ( 9.796090618744123901, 3.974415841077565403, 6.102288299938424920 ) ) ;
#127164=ORIENTED_EDGE ( 'NONE', *, *, #163961, .F. ) ;
#127172=CARTESIAN_POINT ( 'NONE',  ( -10.18461545817740088, 3.956598013261175772, 5.433575010662861082 ) ) ;
#127215=CARTESIAN_POINT ( 'NONE',  ( 7.362820735712270803, -5.796536394785693602, -7.362820735712300113 ) ) ;
#127235=ADVANCED_FACE ( 'NONE', ( #119592, #170398 ), #54527, .T. ) ;
#127248=CARTESIAN_POINT ( 'NONE',  ( 7.863746947443975621, -5.507058666270990166, -7.245729715095582613 ) ) ;
#127267=CIRCLE ( 'NONE', #154856, 11.29999999999998828 ) ;
#127395=DIRECTION ( 'NONE',  ( 0.000000000000000000, 0.000000000000000000, -1.000000000000000000 ) ) ;
#127420=EDGE_CURVE ( 'NONE', #109058, #168888, #165885, .T. ) ;
#127438=CARTESIAN_POINT ( 'NONE',  ( 1.347111479062088799E-15, 0.000000000000000000, -11.00000000000000178 ) ) ;
#127456=CARTESIAN_POINT ( 'NONE',  ( -0.3891817118476354476, -6.836286050427575312, -10.85699613887067549 ) ) ;
#127474=DIRECTION ( 'NONE',  ( 0.000000000000000000, 1.000000000000000000, 0.000000000000000000 ) ) ;
#127499=CARTESIAN_POINT ( 'NONE',  ( -8.064677165291197269, -5.223431457505076203, 7.446209719563364082 ) ) ;
#127503=CARTESIAN_POINT ( 'NONE',  ( -8.966533317356066846, 1.405705671057797757, -7.975201661134190267 ) ) ;
#127519=CIRCLE ( 'NONE', #169005, 6.449999999999992184 ) ;
#127529=ORIENTED_EDGE ( 'NONE', *, *, #152899, .T. ) ;
#127553=EDGE_CURVE ( 'NONE', #121557, #41100, #157968, .T. ) ;
#127554=UNCERTAINTY_MEASURE_WITH_UNIT (LENGTH_MEASURE( 1.000000000000000082E-05 ), #74308, 'distance_accuracy_value', 'NONE');
#127555=DIRECTION ( 'NONE',  ( 0.000000000000000000, 0.000000000000000000, -1.000000000000000000 ) ) ;
#127579=CARTESIAN_POINT ( 'NONE',  ( -10.91944002402978775, -9.900000000000005684, 0.1105873483556694958 ) ) ;
#127622=CARTESIAN_POINT ( 'NONE',  ( -10.09384670630917746, -7.616807780223579627, 1.138412281109779656E-15 ) ) ;
#127656=CARTESIAN_POINT ( 'NONE',  ( -0.007601003541780289308, -8.259585062615352413, 10.93184718803891187 ) ) ;
#127673=ADVANCED_FACE ( 'NONE', ( #170072 ), #81695, .F. ) ;
#127713=EDGE_CURVE ( 'NONE', #1871, #33092, #41172, .T. ) ;
#127717=CARTESIAN_POINT ( 'NONE',  ( -6.717278222822391953, -7.246166700180828535, 6.830415307812263137 ) ) ;
#127720=CARTESIAN_POINT ( 'NONE',  ( -0.3870072406890526229, 1.529612873802630002, 11.82510647457161923 ) ) ;
#127761=CARTESIAN_POINT ( 'NONE',  ( 0.2863826248021899001, -7.730039540835504930, -10.99644352130527025 ) ) ;
#127819=ORIENTED_EDGE ( 'NONE', *, *, #63516, .T. ) ;
#127831=CIRCLE ( 'NONE', #20558, 9.523431457505068920 ) ;
#127847=CARTESIAN_POINT ( 'NONE',  ( -0.1489494290324539782, -7.995840219786860992, -9.536979704252555479 ) ) ;
#127851=CARTESIAN_POINT ( 'NONE',  ( 1.668847547943344454E-13, 1.972237431424435750, 11.78526707783969663 ) ) ;
#127865=CARTESIAN_POINT ( 'NONE',  ( 7.777967379493318845, -5.907420853759296264, 7.744830294503448620 ) ) ;
#127875=VERTEX_POINT ( 'NONE', #125680 ) ;
#127888=ORIENTED_EDGE ( 'NONE', *, *, #201067, .T. ) ;
#127915=CARTESIAN_POINT ( 'NONE',  ( -4.792515913634093623E-13, -7.868798029037626485, 9.500000000000001776 ) ) ;
#127944=AXIS2_PLACEMENT_3D ( 'NONE', #85264, #2920, #135111 ) ;
#127978=CARTESIAN_POINT ( 'NONE',  ( 7.722692672890256738, -6.459788825448992355, 7.834474503270634216 ) ) ;
#128001=EDGE_CURVE ( 'NONE', #29585, #65129, #26520, .T. ) ;
#128008=ADVANCED_FACE ( 'NONE', ( #171142 ), #24881, .F. ) ;
#128025=CARTESIAN_POINT ( 'NONE',  ( 11.00029519899100805, -6.134628647623514119, 3.672734859294647059E-15 ) ) ;
#128045=ORIENTED_EDGE ( 'NONE', *, *, #167509, .T. ) ;
#128053=ORIENTED_EDGE ( 'NONE', *, *, #152080, .T. ) ;
#128080=CARTESIAN_POINT ( 'NONE',  ( -9.578245405452070926, -9.921948021430829101, 0.1647502191513203207 ) ) ;
#128091=ORIENTED_EDGE ( 'NONE', *, *, #133645, .T. ) ;
#128124=ORIENTED_EDGE ( 'NONE', *, *, #196046, .T. ) ;
#128139=ORIENTED_EDGE ( 'NONE', *, *, #186547, .T. ) ;
#128169=CARTESIAN_POINT ( 'NONE',  ( 11.07693626658187824, 1.970899860167824924, -4.005980692925287023 ) ) ;
#128170=CARTESIAN_POINT ( 'NONE',  ( -10.42995565840379335, 1.000000000000000888, 5.797106512947690860 ) ) ;
#128209=EDGE_LOOP ( 'NONE', ( #164504, #138179, #150828, #190856 ) ) ;
#128261=ORIENTED_EDGE ( 'NONE', *, *, #12966, .F. ) ;
#128277=CARTESIAN_POINT ( 'NONE',  ( 0.09623479069433779620, -9.919835240146305466, 9.499512666137798433 ) ) ;
#128321=CARTESIAN_POINT ( 'NONE',  ( 8.064677165291193717, -5.223431457505076203, -7.446209719563348983 ) ) ;
#128367=ORIENTED_EDGE ( 'NONE', *, *, #119057, .T. ) ;
#128394=EDGE_CURVE ( 'NONE', #162142, #68781, #111835, .T. ) ;
#128437=CIRCLE ( 'NONE', #159574, 11.99999999999999112 ) ;
#128471=DIRECTION ( 'NONE',  ( 0.000000000000000000, 1.000000000000000000, 0.000000000000000000 ) ) ;
#128508=ORIENTED_EDGE ( 'NONE', *, *, #200438, .T. ) ;
#128520=ORIENTED_EDGE ( 'NONE', *, *, #103265, .F. ) ;
#128562=DIRECTION ( 'NONE',  ( 6.217248937900876626E-15, 0.000000000000000000, 1.000000000000000000 ) ) ;
#128569=AXIS2_PLACEMENT_3D ( 'NONE', #90320, #74064, #39425 ) ;
#128592=ORIENTED_EDGE ( 'NONE', *, *, #41997, .T. ) ;
#128596=LINE ( 'NONE', #164205, #116474 ) ;
#128598=CARTESIAN_POINT ( 'NONE',  ( -9.605391220871888791, -6.900199406649615952, 0.04765083308772638526 ) ) ;
#128653=CARTESIAN_POINT ( 'NONE',  ( 8.029456579251872839, -5.199789852012450808, -7.518896314322964791 ) ) ;
#128654=VERTEX_POINT ( 'NONE', #67808 ) ;
#128656=LINE ( 'NONE', #210866, #43762 ) ;
#128676=CARTESIAN_POINT ( 'NONE',  ( 0.000000000000000000, 15.50000000000019362, 0.000000000000000000 ) ) ;
#128680=FACE_OUTER_BOUND ( 'NONE', #93349, .T. ) ;
#128682=CARTESIAN_POINT ( 'NONE',  ( -6.776370306708066948, -7.161464053357560644, -6.781144757626046626 ) ) ;
#128739=CARTESIAN_POINT ( 'NONE',  ( 7.654042494670951690E-16, 3.799999999999998046, -6.249999999999995559 ) ) ;
#128803=CARTESIAN_POINT ( 'NONE',  ( -1.938011383317839176E-15, -8.407420853759283830, -11.00029519899099917 ) ) ;
#128806=FACE_OUTER_BOUND ( 'NONE', #191684, .T. ) ;
#128868=CARTESIAN_POINT ( 'NONE',  ( 7.725699985795379199, -5.832912386296868590, -7.725699985795413838 ) ) ;
#128877=EDGE_CURVE ( 'NONE', #40383, #190182, #72634, .T. ) ;
#128893=CARTESIAN_POINT ( 'NONE',  ( -0.2943368945748598420, -8.203192640252309431, -9.495705940876561613 ) ) ;
#128928=EDGE_CURVE ( 'NONE', #96195, #76877, #97863, .T. ) ;
#128963=CARTESIAN_POINT ( 'NONE',  ( -0.05425791151749961849, -7.744511198441866640, 9.500000000000131450 ) ) ;
#128972=CARTESIAN_POINT ( 'NONE',  ( -0.04570195657714287013, 1.813436143228260855, 11.99992749206847975 ) ) ;
#128991=CARTESIAN_POINT ( 'NONE',  ( -8.748013565000578140, 3.829536045110815579, -7.724821879577381090 ) ) ;
#129019=EDGE_CURVE ( 'NONE', #183021, #146105, #170676, .T. ) ;
#129023=VERTEX_POINT ( 'NONE', #110020 ) ;
#129029=CARTESIAN_POINT ( 'NONE',  ( 6.717748655458900764, -7.473374494057228645, -6.717748655460318297 ) ) ;
#129031=ORIENTED_EDGE ( 'NONE', *, *, #151935, .T. ) ;
#129054=FILL_AREA_STYLE ('',( #212320 ) ) ;
#129062=CARTESIAN_POINT ( 'NONE',  ( 0.000000000000000000, 0.9200000000000041478, 6.329999999999995630 ) ) ;
#129065=ADVANCED_FACE ( 'NONE', ( #92661 ), #193327, .T. ) ;
#129071=EDGE_LOOP ( 'NONE', ( #172940, #119000, #17552, #137753 ) ) ;
#129112=VERTEX_POINT ( 'NONE', #117476 ) ;
#129113=FACE_OUTER_BOUND ( 'NONE', #161465, .T. ) ;
#129191=ORIENTED_EDGE ( 'NONE', *, *, #164748, .T. ) ;
#129237=FACE_OUTER_BOUND ( 'NONE', #162665, .T. ) ;
#129260=VERTEX_POINT ( 'NONE', #167233 ) ;
#129267=CARTESIAN_POINT ( 'NONE',  ( 0.000000000000000000, 3.499999999999989342, 0.000000000000000000 ) ) ;
#129296=CARTESIAN_POINT ( 'NONE',  ( 0.000000000000000000, 1.000000000000000888, 0.000000000000000000 ) ) ;
#129302=DIRECTION ( 'NONE',  ( 0.000000000000000000, 0.000000000000000000, 1.000000000000000000 ) ) ;
#129312=AXIS2_PLACEMENT_3D ( 'NONE', #46974, #30718, #212633 ) ;
#129329=ORIENTED_EDGE ( 'NONE', *, *, #44272, .T. ) ;
#129432=B_SPLINE_CURVE_WITH_KNOTS ( 'NONE', 3,
 ( #52097, #150679, #167976, #88878, #18513, #72592 ),
 .UNSPECIFIED., .F., .F.,
 ( 4, 2, 4 ),
 ( 0.000000000000000000, 0.001225895755212361030, 0.002451791510424721626 ),
 .UNSPECIFIED. ) ;
#129530=DIRECTION ( 'NONE',  ( -0.000000000000000000, -1.000000000000000000, -0.000000000000000000 ) ) ;
#129589=CARTESIAN_POINT ( 'NONE',  ( 2.763444990417154240E-17, -6.211932585243244986, 10.91339599544322958 ) ) ;
#129594=CARTESIAN_POINT ( 'NONE',  ( 0.000000000000000000, -5.166862915010145052, 0.000000000000000000 ) ) ;
#129606=VECTOR ( 'NONE', #188627, 1000.000000000000000 ) ;
#129624=CARTESIAN_POINT ( 'NONE',  ( -7.735357998705607585, -5.759585062615363071, 7.724608556409203075 ) ) ;
#129655=CIRCLE ( 'NONE', #108921, 9.499999999999992895 ) ;
#129656=ORIENTED_EDGE ( 'NONE', *, *, #22175, .F. ) ;
#129681=UNCERTAINTY_MEASURE_WITH_UNIT (LENGTH_MEASURE( 1.000000000000000082E-05 ), #107100, 'distance_accuracy_value', 'NONE');
#129734=EDGE_CURVE ( 'NONE', #1301, #146171, #115224, .T. ) ;
#129745=CARTESIAN_POINT ( 'NONE',  ( -11.40591166468356654, 3.507114751586590362, 3.706005353348402753 ) ) ;
#129762=VECTOR ( 'NONE', #168923, 1000.000000000000114 ) ;
#129825=CARTESIAN_POINT ( 'NONE',  ( 7.727353211424198065, -6.453073674884657329, -7.679448064523601403 ) ) ;
#129836=ORIENTED_EDGE ( 'NONE', *, *, #12907, .F. ) ;
#129852=CARTESIAN_POINT ( 'NONE',  ( 0.05513001983271961781, -8.135652870098732947, 11.00000000000013145 ) ) ;
#129854=DIRECTION ( 'NONE',  ( 0.000000000000000000, 1.000000000000000000, 0.000000000000000000 ) ) ;
#129894=( GEOMETRIC_REPRESENTATION_CONTEXT ( 3 ) GLOBAL_UNCERTAINTY_ASSIGNED_CONTEXT ( ( #159448 ) ) GLOBAL_UNIT_ASSIGNED_CONTEXT ( ( #213381, #114541, #160398 ) ) REPRESENTATION_CONTEXT ( 'NONE', 'WORKASPACE' ) );
#129942=DIRECTION ( 'NONE',  ( 0.000000000000000000, 0.000000000000000000, 1.000000000000000000 ) ) ;
#129985=CARTESIAN_POINT ( 'NONE',  ( 0.4644097342742976586, -8.200000000000015277, 9.488641820551100281 ) ) ;
#130087=CARTESIAN_POINT ( 'NONE',  ( 7.778383330260374429, -6.134628647623487474, 7.778383330260353112 ) ) ;
#130121=AXIS2_PLACEMENT_3D ( 'NONE', #51235, #34962, #101032 ) ;
#130126=LINE ( 'NONE', #186228, #176296 ) ;
#130129=CARTESIAN_POINT ( 'NONE',  ( 0.000000000000000000, -13.99999999999999822, 6.249999999999995559 ) ) ;
#130130=ORIENTED_EDGE ( 'NONE', *, *, #131984, .F. ) ;
#130167=CARTESIAN_POINT ( 'NONE',  ( -0.07995206772520195571, -9.200995477224077845, 9.499751636909056884 ) ) ;
#130192=CARTESIAN_POINT ( 'NONE',  ( 6.625366561259610876, -8.010031549403125339, 6.808607288253734069 ) ) ;
#130205=AXIS2_PLACEMENT_3D ( 'NONE', #77326, #146626, #80529 ) ;
#130207=ORIENTED_EDGE ( 'NONE', *, *, #39457, .T. ) ;
#130219=CARTESIAN_POINT ( 'NONE',  ( 0.08000000000000020983, -7.473374494045017968, -9.579665964948882007 ) ) ;
#130242=ORIENTED_EDGE ( 'NONE', *, *, #106666, .T. ) ;
#130248=ORIENTED_EDGE ( 'NONE', *, *, #44338, .T. ) ;
#130252=CARTESIAN_POINT ( 'NONE',  ( -10.99462144896568283, -5.166862915010298707, 0.3541067150203592862 ) ) ;
#130265=B_SPLINE_CURVE_WITH_KNOTS ( 'NONE', 3,
 ( #157907, #59316, #111339, #28956, #75573, #113474, #141682 ),
 .UNSPECIFIED., .F., .F.,
 ( 4, 3, 4 ),
 ( 0.0001135037245265591781, 0.001517139415464318795, 0.002007692284160929319 ),
 .UNSPECIFIED. ) ;
#130284=CARTESIAN_POINT ( 'NONE',  ( 10.90726532705803820, -6.287979527546280423, -0.008173644115955716258 ) ) ;
#130287=CARTESIAN_POINT ( 'NONE',  ( -0.08058608058608254798, -9.900000000000005684, -10.99970480893080804 ) ) ;
#130289=CARTESIAN_POINT ( 'NONE',  ( -9.549638505170037206, -6.527411821100059797, 0.4330238300980920885 ) ) ;
#130308=ORIENTED_EDGE ( 'NONE', *, *, #186461, .T. ) ;
#130315=SURFACE_STYLE_FILL_AREA ( #210400 ) ;
#130317=SURFACE_STYLE_USAGE ( .BOTH. , #77207 ) ;
#130327=ORIENTED_EDGE ( 'NONE', *, *, #177138, .T. ) ;
#130330=CARTESIAN_POINT ( 'NONE',  ( -0.01167607004468995333, -5.765528217051257620, 11.00020965659534156 ) ) ;
#130349=VERTEX_POINT ( 'NONE', #112857 ) ;
#130351=VERTEX_POINT ( 'NONE', #178873 ) ;
#130358=ORIENTED_EDGE ( 'NONE', *, *, #145267, .T. ) ;
#130360=AXIS2_PLACEMENT_3D ( 'NONE', #183451, #1472, #117457 ) ;
#130388=CARTESIAN_POINT ( 'NONE',  ( -9.500587730663498931, -7.019129742887085577, 0.03636482241358145878 ) ) ;
#130423=CIRCLE ( 'NONE', #137314, 0.08000000000000020983 ) ;
#130425=EDGE_LOOP ( 'NONE', ( #7489, #124591, #193539, #122128, #46868, #152378 ) ) ;
#130438=CARTESIAN_POINT ( 'NONE',  ( -7.863746947443979174, -5.507058666270983949, 7.245729715095587053 ) ) ;
#130528=ORIENTED_EDGE ( 'NONE', *, *, #158732, .T. ) ;
#130546=AXIS2_PLACEMENT_3D ( 'NONE', #47864, #98719, #183157 ) ;
#130554=AXIS2_PLACEMENT_3D ( 'NONE', #72342, #124407, #121203 ) ;
#130557=EDGE_CURVE ( 'NONE', #29173, #121012, #7841, .T. ) ;
#130618=EDGE_CURVE ( 'NONE', #78199, #17720, #200403, .T. ) ;
#130629=DIRECTION ( 'NONE',  ( 0.000000000000000000, 1.000000000000000000, 0.000000000000000000 ) ) ;
#130641=CARTESIAN_POINT ( 'NONE',  ( 0.4356160240586413046, -9.063431457505064515, -9.626717610576614348 ) ) ;
#130657=AXIS2_PLACEMENT_3D ( 'NONE', #127717, #177443, #178509 ) ;
#130765=EDGE_LOOP ( 'NONE', ( #22148, #141825, #19596, #12687, #35410, #130308, #20170, #16378, #161190, #204616, #1230, #53822, #63929, #118844, #203647, #58422, #45755, #101760, #2254, #173969, #144566, #209177, #43052, #101889 ) ) ;
#130769=EDGE_LOOP ( 'NONE', ( #166210, #146321, #88839 ) ) ;
#130782=DIRECTION ( 'NONE',  ( 0.000000000000000000, -1.000000000000000000, 0.000000000000000000 ) ) ;
#130785=EDGE_CURVE ( 'NONE', #18108, #192481, #118178, .T. ) ;
#130791=CARTESIAN_POINT ( 'NONE',  ( 8.902524791715917374, 3.162178953954597471, 7.495381307383154557 ) ) ;
#130804=EDGE_CURVE ( 'NONE', #127875, #83638, #163208, .T. ) ;
#130881=CARTESIAN_POINT ( 'NONE',  ( 11.00009153390426420, -6.553298220693314136, -0.005414006223990005216 ) ) ;
#130896=CARTESIAN_POINT ( 'NONE',  ( 6.710127771514622808, -7.162053774861990796, 6.725445687907760650 ) ) ;
#130897=EDGE_CURVE ( 'NONE', #81410, #29860, #77268, .T. ) ;
#130923=CARTESIAN_POINT ( 'NONE',  ( 0.4382560683119230416, -7.700000000000008171, -10.99126615174918165 ) ) ;
#130927=CARTESIAN_POINT ( 'NONE',  ( 0.000000000000000000, 4.000000000000003553, 0.000000000000000000 ) ) ;
#130931=CARTESIAN_POINT ( 'NONE',  ( 9.578219923806454261, -9.914766490055704651, -0.1663656176996578528 ) ) ;
#130944=VECTOR ( 'NONE', #23378, 1000.000000000000000 ) ;
#130973=B_SPLINE_CURVE_WITH_KNOTS ( 'NONE', 3,
 ( #116674, #34294, #100367, #47386 ),
 .UNSPECIFIED., .F., .F.,
 ( 4, 4 ),
 ( 0.000000000000000000, 0.0002909236271752587821 ),
 .UNSPECIFIED. ) ;
#131005=ORIENTED_EDGE ( 'NONE', *, *, #48325, .F. ) ;
#131024=CARTESIAN_POINT ( 'NONE',  ( -7.846302513400014611, -6.700642373080271774, 7.709579522695861442 ) ) ;
#131027=CARTESIAN_POINT ( 'NONE',  ( 0.000000000000000000, -9.006862915010128035, 0.000000000000000000 ) ) ;
#131032=CARTESIAN_POINT ( 'NONE',  ( 0.3909723190919997537, -8.176244038173743789, 9.516020521605820903 ) ) ;
#131051=EDGE_CURVE ( 'NONE', #114731, #157260, #188471, .T. ) ;
#131053=CARTESIAN_POINT ( 'NONE',  ( 9.876669921572342990E-13, -7.246166700193024113, -9.500331257164619458 ) ) ;
#131077=PRESENTATION_STYLE_ASSIGNMENT (( #41516 ) ) ;
#131103=CARTESIAN_POINT ( 'NONE',  ( 6.783773228136841027, -6.684699857435559167, -6.634380643896355068 ) ) ;
#131137=CARTESIAN_POINT ( 'NONE',  ( 0.07804408512527075126, -9.997559919034475939, 9.579522898042023726 ) ) ;
#131152=AXIS2_PLACEMENT_3D ( 'NONE', #129267, #142249, #195239 ) ;
#131164=CARTESIAN_POINT ( 'NONE',  ( 9.479415819240319507, -6.570271182191715020, -0.2417854191286350762 ) ) ;
#131173=CARTESIAN_POINT ( 'NONE',  ( 4.232369794311310053E-13, -9.350066838357705024, 9.500000000000001776 ) ) ;
#131190=AXIS2_PLACEMENT_3D ( 'NONE', #67522, #66456, #69664 ) ;
#131239=EDGE_CURVE ( 'NONE', #173465, #162142, #39238, .T. ) ;
#131243=CARTESIAN_POINT ( 'NONE',  ( -9.578659721986371167, -9.971093151297267809, 0.1384029864568004642 ) ) ;
#131267=CARTESIAN_POINT ( 'NONE',  ( 0.000000000000000000, -5.166862915010145052, 0.000000000000000000 ) ) ;
#131277=CYLINDRICAL_SURFACE ( 'NONE', #109121, 0.08000000000000020983 ) ;
#131278=DIRECTION ( 'NONE',  ( 0.000000000000000000, 0.000000000000000000, 1.000000000000000000 ) ) ;
#131280=ORIENTED_EDGE ( 'NONE', *, *, #127420, .T. ) ;
#131327=ORIENTED_EDGE ( 'NONE', *, *, #133268, .T. ) ;
#131353=AXIS2_PLACEMENT_3D ( 'NONE', #79617, #29818, #111122 ) ;
#131449=CARTESIAN_POINT ( 'NONE',  ( 11.37385970535889257, 1.000000000000000888, -3.825613075418463627 ) ) ;
#131507=SURFACE_SIDE_STYLE ('',( #97912 ) ) ;
#131559=FACE_OUTER_BOUND ( 'NONE', #83636, .T. ) ;
#131570=VERTEX_POINT ( 'NONE', #18206 ) ;
#131618=FACE_OUTER_BOUND ( 'NONE', #208621, .T. ) ;
#131685=LINE ( 'NONE', #64505, #173050 ) ;
#131687=CARTESIAN_POINT ( 'NONE',  ( 0.4299312922663348080, -6.708819892820487851, 9.481437597266053174 ) ) ;
#131704=( BOUNDED_SURFACE ( )  B_SPLINE_SURFACE ( 3, 2, ( 
 ( #126418, #58134, #175105 ),
 ( #154576, #6152, #190252 ),
 ( #192381, #44036, #124293 ),
 ( #188122, #39753, #105858 ) ),
 .UNSPECIFIED., .F., .F., .T. ) 
 B_SPLINE_SURFACE_WITH_KNOTS ( ( 4, 4 ),
 ( 3, 3 ),
 ( 0.01126995942960227343, 0.01373815140602663992 ),
 ( 0.000000000000000000, 1.000000000000000000 ),
 .UNSPECIFIED. ) 
 GEOMETRIC_REPRESENTATION_ITEM ( )  RATIONAL_B_SPLINE_SURFACE ( (
 ( 1.000000000000000000, 0.6947640035331656971, 1.000000000000000000),
 ( 1.000000000000000000, 0.6955505939616358768, 1.000000000000000000),
 ( 1.000000000000000000, 0.6961913616428402340, 1.000000000000000000),
 ( 1.000000000000000000, 0.6967468848049985786, 1.000000000000000000) ) ) 
 REPRESENTATION_ITEM ( '' )  SURFACE ( )  );
#131705=EDGE_LOOP ( 'NONE', ( #38018, #189933, #20225, #177427 ) ) ;
#131711=CARTESIAN_POINT ( 'NONE',  ( -8.013579835756335257, -5.223163706540480788, 7.501945787865621718 ) ) ;
#131808=ORIENTED_EDGE ( 'NONE', *, *, #120547, .T. ) ;
#131832=CARTESIAN_POINT ( 'NONE',  ( -0.06856108760742431196, -7.850763007174490049, -9.549252947205625119 ) ) ;
#131880=ORIENTED_EDGE ( 'NONE', *, *, #93674, .T. ) ;
#131892=CARTESIAN_POINT ( 'NONE',  ( 7.097136523687877840, -8.233137084989836652, -6.434831245971841973 ) ) ;
#131920=CARTESIAN_POINT ( 'NONE',  ( 0.000000000000000000, 1.000000000000000888, 0.000000000000000000 ) ) ;
#131926=CARTESIAN_POINT ( 'NONE',  ( 0.000000000000000000, -5.199999999999996625, 0.000000000000000000 ) ) ;
#131936=CARTESIAN_POINT ( 'NONE',  ( 6.773846765317334651, -7.246166700180801001, 6.773846765317318663 ) ) ;
#131941=DIRECTION ( 'NONE',  ( 0.000000000000000000, 0.08676576675288256990, 0.9962287396576072762 ) ) ;
#131967=SURFACE_STYLE_FILL_AREA ( #211023 ) ;
#131984=EDGE_CURVE ( 'NONE', #56213, #67059, #146422, .T. ) ;
#132002=DIRECTION ( 'NONE',  ( 0.000000000000000000, 0.000000000000000000, 1.000000000000000000 ) ) ;
#132043=LINE ( 'NONE', #48631, #67220 ) ;
#132056=EDGE_CURVE ( 'NONE', #101997, #114731, #122362, .T. ) ;
#132058=SURFACE_STYLE_FILL_AREA ( #183955 ) ;
#132067=CARTESIAN_POINT ( 'NONE',  ( -11.29517787156874853, -8.030538574678853792, 0.1971580631239607251 ) ) ;
#132069=ORIENTED_EDGE ( 'NONE', *, *, #186635, .F. ) ;
#132076=CIRCLE ( 'NONE', #80238, 11.89429233241351902 ) ;
#132088=VECTOR ( 'NONE', #53838, 1000.000000000000000 ) ;
#132089=DIRECTION ( 'NONE',  ( 0.000000000000000000, 1.000000000000000000, 0.000000000000000000 ) ) ;
#132118=CARTESIAN_POINT ( 'NONE',  ( 6.827626583076773947, -7.154544010627095219, 6.720112740279239105 ) ) ;
#132124=( BOUNDED_SURFACE ( )  B_SPLINE_SURFACE ( 3, 2, ( 
 ( #114958, #195088, #46726 ),
 ( #112838, #213438, #32581 ),
 ( #80266, #96550, #162597 ),
 ( #64020, #98657, #130167 ),
 ( #164713, #196159, #16301 ),
 ( #170031, #85586, #168971 ),
 ( #87726, #21618, #2173 ),
 ( #20573, #84524, #102911 ) ),
 .UNSPECIFIED., .F., .F., .T. ) 
 B_SPLINE_SURFACE_WITH_KNOTS ( ( 4, 2, 2, 4 ),
 ( 3, 3 ),
 ( 0.000000000000000000, 0.0004912655988793406025, 0.0007368983983190109579, 0.0009825311977586812049 ),
 ( 0.000000000000000000, 1.000000000000000000 ),
 .UNSPECIFIED. ) 
 GEOMETRIC_REPRESENTATION_ITEM ( )  RATIONAL_B_SPLINE_SURFACE ( (
 ( 1.000000000000000000, 0.7100530722026821007, 1.000000000000000000),
 ( 1.000000000000000000, 0.6561915434216080145, 1.000000000000000000),
 ( 1.000000000000000000, 0.5915413786744014857, 1.000000000000000000),
 ( 1.000000000000000000, 0.4908282809847615002, 1.000000000000000000),
 ( 1.000000000000000000, 0.4560392263211024977, 1.000000000000000000),
 ( 1.000000000000000000, 0.3997350557757124445, 1.000000000000000000),
 ( 1.000000000000000000, 0.3799210206804777279, 1.000000000000000000),
 ( 1.000000000000000000, 0.3826834323650904479, 1.000000000000000000) ) ) 
 REPRESENTATION_ITEM ( '' )  SURFACE ( )  );
#132143=EDGE_LOOP ( 'NONE', ( #111842, #159306, #19165, #90202 ) ) ;
#132145=CARTESIAN_POINT ( 'NONE',  ( 0.000000000000000000, 1.000000000000002665, 6.329999999999995630 ) ) ;
#132195=CARTESIAN_POINT ( 'NONE',  ( 0.000000000000000000, 0.9200000000000041478, 0.000000000000000000 ) ) ;
#132222=TOROIDAL_SURFACE ( 'NONE', #204826, 9.580000000000001847, 0.08000000000000000167 ) ;
#132224=CARTESIAN_POINT ( 'NONE',  ( 10.99180900346484968, -6.701306620465910413, -0.4265819271707739779 ) ) ;
#132249=SURFACE_STYLE_USAGE ( .BOTH. , #54162 ) ;
#132250=ORIENTED_EDGE ( 'NONE', *, *, #189331, .T. ) ;
#132282=CARTESIAN_POINT ( 'NONE',  ( 10.91132967064556070, -5.166862915010145052, -0.4350687514514655629 ) ) ;
#132317=CARTESIAN_POINT ( 'NONE',  ( 6.922231005658577629, -8.202869699938531767, -6.506745451169505756 ) ) ;
#132353=B_SPLINE_CURVE_WITH_KNOTS ( 'NONE', 3,
 ( #114174, #162861, #97868, #15504, #81591, #12310, #195353, #78391, #144511, #210519 ),
 .UNSPECIFIED., .F., .F.,
 ( 4, 2, 2, 2, 4 ),
 ( 0.000000000000000000, 0.0002216178067634652128, 0.0004432356135269304256, 0.0006648534202903956655, 0.0008864712270538608512 ),
 .UNSPECIFIED. ) ;
#132395=CARTESIAN_POINT ( 'NONE',  ( -1.734299959503179353E-15, -8.332912386296857932, -10.92578969873748740 ) ) ;
#132415=CARTESIAN_POINT ( 'NONE',  ( -9.578206935422265644, -9.825744180092243596, 0.1671882239536719994 ) ) ;
#132420=CARTESIAN_POINT ( 'NONE',  ( 0.08269815893116483352, -5.360092950639683274, 10.99976946526262900 ) ) ;
#132438=CARTESIAN_POINT ( 'NONE',  ( -10.55819884875827697, -6.268611901546719878, 1.734723475976807094E-15 ) ) ;
#132443=AXIS2_PLACEMENT_3D ( 'NONE', #4190, #155817, #37792 ) ;
#132450=CARTESIAN_POINT ( 'NONE',  ( 7.721398836998367265, -6.134628647623499909, -7.721398836998390358 ) ) ;
#132470=ORIENTED_EDGE ( 'NONE', *, *, #164748, .F. ) ;
#132483=CARTESIAN_POINT ( 'NONE',  ( 0.08367765422324577318, -9.912493506416723221, 9.499631469177300502 ) ) ;
#132492=EDGE_CURVE ( 'NONE', #129260, #42950, #149951, .T. ) ;
#132498=CIRCLE ( 'NONE', #80673, 6.249999999999995559 ) ;
#132516=AXIS2_PLACEMENT_3D ( 'NONE', #65684, #119865, #181585 ) ;
#132620=EDGE_CURVE ( 'NONE', #127089, #96541, #28520, .T. ) ;
#132666=CARTESIAN_POINT ( 'NONE',  ( 1.637338291174485510E-15, -6.530144695498204754, 11.00000000000000178 ) ) ;
#132670=DIRECTION ( 'NONE',  ( 0.000000000000000000, 0.000000000000000000, -1.000000000000000000 ) ) ;
#132716=CARTESIAN_POINT ( 'NONE',  ( -2.331034670843834533E-15, -7.868711954895448280, 9.183873791909961781 ) ) ;
#132763=CARTESIAN_POINT ( 'NONE',  ( 10.99935770452674610, -5.294776013890325039, -0.1368885365587498570 ) ) ;
#132776=CARTESIAN_POINT ( 'NONE',  ( 6.663994888585881959, -7.154544010627095219, -6.770610912236887380 ) ) ;
#132816=B_SPLINE_CURVE_WITH_KNOTS ( 'NONE', 3,
 ( #192792, #100370, #128963, #127915 ),
 .UNSPECIFIED., .F., .F.,
 ( 4, 4 ),
 ( 0.000000000000000000, 0.0004037790303856251119 ),
 .UNSPECIFIED. ) ;
#132855=ORIENTED_EDGE ( 'NONE', *, *, #107143, .F. ) ;
#132872=UNCERTAINTY_MEASURE_WITH_UNIT (LENGTH_MEASURE( 1.000000000000000082E-05 ), #140026, 'distance_accuracy_value', 'NONE');
#132877=DIRECTION ( 'NONE',  ( -1.000000000000000000, 0.000000000000000000, 0.000000000000000000 ) ) ;
#132907=ORIENTED_EDGE ( 'NONE', *, *, #153405, .F. ) ;
#132914=CARTESIAN_POINT ( 'NONE',  ( -8.103009739377982967, -6.893137084989842123, 7.439168848974024861 ) ) ;
#132940=CARTESIAN_POINT ( 'NONE',  ( -6.773846765317318663, -7.246166700180828535, 6.773846765317342644 ) ) ;
#132983=( NAMED_UNIT ( * ) SI_UNIT ( $, .STERADIAN. ) SOLID_ANGLE_UNIT ( ) );
#133000=DIRECTION ( 'NONE',  ( 0.000000000000000000, 0.000000000000000000, 1.000000000000000000 ) ) ;
#133029=CARTESIAN_POINT ( 'NONE',  ( 9.578796289606994918, -9.978085408363298825, -0.1296641399399049710 ) ) ;
#133125=CARTESIAN_POINT ( 'NONE',  ( -0.08000000000000367928, 7.849261790823902629, 9.579665964948883783 ) ) ;
#133128=CARTESIAN_POINT ( 'NONE',  ( -0.1000000000000080685, -9.919999999999998153, -10.91954211494235238 ) ) ;
#133129=ORIENTED_EDGE ( 'NONE', *, *, #106815, .F. ) ;
#133156=B_SPLINE_CURVE_WITH_KNOTS ( 'NONE', 3,
 ( #156956, #190490, #83135, #82072 ),
 .UNSPECIFIED., .F., .F.,
 ( 4, 4 ),
 ( 0.0005910214237607931166, 0.001001414237305830969 ),
 .UNSPECIFIED. ) ;
#133179=CARTESIAN_POINT ( 'NONE',  ( 0.09999999999999592548, -9.999999999999994671, 10.91954211494236660 ) ) ;
#133198=ADVANCED_FACE ( 'NONE', ( #210437 ), #62078, .T. ) ;
#133236=CARTESIAN_POINT ( 'NONE',  ( 8.948250016579860855, 1.813773193624685254, 7.995571895478047253 ) ) ;
#133244=CARTESIAN_POINT ( 'NONE',  ( -6.773846765307970585, -7.473374494058216300, 6.773846765307992790 ) ) ;
#133268=EDGE_CURVE ( 'NONE', #110438, #131570, #100616, .T. ) ;
#133286=CARTESIAN_POINT ( 'NONE',  ( -0.4366904681730566784, -5.787668213791788752, -10.40319425600973346 ) ) ;
#133304=FACE_OUTER_BOUND ( 'NONE', #159411, .T. ) ;
#133315=AXIS2_PLACEMENT_3D ( 'NONE', #108021, #155637, #207573 ) ;
#133343=DIRECTION ( 'NONE',  ( 0.000000000000000000, -1.000000000000000000, 0.000000000000000000 ) ) ;
#133381=CARTESIAN_POINT ( 'NONE',  ( -7.404765023120893019, -6.836271202499959010, -7.949604103952373713 ) ) ;
#133392=VERTEX_POINT ( 'NONE', #79386 ) ;
#133394=( BOUNDED_SURFACE ( )  B_SPLINE_SURFACE ( 3, 2, ( 
 ( #163438, #15018, #147195 ),
 ( #64850, #164494, #16080 ),
 ( #82163, #34484, #18221 ),
 ( #203367, #84306, #71234 ) ),
 .UNSPECIFIED., .F., .F., .T. ) 
 B_SPLINE_SURFACE_WITH_KNOTS ( ( 4, 4 ),
 ( 3, 3 ),
 ( 8.470329472543003391E-22, 3.124390317667046857E-05 ),
 ( 0.000000000000000000, 1.000000000000000000 ),
 .UNSPECIFIED. ) 
 GEOMETRIC_REPRESENTATION_ITEM ( )  RATIONAL_B_SPLINE_SURFACE ( (
 ( 1.000000000000000000, 0.7071067811860876073, 1.000000000000000000),
 ( 1.000000000000000000, 0.7090998123827956245, 1.000000000000000000),
 ( 1.000000000000000000, 0.7100789167761989429, 1.000000000000000000),
 ( 1.000000000000000000, 0.7100530722022271313, 1.000000000000000000) ) ) 
 REPRESENTATION_ITEM ( '' )  SURFACE ( )  );
#133404=CARTESIAN_POINT ( 'NONE',  ( 10.34545848478754237, -8.336144560139965520, -0.6172425113790489526 ) ) ;
#133437=CARTESIAN_POINT ( 'NONE',  ( 9.620809655836525920, -9.180994456877186849, -0.3503521373105082937 ) ) ;
#133444=( NAMED_UNIT ( * ) PLANE_ANGLE_UNIT ( ) SI_UNIT ( $, .RADIAN. ) );
#133449=AXIS2_PLACEMENT_3D ( 'NONE', #194659, #209830, #46303 ) ;
#133460=ORIENTED_EDGE ( 'NONE', *, *, #56480, .F. ) ;
#133466=EDGE_CURVE ( 'NONE', #157711, #55041, #12745, .T. ) ;
#133478=LINE ( 'NONE', #14336, #56328 ) ;
#133517=CARTESIAN_POINT ( 'NONE',  ( -6.506163559800210550, -8.203199116536534774, -6.922777049148881368 ) ) ;
#133519=CARTESIAN_POINT ( 'NONE',  ( 9.499656837482749694, -9.914216672575010492, -0.08076498840996278183 ) ) ;
#133529=ADVANCED_FACE ( 'NONE', ( #198448 ), #161721, .T. ) ;
#133532=ORIENTED_EDGE ( 'NONE', *, *, #40826, .T. ) ;
#133547=CARTESIAN_POINT ( 'NONE',  ( 0.02500845152586854067, 3.700502905159954725, -11.79962023279681560 ) ) ;
#133559=AXIS2_PLACEMENT_3D ( 'NONE', #91541, #170619, #121962 ) ;
#133563=CIRCLE ( 'NONE', #157668, 9.616019636405017224 ) ;
#133588=CARTESIAN_POINT ( 'NONE',  ( -10.91255906795571562, 3.426985321572576737, 3.952372590954746023 ) ) ;
#133598=VECTOR ( 'NONE', #78771, 1000.000000000000000 ) ;
#133641=VERTEX_POINT ( 'NONE', #22889 ) ;
#133645=EDGE_CURVE ( 'NONE', #151754, #5447, #167045, .T. ) ;
#133796=CARTESIAN_POINT ( 'NONE',  ( -8.673617379884035472E-15, 3.507114751586604129, -11.99288524841337455 ) ) ;
#133851=B_SPLINE_CURVE_WITH_KNOTS ( 'NONE', 3,
 ( #174047, #125349, #109090, #73296, #106945, #189199, #92794, #123234 ),
 .UNSPECIFIED., .F., .F.,
 ( 4, 2, 2, 4 ),
 ( 0.000000000000000000, 0.0001985720215089283687, 0.0003971440430178567373, 0.0007942880860357131494 ),
 .UNSPECIFIED. ) ;
#133855=CARTESIAN_POINT ( 'NONE',  ( -0.2903707658989356788, -5.254568858751054172, -10.97058181929407716 ) ) ;
#133866=CARTESIAN_POINT ( 'NONE',  ( -10.99970480893081337, -6.134628647623513231, -0.08058608058607207025 ) ) ;
#133904=AXIS2_PLACEMENT_3D ( 'NONE', #102572, #104724, #103651 ) ;
#133924=LINE ( 'NONE', #19047, #122707 ) ;
#133942=FACE_OUTER_BOUND ( 'NONE', #186990, .T. ) ;
#133975=LINE ( 'NONE', #85179, #52755 ) ;
#133993=DIRECTION ( 'NONE',  ( -0.9990890794760038940, 0.000000000000000000, 0.04267330865764931702 ) ) ;
#134004=( BOUNDED_SURFACE ( )  B_SPLINE_SURFACE ( 3, 2, ( 
 ( #69961, #51624, #151257 ),
 ( #54816, #2827, #1763 ),
 ( #116666, #68898, #202088 ),
 ( #4952, #135017, #182664 ) ),
 .UNSPECIFIED., .F., .F., .F. ) 
 B_SPLINE_SURFACE_WITH_KNOTS ( ( 4, 4 ),
 ( 3, 3 ),
 ( 0.000000000000000000, 3.124390133962077760E-05 ),
 ( 0.000000000000000000, 1.000000000000000000 ),
 .UNSPECIFIED. ) 
 GEOMETRIC_REPRESENTATION_ITEM ( )  RATIONAL_B_SPLINE_SURFACE ( (
 ( 1.000000000000000000, 0.7100530722023767893, 1.000000000000000000),
 ( 1.000000000000000000, 0.7100778649077733595, 1.000000000000000000),
 ( 1.000000000000000000, 0.7091082185075940902, 1.000000000000000000),
 ( 1.000000000000000000, 0.7071067811862460362, 1.000000000000000000) ) ) 
 REPRESENTATION_ITEM ( '' )  SURFACE ( )  );
#134016=CARTESIAN_POINT ( 'NONE',  ( -7.550983558724425393, -6.148216694138056049, 7.550983558724451150 ) ) ;
#134058=DIRECTION ( 'NONE',  ( 0.000000000000000000, 1.000000000000000000, 0.000000000000000000 ) ) ;
#134100=CARTESIAN_POINT ( 'NONE',  ( 9.579089671862750066, -9.990657512341117652, -0.1108584966531479393 ) ) ;
#134105=ORIENTED_EDGE ( 'NONE', *, *, #143796, .F. ) ;
#134113=EDGE_CURVE ( 'NONE', #34907, #86477, #90744, .T. ) ;
#134162=DIRECTION ( 'NONE',  ( 0.000000000000000000, 0.000000000000000000, 1.000000000000000000 ) ) ;
#134180=( NAMED_UNIT ( * ) PLANE_ANGLE_UNIT ( ) SI_UNIT ( $, .RADIAN. ) );
#134212=ADVANCED_FACE ( 'NONE', ( #64242 ), #199324, .T. ) ;
#134215=DIRECTION ( 'NONE',  ( 1.000000000000000000, 0.000000000000000000, -1.224646799147353207E-16 ) ) ;
#134234=CARTESIAN_POINT ( 'NONE',  ( 8.773304256324777839, 3.742896273583256939, 7.826845210040881184 ) ) ;
#134260=CARTESIAN_POINT ( 'NONE',  ( 0.000000000000000000, -6.893137084989842123, 0.000000000000000000 ) ) ;
#134269=CARTESIAN_POINT ( 'NONE',  ( 10.10493793804581131, 0.9691415390508739680, 6.281047173807365880 ) ) ;
#134278=ORIENTED_EDGE ( 'NONE', *, *, #150154, .T. ) ;
#134300=CARTESIAN_POINT ( 'NONE',  ( -0.09053139919707911543, -9.918143888366140359, -9.499568811299521798 ) ) ;
#134318=AXIS2_PLACEMENT_3D ( 'NONE', #103986, #5368, #205726 ) ;
#134319=( GEOMETRIC_REPRESENTATION_CONTEXT ( 3 ) GLOBAL_UNCERTAINTY_ASSIGNED_CONTEXT ( ( #64590 ) ) GLOBAL_UNIT_ASSIGNED_CONTEXT ( ( #63100, #193092, #196306 ) ) REPRESENTATION_CONTEXT ( 'NONE', 'WORKASPACE' ) );
#134335=CARTESIAN_POINT ( 'NONE',  ( 0.000000000000000000, -7.154544010627095219, 0.000000000000000000 ) ) ;
#134345=DIRECTION ( 'NONE',  ( 7.610300982150707428E-15, -1.000000000000000000, -7.722633184682877167E-15 ) ) ;
#134348=EDGE_CURVE ( 'NONE', #149119, #197280, #170445, .T. ) ;
#134353=CARTESIAN_POINT ( 'NONE',  ( 10.99374989157287885, -6.893136995915043919, -0.3811408430856385587 ) ) ;
#134380=CARTESIAN_POINT ( 'NONE',  ( 7.777967379493318845, -9.999999999999994671, 7.664830294503448549 ) ) ;
#134414=AXIS2_PLACEMENT_3D ( 'NONE', #197332, #122586, #168040 ) ;
#134446=CARTESIAN_POINT ( 'NONE',  ( -7.008396152629729592, -6.708819892820514497, 6.400381488218093828 ) ) ;
#134462=ORIENTED_EDGE ( 'NONE', *, *, #134113, .F. ) ;
#134471=CARTESIAN_POINT ( 'NONE',  ( 10.75419052074084902, -7.927673425445468602, -0.6248749548428326195 ) ) ;
#134474=ADVANCED_FACE ( 'NONE', ( #19736 ), #15095, .F. ) ;
#134495=ADVANCED_FACE ( 'NONE', ( #135645 ), #168977, .T. ) ;
#134540=EDGE_CURVE ( 'NONE', #17507, #81410, #59179, .T. ) ;
#134549=B_SPLINE_CURVE_WITH_KNOTS ( 'NONE', 3,
 ( #120604, #92330, #190840, #7819 ),
 .UNSPECIFIED., .F., .F.,
 ( 4, 4 ),
 ( 0.000000000000000000, 6.033646489354672709E-05 ),
 .UNSPECIFIED. ) ;
#134568=ORIENTED_EDGE ( 'NONE', *, *, #76837, .F. ) ;
#134578=CARTESIAN_POINT ( 'NONE',  ( 7.727873494160014900, -5.742104877864247392, -7.828177403543865154 ) ) ;
#134583=DIRECTION ( 'NONE',  ( 0.000000000000000000, 0.000000000000000000, -1.000000000000000000 ) ) ;
#134585=CARTESIAN_POINT ( 'NONE',  ( 7.446209719563365859, -5.223431457505076203, 8.064677165291195493 ) ) ;
#134610=CARTESIAN_POINT ( 'NONE',  ( 0.1515253745957860221, 3.870538056096196833, -11.62858902121510951 ) ) ;
#134641=DIRECTION ( 'NONE',  ( -0.04267330865764863701, 0.000000000000000000, -0.9990890794760038940 ) ) ;
#134642=CARTESIAN_POINT ( 'NONE',  ( -9.498553103985718948, -9.900000000000005684, 0.1657978611541623959 ) ) ;
#134651=DIRECTION ( 'NONE',  ( -0.000000000000000000, -1.000000000000000000, -0.000000000000000000 ) ) ;
#134699=SURFACE_STYLE_FILL_AREA ( #151992 ) ;
#134720=AXIS2_PLACEMENT_3D ( 'NONE', #193367, #129530, #143601 ) ;
#134722=DIRECTION ( 'NONE',  ( 0.000000000000000000, -1.000000000000000000, 0.000000000000000000 ) ) ;
#134803=MECHANICAL_DESIGN_GEOMETRIC_PRESENTATION_REPRESENTATION('',(#214343),#55309);
#134814=CARTESIAN_POINT ( 'NONE',  ( 6.717278222822382183, -7.246166700180828535, -6.750415307812249743 ) ) ;
#134829=CARTESIAN_POINT ( 'NONE',  ( 0.4683205530892388113, -8.233137084989849086, 9.568546172724163412 ) ) ;
#134840=CARTESIAN_POINT ( 'NONE',  ( 6.783773251375732727, -6.684699875907444522, -6.634380621478984885 ) ) ;
#134915=CARTESIAN_POINT ( 'NONE',  ( -6.830415307812261361, -7.246166700180801001, -6.717278222822380407 ) ) ;
#134917=CARTESIAN_POINT ( 'NONE',  ( 10.67870335800436621, -6.148216694138044502, -1.725267604293023415E-15 ) ) ;
#134985=EDGE_CURVE ( 'NONE', #34393, #183422, #87314, .T. ) ;
#134995=ORIENTED_EDGE ( 'NONE', *, *, #13865, .T. ) ;
#135006=CYLINDRICAL_SURFACE ( 'NONE', #63191, 0.09999999999999990841 ) ;
#135017=CARTESIAN_POINT ( 'NONE',  ( 0.09916492693096318201, -10.00000000000016342, 9.499482423651661733 ) ) ;
#135027=EDGE_CURVE ( 'NONE', #183550, #148587, #107472, .T. ) ;
#135038=CARTESIAN_POINT ( 'NONE',  ( -7.796438949605438040, -6.657020681836948839, 7.586009164902152158 ) ) ;
#135064=CARTESIAN_POINT ( 'NONE',  ( -10.42871741020803000, 1.405922845961221412, 5.936700867306084817 ) ) ;
#135068=CARTESIAN_POINT ( 'NONE',  ( 0.4370932794886464023, -5.427673425445469491, 10.76345817711984409 ) ) ;
#135093=CARTESIAN_POINT ( 'NONE',  ( 9.481348452320371933, -9.006862915010128035, -0.5950054837411746789 ) ) ;
#135105=DIRECTION ( 'NONE',  ( 0.000000000000000000, 1.000000000000000000, 0.000000000000000000 ) ) ;
#135108=VERTEX_POINT ( 'NONE', #177744 ) ;
#135111=DIRECTION ( 'NONE',  ( -1.000000000000000000, 1.561251128379122346E-12, 0.000000000000000000 ) ) ;
#135128=ORIENTED_EDGE ( 'NONE', *, *, #18222, .T. ) ;
#135163=EDGE_CURVE ( 'NONE', #18033, #195316, #214114, .T. ) ;
#135165=PRODUCT_DEFINITION ( 'UNKNOWN', '', #83370, #33075 ) ;
#135168=B_SPLINE_CURVE_WITH_KNOTS ( 'NONE', 3,
 ( #106821, #125238, #140369, #191197, #42863, #108971, #4954, #71032, #113243, #30871 ),
 .UNSPECIFIED., .F., .F.,
 ( 4, 2, 2, 2, 4 ),
 ( 7.684844577824277550E-18, 0.0002021113321160356176, 0.0004042226642320635374, 0.0006063339963480915114, 0.0008084453284641193770 ),
 .UNSPECIFIED. ) ;
#135244=( BOUNDED_SURFACE ( )  B_SPLINE_SURFACE ( 3, 2, ( 
 ( #201018, #138200, #6020 ),
 ( #167487, #85162, #120951 ),
 ( #7087, #105716, #204211 ),
 ( #153369, #89452, #20145 ),
 ( #155505, #19082, #88373 ),
 ( #23342, #169614, #55863 ),
 ( #38552, #186922, #22264 ),
 ( #104630, #122020, #68887 ) ),
 .UNSPECIFIED., .F., .F., .F. ) 
 B_SPLINE_SURFACE_WITH_KNOTS ( ( 4, 2, 2, 4 ),
 ( 3, 3 ),
 ( -4.065758146820641628E-19, 0.0002475938981900014865, 0.0004951877963800034067, 0.0009903755927600072471 ),
 ( 0.000000000000000000, 1.000000000000000000 ),
 .UNSPECIFIED. ) 
 GEOMETRIC_REPRESENTATION_ITEM ( )  RATIONAL_B_SPLINE_SURFACE ( (
 ( 1.000000000000000000, 0.9238795325112891810, 1.000000000000000000),
 ( 1.000000000000000000, 0.9248499699752523728, 1.000000000000000000),
 ( 1.000000000000000000, 0.9171047238584710826, 1.000000000000000000),
 ( 1.000000000000000000, 0.8907236462368126606, 1.000000000000000000),
 ( 1.000000000000000000, 0.8725411758596960388, 1.000000000000000000),
 ( 1.000000000000000000, 0.8105159241138063519, 1.000000000000000000),
 ( 1.000000000000000000, 0.7599483315144157647, 1.000000000000000000),
 ( 1.000000000000000000, 0.7045118851637699464, 1.000000000000000000) ) ) 
 REPRESENTATION_ITEM ( '' )  SURFACE ( )  );
#135263=CARTESIAN_POINT ( 'NONE',  ( 0.000000000000000000, 4.006659545634088992, 0.000000000000000000 ) ) ;
#135322=( NAMED_UNIT ( * ) PLANE_ANGLE_UNIT ( ) SI_UNIT ( $, .RADIAN. ) );
#135345=FACE_OUTER_BOUND ( 'NONE', #189954, .T. ) ;
#135352=DIRECTION ( 'NONE',  ( 0.000000000000000000, 0.000000000000000000, -1.000000000000000000 ) ) ;
#135361=CARTESIAN_POINT ( 'NONE',  ( -7.142181811248260459E-15, -6.291672674598642878, 10.90688615205475465 ) ) ;
#135442=CARTESIAN_POINT ( 'NONE',  ( 9.499984059629561273, -7.809931833644721877, 0.02724524595756149317 ) ) ;
#135455=CARTESIAN_POINT ( 'NONE',  ( 1.408343819019454993E-15, 1.000000000000000888, 11.49999999999998934 ) ) ;
#135487=CARTESIAN_POINT ( 'NONE',  ( -7.100579091573052892, -6.583980363594996277, 6.484567079770450881 ) ) ;
#135489=CARTESIAN_POINT ( 'NONE',  ( -1.138412281109779656E-15, -6.027819618361853315, -10.79920600060117053 ) ) ;
#135527=ORIENTED_EDGE ( 'NONE', *, *, #73451, .F. ) ;
#135531=FACE_OUTER_BOUND ( 'NONE', #86742, .T. ) ;
#135544=CARTESIAN_POINT ( 'NONE',  ( 10.35465518852990741, -5.836144560139977955, -0.4365953560983623083 ) ) ;
#135572=CARTESIAN_POINT ( 'NONE',  ( -9.096228393767150422, 0.9691415390508330008, -7.669416753559259448 ) ) ;
#135574=AXIS2_PLACEMENT_3D ( 'NONE', #90492, #206345, #125193 ) ;
#135575=CARTESIAN_POINT ( 'NONE',  ( -7.679448064523687556, -6.453073674884586275, -7.727353211424378365 ) ) ;
#135601=ORIENTED_EDGE ( 'NONE', *, *, #109387, .F. ) ;
#135611=ORIENTED_EDGE ( 'NONE', *, *, #29409, .F. ) ;
#135617=EDGE_CURVE ( 'NONE', #90168, #184212, #202363, .T. ) ;
#135620=CARTESIAN_POINT ( 'NONE',  ( 0.2582262029270430137, -8.187798858731223817, 9.496816297611140101 ) ) ;
#135627=CARTESIAN_POINT ( 'NONE',  ( 9.499615238232420822, -9.906571760739462107, -0.08550182772145330234 ) ) ;
#135645=FACE_OUTER_BOUND ( 'NONE', #171365, .T. ) ;
#135663=ADVANCED_FACE ( 'NONE', ( #119183 ), #202476, .T. ) ;
#135683=VERTEX_POINT ( 'NONE', #102878 ) ;
#135685=ADVANCED_FACE ( 'NONE', ( #167875 ), #43135, .F. ) ;
#135687=LINE ( 'NONE', #86925, #158511 ) ;
#135708=EDGE_LOOP ( 'NONE', ( #107307, #124760, #150013, #19558 ) ) ;
#135757=ORIENTED_EDGE ( 'NONE', *, *, #113687, .T. ) ;
#135788=ORIENTED_EDGE ( 'NONE', *, *, #8812, .T. ) ;
#135808=AXIS2_PLACEMENT_3D ( 'NONE', #34851, #67334, #115123 ) ;
#135866=AXIS2_PLACEMENT_3D ( 'NONE', #170938, #122295, #56134 ) ;
#135884=CARTESIAN_POINT ( 'NONE',  ( 9.499700864329909678, -7.154544010627095219, 0.07538891330675548397 ) ) ;
#135901=CARTESIAN_POINT ( 'NONE',  ( -6.400381488218095605, -6.708819892820500286, -7.008396152629720710 ) ) ;
#135925=B_SPLINE_CURVE_WITH_KNOTS ( 'NONE', 3,
 ( #205689, #142877, #26938, #171065 ),
 .UNSPECIFIED., .F., .F.,
 ( 4, 4 ),
 ( 0.000000000000000000, 0.0002909236271752537947 ),
 .UNSPECIFIED. ) ;
#135948=VECTOR ( 'NONE', #1044, 1000.000000000000000 ) ;
#136046=( NAMED_UNIT ( * ) SI_UNIT ( $, .STERADIAN. ) SOLID_ANGLE_UNIT ( ) );
#136081=CARTESIAN_POINT ( 'NONE',  ( -9.617648866954029430, -9.063431457505044975, 0.6035590660249372519 ) ) ;
#136097=CARTESIAN_POINT ( 'NONE',  ( 3.223391908310548028E-14, -7.616807913963251409, -10.09384657274512165 ) ) ;
#136104=EDGE_CURVE ( 'NONE', #183752, #34907, #23741, .T. ) ;
#136119=EDGE_CURVE ( 'NONE', #209973, #133641, #171160, .T. ) ;
#136123=CARTESIAN_POINT ( 'NONE',  ( -10.91804383151480629, -9.900000000000005684, 0.1905751639681794174 ) ) ;
#136136=CARTESIAN_POINT ( 'NONE',  ( 10.96499746917716678, -5.350147675656132584, -0.1749484593404596611 ) ) ;
#136140=ORIENTED_EDGE ( 'NONE', *, *, #67115, .F. ) ;
#136146=B_SPLINE_CURVE_WITH_KNOTS ( 'NONE', 3,
 ( #204625, #57340, #190519, #56276 ),
 .UNSPECIFIED., .F., .F.,
 ( 4, 4 ),
 ( 0.000000000000000000, 0.0004065497138311778428 ),
 .UNSPECIFIED. ) ;
#136147=ORIENTED_EDGE ( 'NONE', *, *, #51899, .T. ) ;
#136154=PLANE ( 'NONE',  #33514 ) ;
#136158=ORIENTED_EDGE ( 'NONE', *, *, #183636, .T. ) ;
#136171=AXIS2_PLACEMENT_3D ( 'NONE', #130289, #213558, #62014 ) ;
#136187=AXIS2_PLACEMENT_3D ( 'NONE', #168134, #203804, #202740 ) ;
#136304=CARTESIAN_POINT ( 'NONE',  ( -9.531438498077104526, -8.057097448493919956, 0.1980946632349051273 ) ) ;
#136327=CARTESIAN_POINT ( 'NONE',  ( -1.138412281109779656E-15, -7.357813805514521910, -9.695354081530195955 ) ) ;
#136350=CARTESIAN_POINT ( 'NONE',  ( -7.726139724254740493, -6.443545996361842221, 7.681709917290615586 ) ) ;
#136375=DIRECTION ( 'NONE',  ( 1.000000000000000000, 2.168404344971003188E-14, 0.000000000000000000 ) ) ;
#136384=PRESENTATION_STYLE_ASSIGNMENT (( #17258 ) ) ;
#136386=CIRCLE ( 'NONE', #43011, 9.579999999999992966 ) ;
#136408=CARTESIAN_POINT ( 'NONE',  ( -0.09916492693109210665, -9.920000000000095852, -9.499482423651642193 ) ) ;
#136424=CARTESIAN_POINT ( 'NONE',  ( -0.08058608058608779379, -6.134628647623513231, 10.99970480893080804 ) ) ;
#136479=CIRCLE ( 'NONE', #126189, 11.99999999999999112 ) ;
#136511=CARTESIAN_POINT ( 'NONE',  ( 9.495732322661975644, -8.202835266173755357, -0.2934966634902085869 ) ) ;
#136518=COLOUR_RGB ( '', 0.66274510, 0.83137255, 0.94901961) ;
#136531=CARTESIAN_POINT ( 'NONE',  ( -11.41010744128099219, 2.630042260599918080, 3.716153451272427688 ) ) ;
#136536=AXIS2_PLACEMENT_3D ( 'NONE', #72585, #57418, #139762 ) ;
#136556=CARTESIAN_POINT ( 'NONE',  ( -6.743487189263854376, -7.020359948792041394, 6.692370362266554906 ) ) ;
#136578=ORIENTED_EDGE ( 'NONE', *, *, #65255, .T. ) ;
#136619=CARTESIAN_POINT ( 'NONE',  ( -10.87247189006428449, -6.708723052947955345, 0.1888596022590807721 ) ) ;
#136695=CARTESIAN_POINT ( 'NONE',  ( 9.499606442108964544, -9.901472054505708442, -0.08647222121513538362 ) ) ;
#136715=CARTESIAN_POINT ( 'NONE',  ( 6.447678837262253104, -6.532648880269189107, 6.949550370341235350 ) ) ;
#136746=CARTESIAN_POINT ( 'NONE',  ( -0.1000000000000028644, -9.999999999999994671, -9.579478065113972818 ) ) ;
#136774=ORIENTED_EDGE ( 'NONE', *, *, #87175, .F. ) ;
#136779=CARTESIAN_POINT ( 'NONE',  ( 0.000000000000000000, 0.03624871340549007392, 0.000000000000000000 ) ) ;
#136785=MECHANICAL_DESIGN_GEOMETRIC_PRESENTATION_REPRESENTATION('',(#22635),#129894);
#136794=B_SPLINE_CURVE_WITH_KNOTS ( 'NONE', 3,
 ( #85399, #119033, #16107, #131024, #3055, #918, #114768, #163465 ),
 .UNSPECIFIED., .F., .F.,
 ( 4, 2, 2, 4 ),
 ( 0.000000000000000000, 0.0005156231957999649930, 0.0007734347936999474895, 0.001031246391599929986 ),
 .UNSPECIFIED. ) ;
#136801=DIRECTION ( 'NONE',  ( 0.7431448254773955764, 0.000000000000000000, 0.6691306063588566833 ) ) ;
#136808=DIRECTION ( 'NONE',  ( 0.000000000000000000, 0.000000000000000000, -1.000000000000000000 ) ) ;
#136810=ORIENTED_EDGE ( 'NONE', *, *, #75639, .F. ) ;
#136845=CARTESIAN_POINT ( 'NONE',  ( -7.987977580929922716, -5.530730635397378414, -7.987977580929888077 ) ) ;
#136901=FILL_AREA_STYLE_COLOUR ( '', #97791 ) ;
#136943=CARTESIAN_POINT ( 'NONE',  ( -10.99967557777140925, -6.699439830718301181, 0.09581361862939005714 ) ) ;
#136964=ORIENTED_EDGE ( 'NONE', *, *, #152781, .T. ) ;
#136966=CARTESIAN_POINT ( 'NONE',  ( 7.721398836998394799, -5.907420853759296264, 7.721398836998372595 ) ) ;
#137034=CARTESIAN_POINT ( 'NONE',  ( -10.99387514841215463, -6.699757570937981299, 0.3793797362571516008 ) ) ;
#137099=VERTEX_POINT ( 'NONE', #40836 ) ;
#137106=DIRECTION ( 'NONE',  ( 0.000000000000000000, 0.000000000000000000, -1.000000000000000000 ) ) ;
#137110=ORIENTED_EDGE ( 'NONE', *, *, #63516, .F. ) ;
#137121=ADVANCED_FACE ( 'NONE', ( #110154 ), #131704, .F. ) ;
#137134=EDGE_CURVE ( 'NONE', #109006, #54631, #185204, .T. ) ;
#137160=EDGE_CURVE ( 'NONE', #19237, #19391, #133851, .T. ) ;
#137166=LINE ( 'NONE', #54836, #130944 ) ;
#137170=CARTESIAN_POINT ( 'NONE',  ( -10.39230484541327826, 3.447199233515649386, -5.999999999999975131 ) ) ;
#137199=CARTESIAN_POINT ( 'NONE',  ( 0.000000000000000000, 15.50000000000019362, 0.000000000000000000 ) ) ;
#137241=CARTESIAN_POINT ( 'NONE',  ( 11.41042268598792653, 3.467171072964057910, -3.707471073020402574 ) ) ;
#137244=AXIS2_PLACEMENT_3D ( 'NONE', #152034, #3605, #20926 ) ;
#137245=CARTESIAN_POINT ( 'NONE',  ( 10.91970695577495043, -5.907420853759282053, 8.673617379884035472E-15 ) ) ;
#137253=DIRECTION ( 'NONE',  ( 1.000000000000000000, 0.000000000000000000, 1.224646799147353207E-16 ) ) ;
#137286=AXIS2_PLACEMENT_3D ( 'NONE', #6373, #5289, #202431 ) ;
#137314=AXIS2_PLACEMENT_3D ( 'NONE', #134915, #117641, #18987 ) ;
#137317=CARTESIAN_POINT ( 'NONE',  ( 0.1309013025973270183, -5.411711732698802457, 10.96028113393447434 ) ) ;
#137352=CARTESIAN_POINT ( 'NONE',  ( 6.717278222822382183, 7.849261790823902629, -6.830415307812251591 ) ) ;
#137375=CARTESIAN_POINT ( 'NONE',  ( -9.495705940876565165, -8.203192640252289891, 0.2943368945748078280 ) ) ;
#137379=ORIENTED_EDGE ( 'NONE', *, *, #5161, .F. ) ;
#137383=FACE_OUTER_BOUND ( 'NONE', #10000, .T. ) ;
#137443=DIRECTION ( 'NONE',  ( 2.168462536859579677E-14, -1.000000000000000000, 9.418999208338882750E-28 ) ) ;
#137483=CARTESIAN_POINT ( 'NONE',  ( 0.000000000000000000, 0.000000000000000000, 10.99999999999999112 ) ) ;
#137491=CARTESIAN_POINT ( 'NONE',  ( 0.3811408430856297880, -6.893136995914741050, 10.99374989157288063 ) ) ;
#137509=DIRECTION ( 'NONE',  ( 0.6724985119639503850, 0.7071067811865539010, -0.2185080122244115464 ) ) ;
#137513=ORIENTED_EDGE ( 'NONE', *, *, #156758, .F. ) ;
#137531=FACE_OUTER_BOUND ( 'NONE', #156127, .T. ) ;
#137549=AXIS2_PLACEMENT_3D ( 'NONE', #183829, #134058, #150284 ) ;
#137554=ORIENTED_EDGE ( 'NONE', *, *, #70817, .T. ) ;
#137561=PLANE ( 'NONE',  #134318 ) ;
#137626=CARTESIAN_POINT ( 'NONE',  ( 7.893838479094925198, -5.325441678136449752, -7.661067326845484970 ) ) ;
#137628=CARTESIAN_POINT ( 'NONE',  ( -1.040834085586084257E-14, -7.246166700194011767, -9.579665964935651701 ) ) ;
#137650=CARTESIAN_POINT ( 'NONE',  ( 2.493954129951861720, 3.487142912321097299, -11.73313169142967460 ) ) ;
#137658=DIRECTION ( 'NONE',  ( 0.000000000000000000, 1.000000000000000000, 0.000000000000000000 ) ) ;
#137674=EDGE_CURVE ( 'NONE', #101925, #58795, #200910, .T. ) ;
#137681=CARTESIAN_POINT ( 'NONE',  ( 0.000000000000000000, -8.176568542494919711, 0.000000000000000000 ) ) ;
#137708=CARTESIAN_POINT ( 'NONE',  ( 10.91970695577495043, -6.134628647623513231, 5.204170427930421283E-15 ) ) ;
#137710=CARTESIAN_POINT ( 'NONE',  ( -7.547439985188169054, -6.717993526550385397, -7.827294160508111887 ) ) ;
#137711=STYLED_ITEM ( 'NONE', ( #97594 ), #203108 ) ;
#137753=ORIENTED_EDGE ( 'NONE', *, *, #77660, .F. ) ;
#137785=CARTESIAN_POINT ( 'NONE',  ( 0.1421055763938798289, -7.985988503423667062, 9.537847510268184337 ) ) ;
#137791=CARTESIAN_POINT ( 'NONE',  ( 0.000000000000000000, -5.199999999999996625, 0.000000000000000000 ) ) ;
#137819=CARTESIAN_POINT ( 'NONE',  ( 7.726139724254739605, -6.443545996361851103, -7.681709917290612921 ) ) ;
#137824=ORIENTED_EDGE ( 'NONE', *, *, #63903, .T. ) ;
#137861=COLOUR_RGB ( '', 0.08235294, 0.09019608, 0.10196078) ;
#137878=CARTESIAN_POINT ( 'NONE',  ( -1.138412281109779656E-15, -9.418601272600234608, 9.907592596884327918 ) ) ;
#137941=SURFACE_SIDE_STYLE ('',( #54543 ) ) ;
#137948=CARTESIAN_POINT ( 'NONE',  ( -6.662118508819848905, -7.185026885899485016, 6.772457744868685126 ) ) ;
#137950=AXIS2_PLACEMENT_3D ( 'NONE', #153930, #103043, #70503 ) ;
#137967=PRESENTATION_STYLE_ASSIGNMENT (( #19920 ) ) ;
#137968=EDGE_CURVE ( 'NONE', #137099, #206526, #82012, .T. ) ;
#137976=CARTESIAN_POINT ( 'NONE',  ( -10.99970480906932302, -5.741816521215535651, -0.08058606168007156900 ) ) ;
#137989=CARTESIAN_POINT ( 'NONE',  ( 10.99943592164173012, -9.900000000000019895, -0.1113975120799794716 ) ) ;
#138000=CARTESIAN_POINT ( 'NONE',  ( -0.008173644115966258172, -6.287979527546275982, -10.90726532705803820 ) ) ;
#138005=AXIS2_PLACEMENT_3D ( 'NONE', #187872, #166303, #39500 ) ;
#138009=CARTESIAN_POINT ( 'NONE',  ( -10.99970480893081870, -6.134628647623513231, -0.08058608058607828750 ) ) ;
#138024=EDGE_LOOP ( 'NONE', ( #197676, #13326, #4765, #173348 ) ) ;
#138037=FACE_OUTER_BOUND ( 'NONE', #202103, .T. ) ;
#138038=CARTESIAN_POINT ( 'NONE',  ( 6.875062624577638282, -8.049367966558001797, -6.605500049835221432 ) ) ;
#138046=CARTESIAN_POINT ( 'NONE',  ( 0.2633404184768576850, -6.747343053191802831, 9.488968570712993156 ) ) ;
#138088=ORIENTED_EDGE ( 'NONE', *, *, #65889, .T. ) ;
#138164=ADVANCED_FACE ( 'NONE', ( #165227 ), #112143, .T. ) ;
#138179=ORIENTED_EDGE ( 'NONE', *, *, #97346, .T. ) ;
#138182=CARTESIAN_POINT ( 'NONE',  ( -10.00050683067322765, 3.975933801733735340, 5.773795310721945739 ) ) ;
#138185=ORIENTED_EDGE ( 'NONE', *, *, #124333, .F. ) ;
#138199=CARTESIAN_POINT ( 'NONE',  ( -9.579665964948882007, -7.325744180092283564, 5.204170427930421283E-15 ) ) ;
#138200=CARTESIAN_POINT ( 'NONE',  ( 10.98194350564910415, -7.699999999999993072, -0.6300133639306324529 ) ) ;
#138232=DIRECTION ( 'NONE',  ( -0.01043841336116912988, 0.000000000000000000, -0.9999455182791217034 ) ) ;
#138266=CARTESIAN_POINT ( 'NONE',  ( 6.830415307812257808, -7.246166700180801001, 6.717278222822394618 ) ) ;
#138272=CARTESIAN_POINT ( 'NONE',  ( 2.400879090975676089, 3.975933801733734896, -11.29524806062144116 ) ) ;
#138291=DIRECTION ( 'NONE',  ( 0.000000000000000000, 0.000000000000000000, -1.000000000000000000 ) ) ;
#138301=CARTESIAN_POINT ( 'NONE',  ( -9.473215147174821382, -6.532648913094946330, 0.3561222683123355104 ) ) ;
#138364=CARTESIAN_POINT ( 'NONE',  ( -6.773846765317340868, -7.246166700180801001, -6.773846765317301788 ) ) ;
#138444=EDGE_LOOP ( 'NONE', ( #114129, #157312, #39236 ) ) ;
#138452=( BOUNDED_SURFACE ( )  B_SPLINE_SURFACE ( 3, 2, ( 
 ( #202360, #54010, #203426 ),
 ( #3089, #37760, #36677 ),
 ( #205578, #86506, #172036 ),
 ( #103833, #169881, #39905 ),
 ( #21471, #71295, #121230 ),
 ( #107092, #19356, #187200 ),
 ( #56146, #38828, #104912 ),
 ( #69160, #22552, #88658 ) ),
 .UNSPECIFIED., .F., .F., .T. ) 
 B_SPLINE_SURFACE_WITH_KNOTS ( ( 4, 2, 2, 4 ),
 ( 3, 3 ),
 ( 0.000000000000000000, 0.0002204160392919284333, 0.0004408320785838568665, 0.0008816641571677137331 ),
 ( 0.000000000000000000, 1.000000000000000000 ),
 .UNSPECIFIED. ) 
 GEOMETRIC_REPRESENTATION_ITEM ( )  RATIONAL_B_SPLINE_SURFACE ( (
 ( 1.000000000000000000, 0.4127341956165090364, 1.000000000000000000),
 ( 1.000000000000000000, 0.4103180386331816698, 1.000000000000000000),
 ( 1.000000000000000000, 0.4223234233957802730, 1.000000000000000000),
 ( 1.000000000000000000, 0.4613847219399360156, 1.000000000000000000),
 ( 1.000000000000000000, 0.4878744032655297769, 1.000000000000000000),
 ( 1.000000000000000000, 0.5702658980235773001, 1.000000000000000000),
 ( 1.000000000000000000, 0.6280001242509168913, 1.000000000000000000),
 ( 1.000000000000000000, 0.6787756258918240526, 1.000000000000000000) ) ) 
 REPRESENTATION_ITEM ( '' )  SURFACE ( )  );
#138455=PRESENTATION_STYLE_ASSIGNMENT (( #73428 ) ) ;
#138541=EDGE_LOOP ( 'NONE', ( #7151, #14458, #35793, #2797 ) ) ;
#138557=CIRCLE ( 'NONE', #62480, 10.99999999999999112 ) ;
#138560=CARTESIAN_POINT ( 'NONE',  ( -0.07933194154488883154, -9.746166700180788567, -9.499668754385620417 ) ) ;
#138568=CARTESIAN_POINT ( 'NONE',  ( -10.96384327792182134, -7.754568858751050620, 0.4817895937885991464 ) ) ;
#138574=( NAMED_UNIT ( * ) SI_UNIT ( $, .STERADIAN. ) SOLID_ANGLE_UNIT ( ) );
#138616=VERTEX_POINT ( 'NONE', #154316 ) ;
#138624=CARTESIAN_POINT ( 'NONE',  ( 0.000000000000000000, -0.9200000000000041478, 0.000000000000000000 ) ) ;
#138625=EDGE_CURVE ( 'NONE', #113056, #183752, #5370, .T. ) ;
#138653=CARTESIAN_POINT ( 'NONE',  ( 0.000000000000000000, -7.666862915010147717, 0.000000000000000000 ) ) ;
#138683=EDGE_CURVE ( 'NONE', #146171, #190376, #154161, .T. ) ;
#138709=ORIENTED_EDGE ( 'NONE', *, *, #11469, .T. ) ;
#138749=CARTESIAN_POINT ( 'NONE',  ( 9.521443730523927229, -8.144690279336728622, -0.3123298761244219790 ) ) ;
#138751=DIRECTION ( 'NONE',  ( 0.000000000000000000, 0.000000000000000000, 1.000000000000000000 ) ) ;
#138778=CARTESIAN_POINT ( 'NONE',  ( -7.721398836998401016, -6.134628647623487474, -7.721398836998358384 ) ) ;
#138810=CARTESIAN_POINT ( 'NONE',  ( 6.922777049148924000, -8.203199116536602276, -6.506163559800166141 ) ) ;
#138813=CARTESIAN_POINT ( 'NONE',  ( 9.499771961674738918, -7.051679281653861153, 0.06642998979260432424 ) ) ;
#138821=CARTESIAN_POINT ( 'NONE',  ( 0.000000000000000000, 3.499999999999989342, 0.000000000000000000 ) ) ;
#138830=AXIS2_PLACEMENT_3D ( 'NONE', #213011, #117731, #1746 ) ;
#138833=DIRECTION ( 'NONE',  ( 0.000000000000000000, 0.000000000000000000, 1.000000000000000000 ) ) ;
#138837=CARTESIAN_POINT ( 'NONE',  ( -9.586610838029432813, -7.161464053357567749, 0.003376046620578128550 ) ) ;
#138852=CARTESIAN_POINT ( 'NONE',  ( 0.3123298761244165389, -8.144690279336737504, 9.521443730523929005 ) ) ;
#138893=VERTEX_POINT ( 'NONE', #197468 ) ;
#138938=EDGE_CURVE ( 'NONE', #142721, #111346, #24825, .T. ) ;
#138944=ORIENTED_EDGE ( 'NONE', *, *, #160078, .F. ) ;
#138947=CARTESIAN_POINT ( 'NONE',  ( 0.000000000000000000, -13.99999999999999822, 0.000000000000000000 ) ) ;
#138951=CARTESIAN_POINT ( 'NONE',  ( -6.773846765307970585, -7.473374494058216300, 6.773846765307992790 ) ) ;
#138954=ORIENTED_EDGE ( 'NONE', *, *, #13614, .F. ) ;
#138956=CARTESIAN_POINT ( 'NONE',  ( 9.512045263456263555, -8.176568542494905500, -0.4655551865852067817 ) ) ;
#138965=ORIENTED_EDGE ( 'NONE', *, *, #191143, .T. ) ;
#138982=COLOUR_RGB ( '', 0.08235294, 0.09019608, 0.10196078) ;
#139012=VECTOR ( 'NONE', #118027, 1000.000000000000000 ) ;
#139036=DIRECTION ( 'NONE',  ( 0.6762880771785568790, 0.000000000000000000, 0.7366372490351884572 ) ) ;
#139060=CARTESIAN_POINT ( 'NONE',  ( -6.773376349083142678, -7.246166700180801001, -6.661184041420939117 ) ) ;
#139102=CARTESIAN_POINT ( 'NONE',  ( 7.772296586883624236, -5.601927612791787858, 7.784592198500461357 ) ) ;
#139112=CYLINDRICAL_SURFACE ( 'NONE', #75228, 9.499999999999992895 ) ;
#139118=AXIS2_PLACEMENT_3D ( 'NONE', #154963, #72626, #48156 ) ;
#139244=ORIENTED_EDGE ( 'NONE', *, *, #100257, .T. ) ;
#139247=CARTESIAN_POINT ( 'NONE',  ( -10.30923643716943872, 0.9706168436483918471, 5.952040432139342307 ) ) ;
#139265=CARTESIAN_POINT ( 'NONE',  ( 0.000000000000000000, 3.499999999999989342, 0.000000000000000000 ) ) ;
#139312=CARTESIAN_POINT ( 'NONE',  ( -0.4694063952341946955, -6.893137084989842123, -10.98997987423602751 ) ) ;
#139332=CARTESIAN_POINT ( 'NONE',  ( -10.39230484541323740, 3.447199233515621408, 6.000000000000048850 ) ) ;
#139348=EDGE_LOOP ( 'NONE', ( #27683, #129031, #148546, #98698 ) ) ;
#139362=CARTESIAN_POINT ( 'NONE',  ( 0.000000000000000000, 0.000000000000000000, 0.000000000000000000 ) ) ;
#139373=DIRECTION ( 'NONE',  ( 0.000000000000000000, 0.000000000000000000, 1.000000000000000000 ) ) ;
#139408=ORIENTED_EDGE ( 'NONE', *, *, #41681, .F. ) ;
#139434=CARTESIAN_POINT ( 'NONE',  ( 0.001932293024931841172, -9.922538603026485049, 10.91970414279959378 ) ) ;
#139435=ORIENTED_EDGE ( 'NONE', *, *, #104201, .T. ) ;
#139489=FILL_AREA_STYLE ('',( #92876 ) ) ;
#139509=VERTEX_POINT ( 'NONE', #1382 ) ;
#139517=ORIENTED_EDGE ( 'NONE', *, *, #59579, .F. ) ;
#139560=CARTESIAN_POINT ( 'NONE',  ( -9.499606442108964544, -9.746166700193986898, 0.08647222121513808979 ) ) ;
#139563=CARTESIAN_POINT ( 'NONE',  ( -0.3656762941044116033, -7.723177556212100114, 10.97096416026169052 ) ) ;
#139592=VECTOR ( 'NONE', #107501, 1000.000000000000000 ) ;
#139623=CARTESIAN_POINT ( 'NONE',  ( 8.103009739378183696, -6.700000000000002842, -7.439168848973796599 ) ) ;
#139632=EDGE_CURVE ( 'NONE', #12663, #10241, #95436, .T. ) ;
#139678=AXIS2_PLACEMENT_3D ( 'NONE', #58848, #92451, #23118 ) ;
#139694=DIRECTION ( 'NONE',  ( 0.000000000000000000, 3.252606517456504467E-14, -1.000000000000000000 ) ) ;
#139720=B_SPLINE_CURVE_WITH_KNOTS ( 'NONE', 3,
 ( #140603, #205542, #105978, #189305, #173077, #124400, #190358, #42020 ),
 .UNSPECIFIED., .F., .F.,
 ( 4, 2, 2, 4 ),
 ( 0.000000000000000000, 0.0004970278158210322947, 0.0007455417237315461109, 0.0009940556316420600357 ),
 .UNSPECIFIED. ) ;
#139737=LINE ( 'NONE', #104018, #108138 ) ;
#139743=DIRECTION ( 'NONE',  ( -0.000000000000000000, -1.000000000000000000, -0.000000000000000000 ) ) ;
#139744=TOROIDAL_SURFACE ( 'NONE', #115642, 9.580000000000003624, 0.08000000000000000167 ) ;
#139762=DIRECTION ( 'NONE',  ( 0.000000000000000000, 0.000000000000000000, -1.000000000000000000 ) ) ;
#139769=CARTESIAN_POINT ( 'NONE',  ( 0.000000000000000000, 1.000000000000000888, 8.049999999999993605 ) ) ;
#139788=EDGE_LOOP ( 'NONE', ( #128592, #143941, #181212, #51106 ) ) ;
#139792=CARTESIAN_POINT ( 'NONE',  ( 0.000000000000000000, -9.999999999999994671, 0.000000000000000000 ) ) ;
#139810=CARTESIAN_POINT ( 'NONE',  ( -7.770158002573702483, -5.767087321559040802, 7.786489011996849285 ) ) ;
#139824=CARTESIAN_POINT ( 'NONE',  ( -10.04733898909035794, 1.529612873802629780, -6.247711339171014622 ) ) ;
#139844=ORIENTED_EDGE ( 'NONE', *, *, #165066, .T. ) ;
#139853=FACE_OUTER_BOUND ( 'NONE', #180271, .T. ) ;
#139860=DIRECTION ( 'NONE',  ( -0.9998476951563912696, 0.000000000000000000, 0.01745240643728004568 ) ) ;
#139862=EDGE_CURVE ( 'NONE', #116385, #142909, #4095, .T. ) ;
#139878=VERTEX_POINT ( 'NONE', #103185 ) ;
#139891=ORIENTED_EDGE ( 'NONE', *, *, #207315, .F. ) ;
#139921=( BOUNDED_SURFACE ( )  B_SPLINE_SURFACE ( 3, 2, ( 
 ( #165930, #69467, #135572 ),
 ( #184293, #20717, #168062 ),
 ( #35918, #87878, #117238 ),
 ( #182158, #68401, #101994 ) ),
 .UNSPECIFIED., .F., .F., .F. ) 
 B_SPLINE_SURFACE_WITH_KNOTS ( ( 4, 4 ),
 ( 3, 3 ),
 ( 0.005313560486515473899, 0.008339948430246690511 ),
 ( 0.000000000000000000, 1.000000000000000000 ),
 .UNSPECIFIED. ) 
 GEOMETRIC_REPRESENTATION_ITEM ( )  RATIONAL_B_SPLINE_SURFACE ( (
 ( 1.000000000000000000, 0.7184380228464071205, 1.000000000000000000),
 ( 1.000000000000000000, 0.7185467277397555863, 1.000000000000000000),
 ( 1.000000000000000000, 0.7186585579881037411, 1.000000000000000000),
 ( 1.000000000000000000, 0.7187737999613683648, 1.000000000000000000) ) ) 
 REPRESENTATION_ITEM ( '' )  SURFACE ( )  );
#139968=CIRCLE ( 'NONE', #122722, 9.499999999999991118 ) ;
#140022=CYLINDRICAL_SURFACE ( 'NONE', #59169, 6.249999999999995559 ) ;
#140026=( LENGTH_UNIT ( ) NAMED_UNIT ( * ) SI_UNIT ( .MILLI., .METRE. ) );
#140082=DIRECTION ( 'NONE',  ( 0.000000000000000000, 0.000000000000000000, 1.000000000000000000 ) ) ;
#140127=CARTESIAN_POINT ( 'NONE',  ( -11.00029519899100450, -5.907420853759283830, 6.708500942254059474E-15 ) ) ;
#140175=ORIENTED_EDGE ( 'NONE', *, *, #124443, .T. ) ;
#140186=CARTESIAN_POINT ( 'NONE',  ( 7.717216217110708598, -5.600320323339623485, 7.761717428875256175 ) ) ;
#140199=CARTESIAN_POINT ( 'NONE',  ( 0.09872732973948897262, -6.896119493545150192, 9.497255425109711879 ) ) ;
#140210=TOROIDAL_SURFACE ( 'NONE', #50348, 10.92000000000000171, 0.08000000000000000167 ) ;
#140241=VECTOR ( 'NONE', #104166, 1000.000000000000000 ) ;
#140317=CARTESIAN_POINT ( 'NONE',  ( -0.09630943990284260292, -9.919512026728389387, -10.99957837791001225 ) ) ;
#140352=CARTESIAN_POINT ( 'NONE',  ( -9.499750697158754420, -9.920000000031521381, 0.06885943948997631792 ) ) ;
#140369=CARTESIAN_POINT ( 'NONE',  ( 11.31269326259041108, 3.603011019375353730, -3.682594235848559716 ) ) ;
#140374=CARTESIAN_POINT ( 'NONE',  ( -7.407835137441776574, -5.166862915010159263, -8.023115266309144289 ) ) ;
#140404=DIRECTION ( 'NONE',  ( -0.7071067811865462405, 0.000000000000000000, 0.7071067811865489050 ) ) ;
#140413=ORIENTED_EDGE ( 'NONE', *, *, #17921, .F. ) ;
#140442=EDGE_CURVE ( 'NONE', #169714, #80718, #119730, .T. ) ;
#140466=CARTESIAN_POINT ( 'NONE',  ( -0.1515253745957804432, 3.870538056096192836, 11.62858902121511839 ) ) ;
#140504=CARTESIAN_POINT ( 'NONE',  ( -7.037870247915956945, -8.233137084989836652, 6.381095703207982694 ) ) ;
#140603=CARTESIAN_POINT ( 'NONE',  ( -10.99943592164172834, -8.407420853759269619, 0.1113975120798846308 ) ) ;
#140610=SURFACE_STYLE_USAGE ( .BOTH. , #107059 ) ;
#140637=B_SPLINE_CURVE_WITH_KNOTS ( 'NONE', 3,
 ( #1055, #119158, #185142, #120239, #19449, #70317, #3181 ),
 .UNSPECIFIED., .F., .F.,
 ( 4, 3, 4 ),
 ( 0.0001135037246152890099, 0.0006245292469112829472, 0.002007692286193829209 ),
 .UNSPECIFIED. ) ;
#140688=CARTESIAN_POINT ( 'NONE',  ( 7.680942717881078075, -5.294771359305314284, 7.874499448206171870 ) ) ;
#140695=DIRECTION ( 'NONE',  ( 3.552713678800500929E-15, 0.000000000000000000, 1.000000000000000000 ) ) ;
#140720=CARTESIAN_POINT ( 'NONE',  ( -0.3870405448657274761, 1.264806443676224079, 11.85654951141428981 ) ) ;
#140729=STYLED_ITEM ( 'NONE', ( #150639 ), #144182 ) ;
#140759=CARTESIAN_POINT ( 'NONE',  ( 6.844806938814767427, -6.074287852078585459, 7.461813752226492014 ) ) ;
#140793=B_SPLINE_CURVE_WITH_KNOTS ( 'NONE', 3,
 ( #140504, #174059, #155651, #204359, #22417, #88526, #25631, #72234 ),
 .UNSPECIFIED., .F., .F.,
 ( 4, 2, 2, 4 ),
 ( 0.000000000000000000, 0.0002567066673176306157, 0.0005134133346352612315, 0.001026826669270521596 ),
 .UNSPECIFIED. ) ;
#140817=CARTESIAN_POINT ( 'NONE',  ( 0.000000000000000000, -6.836568542494925182, 0.000000000000000000 ) ) ;
#140838=EDGE_CURVE ( 'NONE', #40383, #163622, #71250, .T. ) ;
#140868=ORIENTED_EDGE ( 'NONE', *, *, #18861, .T. ) ;
#140872=EDGE_CURVE ( 'NONE', #72330, #71109, #126709, .T. ) ;
#140878=CARTESIAN_POINT ( 'NONE',  ( -0.005973655271646400276, -7.189371949516665694, -9.500370076773238637 ) ) ;
#140889=AXIS2_PLACEMENT_3D ( 'NONE', #134380, #1115, #69310 ) ;
#140906=CARTESIAN_POINT ( 'NONE',  ( -9.871989323747691003, 3.235871879154613051, -6.146221223954435153 ) ) ;
#140911=CARTESIAN_POINT ( 'NONE',  ( -9.561191386655703894, -9.006862915010128035, 0.6000160562358372029 ) ) ;
#140961=EDGE_CURVE ( 'NONE', #207870, #21223, #164129, .T. ) ;
#140970=( BOUNDED_SURFACE ( )  B_SPLINE_SURFACE ( 3, 2, ( 
 ( #36643, #52900, #167722 ),
 ( #115832, #200197, #119034 ),
 ( #51850, #168784, #181818 ),
 ( #20389, #86473, #152537 ),
 ( #136304, #186092, #103801 ),
 ( #169850, #21438, #137375 ),
 ( #75560, #171998, #22513 ),
 ( #7333, #125459, #90763 ) ),
 .UNSPECIFIED., .F., .F., .F. ) 
 B_SPLINE_SURFACE_WITH_KNOTS ( ( 4, 2, 2, 4 ),
 ( 3, 3 ),
 ( 5.421010862427522170E-20, 0.0005123566476021758223, 0.0007685349714032637877, 0.001024713295204351645 ),
 ( 0.000000000000000000, 1.000000000000000000 ),
 .UNSPECIFIED. ) 
 GEOMETRIC_REPRESENTATION_ITEM ( )  RATIONAL_B_SPLINE_SURFACE ( (
 ( 1.000000000000000000, 0.7100530722026819896, 1.000000000000000000),
 ( 1.000000000000000000, 0.7667719522827127765, 1.000000000000000000),
 ( 1.000000000000000000, 0.8160440554223272747, 1.000000000000000000),
 ( 1.000000000000000000, 0.8737249316769533092, 1.000000000000000000),
 ( 1.000000000000000000, 0.8903164784318444713, 1.000000000000000000),
 ( 1.000000000000000000, 0.9150853305242792057, 1.000000000000000000),
 ( 1.000000000000000000, 0.9227739504731496956, 1.000000000000000000),
 ( 1.000000000000000000, 0.9238795325112855172, 1.000000000000000000) ) ) 
 REPRESENTATION_ITEM ( '' )  SURFACE ( )  );
#140982=CARTESIAN_POINT ( 'NONE',  ( -10.99873804690111356, -8.265528217051425486, 0.1803058380984418063 ) ) ;
#140994=DIRECTION ( 'NONE',  ( 0.000000000000000000, -1.000000000000000000, 0.000000000000000000 ) ) ;
#141003=ADVANCED_FACE ( 'NONE', ( #13592 ), #61287, .T. ) ;
#141011=DIRECTION ( 'NONE',  ( 0.6716942845482061220, 0.000000000000000000, 0.7408284471490504952 ) ) ;
#141047=CARTESIAN_POINT ( 'NONE',  ( 7.721398836998350390, -5.907420853759296264, -7.721398836998385917 ) ) ;
#141048=CIRCLE ( 'NONE', #47639, 0.07999999999999984901 ) ;
#141111=SURFACE_STYLE_USAGE ( .BOTH. , #90200 ) ;
#141120=ORIENTED_EDGE ( 'NONE', *, *, #145267, .F. ) ;
#141125=ORIENTED_EDGE ( 'NONE', *, *, #50663, .F. ) ;
#141144=ORIENTED_EDGE ( 'NONE', *, *, #5382, .T. ) ;
#141163=ORIENTED_EDGE ( 'NONE', *, *, #28627, .T. ) ;
#141206=FILL_AREA_STYLE ('',( #114847 ) ) ;
#141222=AXIS2_PLACEMENT_3D ( 'NONE', #134335, #33596, #118116 ) ;
#141269=DIRECTION ( 'NONE',  ( 0.000000000000000000, 1.000000000000000000, 0.000000000000000000 ) ) ;
#141292=CIRCLE ( 'NONE', #89307, 0.08000000000000040412 ) ;
#141296=CARTESIAN_POINT ( 'NONE',  ( 0.08058608058607655278, -9.902238891812018551, 10.99970480893082225 ) ) ;
#141329=ORIENTED_EDGE ( 'NONE', *, *, #166507, .T. ) ;
#141343=CARTESIAN_POINT ( 'NONE',  ( -2.450294804887450884, 1.972237431424518794, 11.52773071619796497 ) ) ;
#141358=CARTESIAN_POINT ( 'NONE',  ( -9.586610838029429260, -7.161464053357574855, 0.003376046620574835178 ) ) ;
#141433=CARTESIAN_POINT ( 'NONE',  ( -9.499766273075884726, -9.919999999999998153, 0.06663900456894793212 ) ) ;
#141483=B_SPLINE_CURVE_WITH_KNOTS ( 'NONE', 3,
 ( #109850, #175864, #163613, #34651 ),
 .UNSPECIFIED., .F., .F.,
 ( 4, 4 ),
 ( 4.336808689941991736E-19, 6.033646489354566999E-05 ),
 .UNSPECIFIED. ) ;
#141485=CARTESIAN_POINT ( 'NONE',  ( 8.830779531597181986, 3.974415841077565403, 7.430925027917878900 ) ) ;
#141572=ORIENTED_EDGE ( 'NONE', *, *, #194669, .T. ) ;
#141596=CARTESIAN_POINT ( 'NONE',  ( 0.04699017840226540899, -9.984793624843945281, 10.91963405940079568 ) ) ;
#141652=CARTESIAN_POINT ( 'NONE',  ( -0.4382560683119304801, -7.666862915010147717, 10.99126615174920119 ) ) ;
#141657=CARTESIAN_POINT ( 'NONE',  ( -6.908358566921340760, -6.724344753046663570, 6.684387857553240941 ) ) ;
#141682=CARTESIAN_POINT ( 'NONE',  ( -9.579665964948882007, -7.473374494045003757, 5.204170427930421283E-15 ) ) ;
#141726=CARTESIAN_POINT ( 'NONE',  ( -9.529120656610874963E-19, -8.332912386296857932, 10.92578969873750161 ) ) ;
#141752=CARTESIAN_POINT ( 'NONE',  ( 0.000000000000000000, -6.532648833121157850, 0.000000000000000000 ) ) ;
#141780=CARTESIAN_POINT ( 'NONE',  ( 9.492905263954437345, -8.233136995002492853, -0.3773006915670611416 ) ) ;
#141802=FILL_AREA_STYLE ('',( #206746 ) ) ;
#141809=CARTESIAN_POINT ( 'NONE',  ( -6.784764760059077915, -8.039737506397905520, 6.649736275991423362 ) ) ;
#141825=ORIENTED_EDGE ( 'NONE', *, *, #188097, .T. ) ;
#141841=CARTESIAN_POINT ( 'NONE',  ( -0.05503291520805722592, -6.406027784105811307, 11.00000000000011902 ) ) ;
#141845=DIRECTION ( 'NONE',  ( 0.000000000000000000, 0.000000000000000000, 1.000000000000000000 ) ) ;
#141912=CARTESIAN_POINT ( 'NONE',  ( 0.000000000000000000, -1.000000000000000888, 0.000000000000000000 ) ) ;
#141943=ORIENTED_EDGE ( 'NONE', *, *, #213278, .F. ) ;
#141978=CARTESIAN_POINT ( 'NONE',  ( -7.721398836998398352, -5.907420853759296264, -7.721398836998357496 ) ) ;
#141997=CARTESIAN_POINT ( 'NONE',  ( -7.987977580929896071, -5.530730635397370420, 7.987977580929924493 ) ) ;
#142006=DIRECTION ( 'NONE',  ( 0.9989735196462989908, 1.504112749676232550E-16, -0.04529798058948674572 ) ) ;
#142032=DIRECTION ( 'NONE',  ( 0.000000000000000000, 0.000000000000000000, 1.000000000000000000 ) ) ;
#142038=CARTESIAN_POINT ( 'NONE',  ( -10.96075698767256767, -7.841077028191815401, 0.3746540212968124117 ) ) ;
#142114=CARTESIAN_POINT ( 'NONE',  ( 0.000000000000000000, -5.166862915010145052, 0.000000000000000000 ) ) ;
#142134=ORIENTED_EDGE ( 'NONE', *, *, #78480, .F. ) ;
#142144=DIRECTION ( 'NONE',  ( 0.000000000000000000, 1.000000000000000000, 0.000000000000000000 ) ) ;
#142148=ORIENTED_EDGE ( 'NONE', *, *, #168717, .F. ) ;
#142193=EDGE_CURVE ( 'NONE', #51705, #36647, #26427, .T. ) ;
#142215=ORIENTED_EDGE ( 'NONE', *, *, #207501, .T. ) ;
#142230=CARTESIAN_POINT ( 'NONE',  ( 0.000000000000000000, 3.079999999999999183, 0.000000000000000000 ) ) ;
#142249=DIRECTION ( 'NONE',  ( -0.000000000000000000, -1.000000000000000000, -0.000000000000000000 ) ) ;
#142251=CARTESIAN_POINT ( 'NONE',  ( -0.02890330888918044711, -9.971207602185762298, -10.91966316483285304 ) ) ;
#142284=CARTESIAN_POINT ( 'NONE',  ( 0.3387883092347047653, -5.166862915010296042, 10.99523224158955870 ) ) ;
#142285=ORIENTED_EDGE ( 'NONE', *, *, #46711, .F. ) ;
#142322=CARTESIAN_POINT ( 'NONE',  ( 6.901817412891589676, -6.554751173179806045, -6.500815856195342413 ) ) ;
#142327=CARTESIAN_POINT ( 'NONE',  ( 7.499070966595098753, -5.223177556212323935, 8.016215341155817242 ) ) ;
#142394=AXIS2_PLACEMENT_3D ( 'NONE', #118052, #36719, #84414 ) ;
#142401=CARTESIAN_POINT ( 'NONE',  ( -2.069187086148977173, 1.970899860167975914, 11.59589854942345077 ) ) ;
#142410=( LENGTH_UNIT ( ) NAMED_UNIT ( * ) SI_UNIT ( .MILLI., .METRE. ) );
#142452=CARTESIAN_POINT ( 'NONE',  ( -0.08500055850267987378, -9.912493587006867557, -10.99967158169069847 ) ) ;
#142472=ORIENTED_EDGE ( 'NONE', *, *, #208381, .T. ) ;
#142549=VECTOR ( 'NONE', #59035, 1000.000000000000000 ) ;
#142579=CARTESIAN_POINT ( 'NONE',  ( -9.003941998343226207E-15, -6.291672674598899562, -10.90688615205694845 ) ) ;
#142582=LINE ( 'NONE', #208589, #203413 ) ;
#142590=ORIENTED_EDGE ( 'NONE', *, *, #25220, .F. ) ;
#142601=CARTESIAN_POINT ( 'NONE',  ( 0.000000000000000000, -6.134628647623513231, 10.91970695577495931 ) ) ;
#142625=CARTESIAN_POINT ( 'NONE',  ( -8.917737905728749581, 3.447199233515649386, -8.029567276306266876 ) ) ;
#142637=CIRCLE ( 'NONE', #49230, 0.07999999999999951594 ) ;
#142652=ORIENTED_EDGE ( 'NONE', *, *, #164009, .F. ) ;
#142675=UNCERTAINTY_MEASURE_WITH_UNIT (LENGTH_MEASURE( 1.000000000000000082E-05 ), #178473, 'distance_accuracy_value', 'NONE');
#142676=CARTESIAN_POINT ( 'NONE',  ( 6.956180625287912811, -6.372104534815299814, 6.956180625285773189 ) ) ;
#142706=TOROIDAL_SURFACE ( 'NONE', #194459, 9.559451093910105612, 0.08000000000000000167 ) ;
#142721=VERTEX_POINT ( 'NONE', #10471 ) ;
#142776=( NAMED_UNIT ( * ) PLANE_ANGLE_UNIT ( ) SI_UNIT ( $, .RADIAN. ) );
#142814=ADVANCED_FACE ( 'NONE', ( #193505 ), #77615, .T. ) ;
#142839=CARTESIAN_POINT ( 'NONE',  ( 9.499668754586233277, -7.643695121331843367, 0.07933191752450531598 ) ) ;
#142843=CARTESIAN_POINT ( 'NONE',  ( 10.99934730582667797, -5.294005300192715424, -0.1376907581457621488 ) ) ;
#142844=DIRECTION ( 'NONE',  ( 0.7071067811865489050, 0.000000000000000000, 0.7071067811865462405 ) ) ;
#142866=AXIS2_PLACEMENT_3D ( 'NONE', #209183, #60823, #37920 ) ;
#142877=CARTESIAN_POINT ( 'NONE',  ( 10.23541933785883806, 1.000000000000000888, 6.134053304049035482 ) ) ;
#142886=CARTESIAN_POINT ( 'NONE',  ( 0.3610206255357477079, -7.699789852011537761, -10.99434576733086111 ) ) ;
#142909=VERTEX_POINT ( 'NONE', #192418 ) ;
#142945=CARTESIAN_POINT ( 'NONE',  ( -0.4294077647110545737, -6.532648833121157850, -9.469892045836658667 ) ) ;
#142959=CARTESIAN_POINT ( 'NONE',  ( -8.902524791715885399, 3.162178953954597471, -7.495381307383191860 ) ) ;
#142972=FILL_AREA_STYLE_COLOUR ( '', #32781 ) ;
#142977=CARTESIAN_POINT ( 'NONE',  ( -9.568546172724161636, -8.233137084989836652, 0.4683205530892458057 ) ) ;
#143030=EDGE_CURVE ( 'NONE', #41517, #182554, #126875, .T. ) ;
#143031=AXIS2_PLACEMENT_3D ( 'NONE', #123407, #137443, #136375 ) ;
#143040=CARTESIAN_POINT ( 'NONE',  ( -10.10176665042269839, 1.000000000000000888, -6.279211784079198999 ) ) ;
#143049=CARTESIAN_POINT ( 'NONE',  ( -6.773846765317340868, -7.246166700180801001, -6.773846765317301788 ) ) ;
#143068=CARTESIAN_POINT ( 'NONE',  ( -8.762124912781128927, 3.934209603697779389, -7.549522310265974312 ) ) ;
#143071=CARTESIAN_POINT ( 'NONE',  ( 7.548736465707318821, -7.034525073441744603, 7.548736465708006271 ) ) ;
#143079=CARTESIAN_POINT ( 'NONE',  ( -10.91962425643199808, -9.999999999999994671, 0.09058751758333691284 ) ) ;
#143104=CARTESIAN_POINT ( 'NONE',  ( 0.02191154088442351378, -9.962467531990274239, 9.579628365760351372 ) ) ;
#143108=AXIS2_PLACEMENT_3D ( 'NONE', #68788, #36300, #119763 ) ;
#143126=CARTESIAN_POINT ( 'NONE',  ( -10.99945475518247484, -9.908704762181759662, 0.1095286008944308248 ) ) ;
#143132=EDGE_CURVE ( 'NONE', #97798, #401, #33383, .T. ) ;
#143150=EDGE_CURVE ( 'NONE', #184212, #138616, #128596, .T. ) ;
#143183=CARTESIAN_POINT ( 'NONE',  ( -7.721398836998399240, -5.907420853759296264, -7.721398836998356607 ) ) ;
#143223=CARTESIAN_POINT ( 'NONE',  ( 0.000000000000000000, -6.134628647623513231, 10.91970695577495931 ) ) ;
#143237=CARTESIAN_POINT ( 'NONE',  ( 9.578206935409037115, -9.746166700193986898, -0.1671882239534273895 ) ) ;
#143273=EDGE_CURVE ( 'NONE', #114068, #204013, #130423, .T. ) ;
#143322=CIRCLE ( 'NONE', #32565, 0.08000000000000020983 ) ;
#143329=CIRCLE ( 'NONE', #160442, 9.616019636405020776 ) ;
#143353=CARTESIAN_POINT ( 'NONE',  ( -10.91970695577495398, -6.134628647623513231, -0.07999999999999153621 ) ) ;
#143387=ORIENTED_EDGE ( 'NONE', *, *, #140872, .F. ) ;
#143392=CARTESIAN_POINT ( 'NONE',  ( 7.057683771862822475, -6.583723166013057515, -6.531918710724782251 ) ) ;
#143397=CARTESIAN_POINT ( 'NONE',  ( 0.000000000000000000, -5.166862915010159263, 0.000000000000000000 ) ) ;
#143447=CARTESIAN_POINT ( 'NONE',  ( -7.341412881700131621, -6.244189044378193110, 6.724721492623497276 ) ) ;
#143473=VECTOR ( 'NONE', #40258, 1000.000000000000114 ) ;
#143567=ADVANCED_FACE ( 'NONE', ( #103458 ), #77872, .T. ) ;
#143601=DIRECTION ( 'NONE',  ( 0.000000000000000000, 0.000000000000000000, 1.000000000000000000 ) ) ;
#143625=CARTESIAN_POINT ( 'NONE',  ( -10.91970695577496997, -5.907420853759282053, 5.204170427930421283E-15 ) ) ;
#143642=FACE_OUTER_BOUND ( 'NONE', #109429, .T. ) ;
#143658=VERTEX_POINT ( 'NONE', #172739 ) ;
#143671=ORIENTED_EDGE ( 'NONE', *, *, #33554, .T. ) ;
#143677=CARTESIAN_POINT ( 'NONE',  ( 0.000000000000000000, 3.799999999999998046, 0.000000000000000000 ) ) ;
#143685=CARTESIAN_POINT ( 'NONE',  ( -1.040834085586084257E-14, -6.796015482748913428, 10.25773349932951461 ) ) ;
#143708=CARTESIAN_POINT ( 'NONE',  ( -8.917737905728749581, 3.038492715500545671, -8.029567276306263324 ) ) ;
#143757=CARTESIAN_POINT ( 'NONE',  ( 7.453913518772580460, -5.212532583863424662, 8.072398248062489401 ) ) ;
#143796=EDGE_CURVE ( 'NONE', #147554, #72330, #23154, .T. ) ;
#143798=EDGE_LOOP ( 'NONE', ( #45592, #74361, #23550, #52219 ) ) ;
#143812=DIRECTION ( 'NONE',  ( 0.000000000000000000, 0.000000000000000000, -1.000000000000000000 ) ) ;
#143891=CARTESIAN_POINT ( 'NONE',  ( 7.779015489124649463, -5.502990254781787272, 7.777446446097295407 ) ) ;
#143897=CARTESIAN_POINT ( 'NONE',  ( 0.000000000000000000, -9.919999999999998153, 0.000000000000000000 ) ) ;
#143899=B_SPLINE_CURVE_WITH_KNOTS ( 'NONE', 3,
 ( #121878, #192114, #9112, #10174, #24271, #40562, #191048 ),
 .UNSPECIFIED., .F., .F.,
 ( 4, 3, 4 ),
 ( 3.315837474970910530E-05, 0.0009000000035470257127, 0.001929259801299068556 ),
 .UNSPECIFIED. ) ;
#143914=CARTESIAN_POINT ( 'NONE',  ( 9.500338091956020747, -7.818966704647656307, 0.03919461954078456989 ) ) ;
#143920=CONICAL_SURFACE ( 'NONE', #206177, 10.99999999999998934, 0.7853981633974533860 ) ;
#143939=FACE_OUTER_BOUND ( 'NONE', #149447, .T. ) ;
#143941=ORIENTED_EDGE ( 'NONE', *, *, #12956, .F. ) ;
#143958=CARTESIAN_POINT ( 'NONE',  ( 0.1645940602202164704, -7.825441678136432877, -10.99897937609837761 ) ) ;
#143963=TOROIDAL_SURFACE ( 'NONE', #71222, 9.580000000000001847, 0.08000000000000000167 ) ;
#143975=CARTESIAN_POINT ( 'NONE',  ( 0.4358566159019752195, -8.896924251528579575, -9.793384314894453269 ) ) ;
#143979=CARTESIAN_POINT ( 'NONE',  ( -11.68720892159070601, 1.016282880930321930, 3.797404372613820911 ) ) ;
#143982=ORIENTED_EDGE ( 'NONE', *, *, #126069, .F. ) ;
#144021=CARTESIAN_POINT ( 'NONE',  ( 0.000000000000000000, 0.7999999999999951594, 0.000000000000000000 ) ) ;
#144047=FACE_OUTER_BOUND ( 'NONE', #15928, .T. ) ;
#144053=CARTESIAN_POINT ( 'NONE',  ( -10.14641618983896976, 3.870538056096199497, 5.683069686889705707 ) ) ;
#144062=CARTESIAN_POINT ( 'NONE',  ( 0.01138762994429960880, -7.792108994756127061, 9.500479199177402023 ) ) ;
#144123=CARTESIAN_POINT ( 'NONE',  ( 0.000000000000000000, 3.447199233515649386, 12.00000000000000178 ) ) ;
#144125=CIRCLE ( 'NONE', #157857, 11.99999999999999112 ) ;
#144177=CARTESIAN_POINT ( 'NONE',  ( -0.007565906569761434060, -9.598697202504085979, 9.591786056756831158 ) ) ;
#144179=ORIENTED_EDGE ( 'NONE', *, *, #132056, .F. ) ;
#144181=( BOUNDED_SURFACE ( )  B_SPLINE_SURFACE ( 3, 2, ( 
 ( #201646, #50102, #67375 ),
 ( #238, #168116, #68454 ),
 ( #19716, #99918, #133517 ),
 ( #116223, #98858, #120509 ),
 ( #182214, #53294, #103117 ),
 ( #117290, #165979, #100964 ),
 ( #149735, #85795, #151875 ),
 ( #164909, #198458, #3449 ) ),
 .UNSPECIFIED., .F., .F., .F. ) 
 B_SPLINE_SURFACE_WITH_KNOTS ( ( 4, 2, 2, 4 ),
 ( 3, 3 ),
 ( 0.000000000000000000, 0.0002575597274893386048, 0.0005151194549786772096, 0.001030238909957354419 ),
 ( 0.000000000000000000, 1.000000000000000000 ),
 .UNSPECIFIED. ) 
 GEOMETRIC_REPRESENTATION_ITEM ( )  RATIONAL_B_SPLINE_SURFACE ( (
 ( 1.000000000000000000, 0.9238795325112795220, 1.000000000000000000),
 ( 1.000000000000000000, 0.9228594682462778476, 1.000000000000000000),
 ( 1.000000000000000000, 0.9150875845228949590, 1.000000000000000000),
 ( 1.000000000000000000, 0.8905471774190931722, 1.000000000000000000),
 ( 1.000000000000000000, 0.8740340839247475735, 1.000000000000000000),
 ( 1.000000000000000000, 0.8160099319848322930, 1.000000000000000000),
 ( 1.000000000000000000, 0.7673743911477570734, 1.000000000000000000),
 ( 1.000000000000000000, 0.7100530722070661493, 1.000000000000000000) ) ) 
 REPRESENTATION_ITEM ( '' )  SURFACE ( )  );
#144182=ADVANCED_FACE ( 'NONE', ( #88840, #202540 ), #36856, .F. ) ;
#144191=CARTESIAN_POINT ( 'NONE',  ( -10.98974895236974092, -7.729832900979438648, 0.4787367839866840669 ) ) ;
#144196=DIRECTION ( 'NONE',  ( 0.000000000000000000, -1.000000000000000000, 0.000000000000000000 ) ) ;
#144216=CONICAL_SURFACE ( 'NONE', #168282, 10.99999999999998934, 0.7853981633974533860 ) ;
#144222=DIRECTION ( 'NONE',  ( 0.000000000000000000, 1.000000000000000000, 0.000000000000000000 ) ) ;
#144243=COLOUR_RGB ( '', 0.08235294, 0.09019608, 0.10196078) ;
#144251=ORIENTED_EDGE ( 'NONE', *, *, #138683, .F. ) ;
#144254=CARTESIAN_POINT ( 'NONE',  ( -7.681496476274705110, -5.295524846228442328, -7.873959529867720519 ) ) ;
#144275=CARTESIAN_POINT ( 'NONE',  ( 6.772456105771886392, -7.184999792969689381, 6.662120174140257589 ) ) ;
#144287=CARTESIAN_POINT ( 'NONE',  ( 6.444907381559374926, -8.233136965322506384, 6.980013479859862535 ) ) ;
#144299=VERTEX_POINT ( 'NONE', #6480 ) ;
#144319=VERTEX_POINT ( 'NONE', #85616 ) ;
#144331=VERTEX_POINT ( 'NONE', #56326 ) ;
#144369=CARTESIAN_POINT ( 'NONE',  ( 6.580818069394648973, -6.606405293530493772, 7.011678565220734960 ) ) ;
#144402=CARTESIAN_POINT ( 'NONE',  ( 7.834948825496932834, -6.134628647623485698, 7.720982897393586342 ) ) ;
#144404=MECHANICAL_DESIGN_GEOMETRIC_PRESENTATION_REPRESENTATION('',(#50797),#113192);
#144474=CARTESIAN_POINT ( 'NONE',  ( 0.07933194151889190471, -9.902237888914267927, 9.499668754386327407 ) ) ;
#144511=CARTESIAN_POINT ( 'NONE',  ( -7.501945787865621718, -5.223163706540480788, -8.013579835756324599 ) ) ;
#144566=ORIENTED_EDGE ( 'NONE', *, *, #199147, .T. ) ;
#144580=AXIS2_PLACEMENT_3D ( 'NONE', #131027, #83257, #32395 ) ;
#144582=CARTESIAN_POINT ( 'NONE',  ( -7.712474369503357075, -6.289226506789209914, -7.712474369503310889 ) ) ;
#144621=DIRECTION ( 'NONE',  ( 0.000000000000000000, 0.000000000000000000, -1.000000000000000000 ) ) ;
#144661=APPLICATION_CONTEXT ( 'automotive_design' ) ;
#144665=CARTESIAN_POINT ( 'NONE',  ( 10.18278199833527964, 3.974415841077570732, -5.432519183637642080 ) ) ;
#144680=AXIS2_PLACEMENT_3D ( 'NONE', #120537, #152956, #104217 ) ;
#144696=AXIS2_PLACEMENT_3D ( 'NONE', #93206, #11915, #92140 ) ;
#144714=EDGE_LOOP ( 'NONE', ( #164797, #70159, #46191, #86335 ) ) ;
#144766=DIRECTION ( 'NONE',  ( -0.000000000000000000, -1.000000000000000000, -0.000000000000000000 ) ) ;
#144770=CARTESIAN_POINT ( 'NONE',  ( -7.755938900619411491, -5.581885079358431589, 7.800371912476625091 ) ) ;
#144775=DIRECTION ( 'NONE',  ( 0.000000000000000000, 1.000000000000000000, 0.000000000000000000 ) ) ;
#144778=( BOUNDED_SURFACE ( )  B_SPLINE_SURFACE ( 3, 2, ( 
 ( #212798, #49261, #196570 ),
 ( #184562, #181376, #149959 ),
 ( #33000, #99077, #2599 ),
 ( #165130, #455, #36183 ),
 ( #64436, #34056, #1528 ),
 ( #67592, #66523, #100129 ),
 ( #137976, #89234, #41555 ),
 ( #202937, #140127, #169395 ) ),
 .UNSPECIFIED., .F., .F., .F. ) 
 B_SPLINE_SURFACE_WITH_KNOTS ( ( 4, 2, 2, 4 ),
 ( 3, 3 ),
 ( 0.000000000000000000, 0.0002475938981900030044, 0.0004951877963800060088, 0.0009903755927600120176 ),
 ( 0.000000000000000000, 1.000000000000000000 ),
 .UNSPECIFIED. ) 
 GEOMETRIC_REPRESENTATION_ITEM ( )  RATIONAL_B_SPLINE_SURFACE ( (
 ( 1.000000000000000000, 0.9238795325112900692, 1.000000000000000000),
 ( 1.000000000000000000, 0.9248499699755210468, 1.000000000000000000),
 ( 1.000000000000000000, 0.9171047238581204741, 1.000000000000000000),
 ( 1.000000000000000000, 0.8907236462371719288, 1.000000000000000000),
 ( 1.000000000000000000, 0.8725411758595089662, 1.000000000000000000),
 ( 1.000000000000000000, 0.8105159241142131377, 1.000000000000000000),
 ( 1.000000000000000000, 0.7599483315141056794, 1.000000000000000000),
 ( 1.000000000000000000, 0.7045118851637689472, 1.000000000000000000) ) ) 
 REPRESENTATION_ITEM ( '' )  SURFACE ( )  );
#144787=EDGE_LOOP ( 'NONE', ( #133532, #46022 ) ) ;
#144804=CARTESIAN_POINT ( 'NONE',  ( -9.609441814500819135, -6.583711573987011789, 0.3689019803512949558 ) ) ;
#144836=VERTEX_POINT ( 'NONE', #113910 ) ;
#144856=CARTESIAN_POINT ( 'NONE',  ( 8.081892667527538876, -5.200000000000006395, -7.462104991928523390 ) ) ;
#144861=VERTEX_POINT ( 'NONE', #176702 ) ;
#144874=CARTESIAN_POINT ( 'NONE',  ( 7.451274665340240411, -7.616254850791388975, -6.794158526849247259 ) ) ;
#144917=CARTESIAN_POINT ( 'NONE',  ( -0.03889815725003768071, -8.115420858948564131, 10.94377971103912195 ) ) ;
#144933=ORIENTED_EDGE ( 'NONE', *, *, #29125, .T. ) ;
#144934=ADVANCED_FACE ( 'NONE', ( #195084 ), #68144, .T. ) ;
#144960=CARTESIAN_POINT ( 'NONE',  ( 7.720982910012531342, -6.306565840633542308, -7.834948813061516582 ) ) ;
#145013=CIRCLE ( 'NONE', #55151, 11.89429233241351902 ) ;
#145104=CARTESIAN_POINT ( 'NONE',  ( -0.03436587256745584490, -7.792803924024958029, -9.554207839743707353 ) ) ;
#145180=CARTESIAN_POINT ( 'NONE',  ( -6.773846765307993678, -7.473374494058229622, -6.773846765307958151 ) ) ;
#145198=ADVANCED_FACE ( 'NONE', ( #184143 ), #102908, .T. ) ;
#145228=ORIENTED_EDGE ( 'NONE', *, *, #146528, .F. ) ;
#145242=VERTEX_POINT ( 'NONE', #165782 ) ;
#145246=CARTESIAN_POINT ( 'NONE',  ( -10.95700306400769897, -7.901429653175727097, 0.3289054322349619919 ) ) ;
#145249=( GEOMETRIC_REPRESENTATION_CONTEXT ( 3 ) GLOBAL_UNCERTAINTY_ASSIGNED_CONTEXT ( ( #33457 ) ) GLOBAL_UNIT_ASSIGNED_CONTEXT ( ( #151033, #52451, #1532 ) ) REPRESENTATION_CONTEXT ( 'NONE', 'WORKASPACE' ) );
#145267=EDGE_CURVE ( 'NONE', #115982, #157333, #167909, .T. ) ;
#145289=EDGE_CURVE ( 'NONE', #99453, #159480, #151217, .T. ) ;
#145304=EDGE_LOOP ( 'NONE', ( #55275, #195175, #6259, #177939, #44043 ) ) ;
#145311=CARTESIAN_POINT ( 'NONE',  ( -7.730132016634532199, -5.756136661604536187, -7.730132016634490455 ) ) ;
#145316=CARTESIAN_POINT ( 'NONE',  ( -11.18654035131441127, 1.000000000000000888, 4.041720556560751021 ) ) ;
#145346=DIRECTION ( 'NONE',  ( 0.000000000000000000, 0.000000000000000000, 1.000000000000000000 ) ) ;
#145373=UNCERTAINTY_MEASURE_WITH_UNIT (LENGTH_MEASURE( 1.000000000000000082E-05 ), #180815, 'distance_accuracy_value', 'NONE');
#145375=CARTESIAN_POINT ( 'NONE',  ( 0.003376046620571365731, -7.161464053357560644, 9.586610838029431036 ) ) ;
#145383=CARTESIAN_POINT ( 'NONE',  ( -7.055228938194283650, -8.176568542494891290, 6.396834479292372144 ) ) ;
#145390=ORIENTED_EDGE ( 'NONE', *, *, #91149, .T. ) ;
#145439=CARTESIAN_POINT ( 'NONE',  ( 6.445605026751811018, -8.233137084989715859, 6.979380938965673131 ) ) ;
#145486=B_SPLINE_CURVE_WITH_KNOTS ( 'NONE', 3,
 ( #102076, #83679, #118387, #134610, #184376, #133547, #20797, #35995 ),
 .UNSPECIFIED., .F., .F.,
 ( 4, 2, 2, 4 ),
 ( 0.000000000000000000, 0.0002034531274099183142, 0.0004069062548198371706, 0.0008138125096396707633 ),
 .UNSPECIFIED. ) ;
#145498=DIRECTION ( 'NONE',  ( 1.000000000000000000, -0.000000000000000000, 1.224646799147353207E-16 ) ) ;
#145505=CARTESIAN_POINT ( 'NONE',  ( 6.855650617048432593, -7.357813805523310435, -6.855650617048458351 ) ) ;
#145604=CARTESIAN_POINT ( 'NONE',  ( 10.45358220256315285, 1.000000000000000888, -5.892590188894412329 ) ) ;
#145667=COLOUR_RGB ( '', 0.40784314, 0.44705882, 0.49803922) ;
#145703=B_SPLINE_CURVE_WITH_KNOTS ( 'NONE', 3,
 ( #180634, #179580, #96214, #182758 ),
 .UNSPECIFIED., .F., .F.,
 ( 4, 4 ),
 ( 0.000000000000000000, 0.0004065497138311910700 ),
 .UNSPECIFIED. ) ;
#145736=DIRECTION ( 'NONE',  ( 0.000000000000000000, -1.000000000000000000, 0.000000000000000000 ) ) ;
#145758=EDGE_LOOP ( 'NONE', ( #10911, #89041 ) ) ;
#145763=CARTESIAN_POINT ( 'NONE',  ( 0.3870735955438693310, 1.000000000000000888, -11.88799243440807274 ) ) ;
#145781=CARTESIAN_POINT ( 'NONE',  ( -10.99943592164172834, -9.999999999999994671, 0.1113975120798846308 ) ) ;
#145783=LINE ( 'NONE', #211786, #40766 ) ;
#145791=CARTESIAN_POINT ( 'NONE',  ( -0.2619794211619215218, -6.848541063415908070, -10.99716886186657661 ) ) ;
#145810=CARTESIAN_POINT ( 'NONE',  ( 0.000000000000000000, -5.166862915010159263, 0.000000000000000000 ) ) ;
#145846=ORIENTED_EDGE ( 'NONE', *, *, #118406, .T. ) ;
#145863=CARTESIAN_POINT ( 'NONE',  ( -7.317172109022185289, -6.705807696133232021, -7.317172109022152426 ) ) ;
#145903=CARTESIAN_POINT ( 'NONE',  ( 11.10517813317444791, 1.720726420432414194, -4.015189785735423733 ) ) ;
#145941=SURFACE_STYLE_USAGE ( .BOTH. , #80907 ) ;
#145961=FACE_OUTER_BOUND ( 'NONE', #144714, .T. ) ;
#146031=PRESENTATION_STYLE_ASSIGNMENT (( #79924 ) ) ;
#146073=SURFACE_STYLE_USAGE ( .BOTH. , #62648 ) ;
#146105=VERTEX_POINT ( 'NONE', #200135 ) ;
#146147=ORIENTED_EDGE ( 'NONE', *, *, #106908, .F. ) ;
#146160=CARTESIAN_POINT ( 'NONE',  ( -0.3866913795912775842, 3.974415841077572509, 11.53480748357604035 ) ) ;
#146171=VERTEX_POINT ( 'NONE', #70126 ) ;
#146232=CARTESIAN_POINT ( 'NONE',  ( -7.465774003072983334, -6.268611901546733201, -7.465774003072939813 ) ) ;
#146284=EDGE_LOOP ( 'NONE', ( #75634, #3864 ) ) ;
#146286=CARTESIAN_POINT ( 'NONE',  ( -7.834948825496940827, -6.134628647623485698, -7.720982897393570354 ) ) ;
#146287=CARTESIAN_POINT ( 'NONE',  ( 7.679448064523580975, -6.453073674884648447, 7.727353211424090595 ) ) ;
#146288=CARTESIAN_POINT ( 'NONE',  ( -0.1738264060025679902, -9.190401220100135049, 9.624818503329224839 ) ) ;
#146321=ORIENTED_EDGE ( 'NONE', *, *, #114330, .T. ) ;
#146338=CARTESIAN_POINT ( 'NONE',  ( -9.499668754385632852, -7.246166700194470067, -0.07933194154487524519 ) ) ;
#146391=CARTESIAN_POINT ( 'NONE',  ( 6.773376349083136461, -7.473374494058229622, 6.661184041420955104 ) ) ;
#146417=DIRECTION ( 'NONE',  ( 0.000000000000000000, 0.000000000000000000, 1.000000000000000000 ) ) ;
#146418=ORIENTED_EDGE ( 'NONE', *, *, #192938, .T. ) ;
#146421=CARTESIAN_POINT ( 'NONE',  ( 0.001123102408843089329, -7.189630408304394926, 9.584291988782279503 ) ) ;
#146422=CIRCLE ( 'NONE', #181016, 0.07999999999999979350 ) ;
#146428=CARTESIAN_POINT ( 'NONE',  ( -6.663994888585887288, -7.154544010627095219, 6.770610912236890044 ) ) ;
#146430=ORIENTED_EDGE ( 'NONE', *, *, #62981, .T. ) ;
#146483=CARTESIAN_POINT ( 'NONE',  ( -0.04582610853913851590, -10.00039265882532824, -11.00004154231846520 ) ) ;
#146494=CIRCLE ( 'NONE', #53060, 0.07999999999999993228 ) ;
#146497=CIRCLE ( 'NONE', #80758, 0.08000000000000020983 ) ;
#146517=SURFACE_STYLE_FILL_AREA ( #195240 ) ;
#146528=EDGE_CURVE ( 'NONE', #93013, #147554, #26088, .T. ) ;
#146531=CARTESIAN_POINT ( 'NONE',  ( -0.08058606167704472634, -5.741816521215563185, 10.99970480906934078 ) ) ;
#146548=FACE_OUTER_BOUND ( 'NONE', #74362, .T. ) ;
#146549=DIRECTION ( 'NONE',  ( 0.000000000000000000, 0.000000000000000000, 1.000000000000000000 ) ) ;
#146554=CARTESIAN_POINT ( 'NONE',  ( -9.579665964948885559, 7.849261790823902629, -0.07999999999998980149 ) ) ;
#146565=DIRECTION ( 'NONE',  ( 0.000000000000000000, 0.000000000000000000, 1.000000000000000000 ) ) ;
#146576=AXIS2_PLACEMENT_3D ( 'NONE', #146554, #213618, #129302 ) ;
#146589=CARTESIAN_POINT ( 'NONE',  ( -9.484513307599961252, -6.630981389236807466, 0.1588444833727626904 ) ) ;
#146616=B_SPLINE_CURVE_WITH_KNOTS ( 'NONE', 3,
 ( #121583, #136695, #17566, #149739, #135627, #119429, #1316, #67378, #133519, #86865, #199525, #51169, #202721, #152929, #186487, #168118 ),
 .UNSPECIFIED., .F., .F.,
 ( 4, 3, 3, 3, 3, 4 ),
 ( 0.000000000000000000, 4.416163517950592750E-06, 1.117787330550273205E-05, 1.792356377820730995E-05, 2.465171878522349184E-05, 3.136847552909858286E-05 ),
 .UNSPECIFIED. ) ;
#146620=ORIENTED_EDGE ( 'NONE', *, *, #134985, .F. ) ;
#146626=DIRECTION ( 'NONE',  ( 0.000000000000000000, 1.000000000000000000, 0.000000000000000000 ) ) ;
#146660=DIRECTION ( 'NONE',  ( -0.000000000000000000, 1.000000000000000000, -0.000000000000000000 ) ) ;
#146736=EDGE_LOOP ( 'NONE', ( #83566, #47981, #153580, #55960, #35921 ) ) ;
#146787=CARTESIAN_POINT ( 'NONE',  ( 10.33323920393387674, 4.021557182957052667, -5.965898435992177617 ) ) ;
#146810=CLOSED_SHELL ( 'NONE', ( #158998, #121837, #56893, #5413, #97096, #59390, #74522, #17633, #42237, #195134, #65822, #36430, #87466, #79941, #165584, #37195, #86509, #149431, #173956, #201706, #196298, #48143, #25207, #174913, #27242, #85507, #43465, #178025, #159434, #37096, #94400, #117578, #144182, #119978, #56751, #81437, #160339, #202122, #179324, #197936, #22111, #19570, #189681, #33195, #100399, #110329, #159239, #86557, #66162, #182098, #156957, #75064, #210702, #128008, #203108, #57138, #90115, #43581, #206144, #56506, #108668, #142814, #194303, #125431, #194681, #203429, #172604, #196809, #86101, #15528, #74846, #44250, #158480, #122337, #62018, #90432, #123144, #54222, #71794, #76442, #144934, #76659, #74075, #84066, #20749, #40352, #52077, #196198, #192908, #184803, #210893, #90686, #180697, #51670, #160866, #137121, #127673, #16500, #208816, #150135, #178601, #200866, #15402, #113616, #134474, #208955, #58775, #202344, #151998, #18732, #8764, #152763, #80978, #102849, #82199, #92642, #108806, #135685, #153018, #11779, #127235, #206650, #135663, #109787, #155903, #86819, #162261, #203635, #38249, #143567, #3210, #23203, #57915, #199601, #191707, #141003, #155116, #166198, #145198, #40762, #35450, #138164, #121014, #198057, #1659, #180030, #115127, #96258, #99603, #108118, #106561, #105238, #191153, #101058, #39511, #163169, #151627, #78029, #64949, #96395, #117192, #100389, #25256, #200993, #16231, #133529, #66977, #110808, #174907, #115639, #26585, #59158, #58379, #181907, #69647, #198572, #97080, #57415, #129065, #147458, #109652, #165521, #30087, #104698, #211495, #203821, #59775, #195939, #110287, #21707, #85334, #105000, #120104, #133198, #11, #167897, #1172, #176145, #50966, #199778, #1267, #8363, #96339, #60535, #115223, #134212, #88291, #201696, #30024, #49813, #134495, #192810, #62527, #27069, #48204, #77243, #97602, #39071, #97204, #92629, #4429, #105685, #5782, #195534, #93703, #172492, #80396, #28318, #178501, #76793, #8950, #80971, #91529, #200496, #52970, #192497, #110989 ) ) ;
#146814=CARTESIAN_POINT ( 'NONE',  ( 9.612263720970512182, -6.681311647492914396, -0.1963700886235927867 ) ) ;
#146823=CARTESIAN_POINT ( 'NONE',  ( 10.91962425643199985, -9.919999999999998153, -0.09058751758333170867 ) ) ;
#146827=CARTESIAN_POINT ( 'NONE',  ( -2.093037498677872144, 1.000000000000000888, 11.70868840297834446 ) ) ;
#146844=CARTESIAN_POINT ( 'NONE',  ( -0.4356160240586524068, -9.063431457505059186, 9.626717610576628559 ) ) ;
#146898=VERTEX_POINT ( 'NONE', #87784 ) ;
#146958=CARTESIAN_POINT ( 'NONE',  ( 10.85277107007934205, 3.956598013261175772, -3.932872935640606915 ) ) ;
#146998=CARTESIAN_POINT ( 'NONE',  ( 0.000000000000000000, -9.999999999999994671, 0.000000000000000000 ) ) ;
#147025=EDGE_CURVE ( 'NONE', #67059, #204013, #38908, .T. ) ;
#147046=EDGE_CURVE ( 'NONE', #71330, #19391, #141048, .T. ) ;
#147056=VECTOR ( 'NONE', #91982, 1000.000000000000000 ) ;
#147110=ORIENTED_EDGE ( 'NONE', *, *, #9580, .F. ) ;
#147130=CARTESIAN_POINT ( 'NONE',  ( -10.39230484541327826, 3.447199233515649386, -5.999999999999975131 ) ) ;
#147195=CARTESIAN_POINT ( 'NONE',  ( -9.579764304849261336, -9.999999999999998224, 0.06720017513373673090 ) ) ;
#147217=FACE_OUTER_BOUND ( 'NONE', #85141, .T. ) ;
#147231=CARTESIAN_POINT ( 'NONE',  ( -3.428579710538708225E-15, -7.630846356335694303, 9.566809970446875866 ) ) ;
#147294=EDGE_LOOP ( 'NONE', ( #82832, #64860, #138944 ) ) ;
#147300=CARTESIAN_POINT ( 'NONE',  ( 6.717278222822382183, -7.246166700180828535, -6.830415307812249814 ) ) ;
#147332=CARTESIAN_POINT ( 'NONE',  ( 0.05647967004077469183, -9.990726209582318162, 9.579565160031989990 ) ) ;
#147333=CARTESIAN_POINT ( 'NONE',  ( -6.937452841262722103, -7.242250812743806776, -6.937452841262681247 ) ) ;
#147347=EDGE_LOOP ( 'NONE', ( #115577, #149753, #135128, #89001 ) ) ;
#147352=( GEOMETRIC_REPRESENTATION_CONTEXT ( 3 ) GLOBAL_UNCERTAINTY_ASSIGNED_CONTEXT ( ( #73620 ) ) GLOBAL_UNIT_ASSIGNED_CONTEXT ( ( #75431, #106921, #172945 ) ) REPRESENTATION_CONTEXT ( 'NONE', 'WORKASPACE' ) );
#147370=CARTESIAN_POINT ( 'NONE',  ( -0.3313999689851416797, -9.006862915010142245, 9.494725171580526535 ) ) ;
#147403=ORIENTED_EDGE ( 'NONE', *, *, #201684, .F. ) ;
#147438=VERTEX_POINT ( 'NONE', #117960 ) ;
#147439=CARTESIAN_POINT ( 'NONE',  ( 6.717748655460326290, -7.473374494057241080, 6.717748655458911422 ) ) ;
#147454=AXIS2_PLACEMENT_3D ( 'NONE', #74131, #73038, #188935 ) ;
#147458=ADVANCED_FACE ( 'NONE', ( #17171 ), #164948, .T. ) ;
#147467=LINE ( 'NONE', #196210, #157384 ) ;
#147486=ORIENTED_EDGE ( 'NONE', *, *, #177138, .F. ) ;
#147530=CARTESIAN_POINT ( 'NONE',  ( 10.86205067566995552, -6.804704122739854810, -0.3107038660269284547 ) ) ;
#147533=CARTESIAN_POINT ( 'NONE',  ( -1.786647479811285890E-05, -9.954793286625749360, -11.00029511060593634 ) ) ;
#147546=CARTESIAN_POINT ( 'NONE',  ( 7.667935170093241659, -6.766388843766955929, 7.887197531381555216 ) ) ;
#147551=CARTESIAN_POINT ( 'NONE',  ( 0.03889815725003424596, -8.115420858948564131, -10.94377971103912195 ) ) ;
#147554=VERTEX_POINT ( 'NONE', #48643 ) ;
#147556=CARTESIAN_POINT ( 'NONE',  ( 9.886825906824942223, 3.934660213246443661, 6.000867881395502756 ) ) ;
#147570=CARTESIAN_POINT ( 'NONE',  ( 0.3866937364864087567, 3.956598013261175772, -11.53692321988872926 ) ) ;
#147576=CARTESIAN_POINT ( 'NONE',  ( 0.2726351642629436522, -5.197079954928608636, 10.99683038201373719 ) ) ;
#147594=ORIENTED_EDGE ( 'NONE', *, *, #95387, .F. ) ;
#147606=AXIS2_PLACEMENT_3D ( 'NONE', #93122, #205768, #189525 ) ;
#147632=CARTESIAN_POINT ( 'NONE',  ( 0.003376046620557637129, -7.161464053357565973, 9.586610838029432813 ) ) ;
#147642=CIRCLE ( 'NONE', #64603, 0.08000000000000020983 ) ;
#147708=EDGE_CURVE ( 'NONE', #147554, #73672, #61051, .T. ) ;
#147788=CYLINDRICAL_SURFACE ( 'NONE', #39077, 11.99999999999999112 ) ;
#147798=CARTESIAN_POINT ( 'NONE',  ( 6.661184041420940005, 7.849261790823902629, -6.773376349083132908 ) ) ;
#147862=CARTESIAN_POINT ( 'NONE',  ( 9.605391220871890567, -6.900199406649618616, -0.04765083308771667775 ) ) ;
#147883=CARTESIAN_POINT ( 'NONE',  ( 0.4655726814510594003, -8.186910006429393150, 9.501690549794789220 ) ) ;
#147905=UNCERTAINTY_MEASURE_WITH_UNIT (LENGTH_MEASURE( 1.000000000000000082E-05 ), #51279, 'distance_accuracy_value', 'NONE');
#147927=FACE_OUTER_BOUND ( 'NONE', #80895, .T. ) ;
#147931=CARTESIAN_POINT ( 'NONE',  ( 10.91970695577495931, -5.907420853759283830, 1.951563910473907981E-15 ) ) ;
#147964=CARTESIAN_POINT ( 'NONE',  ( -9.611339018008548507, -6.606549254265005722, 0.3046331935817704895 ) ) ;
#148043=CARTESIAN_POINT ( 'NONE',  ( 6.773846765307987461, -7.473374494058229622, 6.773846765307971474 ) ) ;
#148047=CARTESIAN_POINT ( 'NONE',  ( -10.87634538855766841, 3.956598013261175772, 3.867819554622464739 ) ) ;
#148049=CARTESIAN_POINT ( 'NONE',  ( -0.1899713450103351353, -8.048696291100961631, -9.532262708098288684 ) ) ;
#148060=DIRECTION ( 'NONE',  ( 0.000000000000000000, -1.000000000000000000, 0.000000000000000000 ) ) ;
#148063=CIRCLE ( 'NONE', #206785, 10.91999999999999105 ) ;
#148102=AXIS2_PLACEMENT_3D ( 'NONE', #78056, #62866, #173455 ) ;
#148118=CARTESIAN_POINT ( 'NONE',  ( 10.96785329849812562, -5.223431457505089526, -0.4373225248172959434 ) ) ;
#148144=CARTESIAN_POINT ( 'NONE',  ( 10.99998664267163484, -6.472053282365753724, 0.02741317976724608543 ) ) ;
#148151=CARTESIAN_POINT ( 'NONE',  ( -6.772456105771887280, -7.184999792969690269, -6.662120174140245155 ) ) ;
#148159=CARTESIAN_POINT ( 'NONE',  ( 6.773376349083136461, -7.246166700180801001, 6.661184041420955104 ) ) ;
#148164=CARTESIAN_POINT ( 'NONE',  ( 0.000000000000000000, -7.154544010627095219, 0.000000000000000000 ) ) ;
#148187=CARTESIAN_POINT ( 'NONE',  ( -7.446209719563359641, -5.223431457505076203, -8.064677165291183059 ) ) ;
#148191=PRESENTATION_STYLE_ASSIGNMENT (( #146073 ) ) ;
#148192=CARTESIAN_POINT ( 'NONE',  ( -10.39025099420816467, 3.467171072964058354, -5.998814208453826069 ) ) ;
#148250=UNCERTAINTY_MEASURE_WITH_UNIT (LENGTH_MEASURE( 1.000000000000000082E-05 ), #121366, 'distance_accuracy_value', 'NONE');
#148266=ORIENTED_EDGE ( 'NONE', *, *, #15354, .T. ) ;
#148277=DIRECTION ( 'NONE',  ( 0.000000000000000000, 0.000000000000000000, -1.000000000000000000 ) ) ;
#148379=EDGE_CURVE ( 'NONE', #160219, #14247, #128656, .T. ) ;
#148411=FACE_OUTER_BOUND ( 'NONE', #129071, .T. ) ;
#148428=DIRECTION ( 'NONE',  ( -1.000000000000000000, 0.000000000000000000, 0.000000000000000000 ) ) ;
#148467=CARTESIAN_POINT ( 'NONE',  ( 0.000000000000000000, 4.006659545634088992, 0.000000000000000000 ) ) ;
#148477=CARTESIAN_POINT ( 'NONE',  ( -11.28709712336964444, 1.000000000000000888, 3.871943585349969741 ) ) ;
#148501=CARTESIAN_POINT ( 'NONE',  ( -9.579417154662856149, -9.998067499250632650, 0.08973735058633736106 ) ) ;
#148502=CARTESIAN_POINT ( 'NONE',  ( 8.044078759455164374, -6.893137084989842123, -7.385065802799731571 ) ) ;
#148514=EDGE_CURVE ( 'NONE', #14615, #148901, #71382, .T. ) ;
#148526=DIRECTION ( 'NONE',  ( 0.000000000000000000, 1.000000000000000000, 0.000000000000000000 ) ) ;
#148546=ORIENTED_EDGE ( 'NONE', *, *, #85823, .F. ) ;
#148553=ORIENTED_EDGE ( 'NONE', *, *, #189032, .F. ) ;
#148587=VERTEX_POINT ( 'NONE', #17978 ) ;
#148592=CARTESIAN_POINT ( 'NONE',  ( 9.499606442108960991, -9.746166700193986898, -0.08647222121512777859 ) ) ;
#148605=CARTESIAN_POINT ( 'NONE',  ( 6.726765609221548203, -8.198316280115703236, -6.726765609221573960 ) ) ;
#148623=B_SPLINE_CURVE_WITH_KNOTS ( 'NONE', 3,
 ( #179828, #31448, #64982, #97526, #10901, #163583, #143104, #15165, #81253, #60732, #147332, #213361, #131137, #197126, #48764, #159303 ),
 .UNSPECIFIED., .F., .F.,
 ( 4, 3, 3, 3, 3, 4 ),
 ( 0.000000000000000000, 3.357617230303741650E-05, 6.715207102180727422E-05, 0.0001007279560762672547, 0.0001343044553218119316, 0.0001562161319167451969 ),
 .UNSPECIFIED. ) ;
#148632=DIRECTION ( 'NONE',  ( 0.000000000000000000, -1.000000000000000000, 0.000000000000000000 ) ) ;
#148662=CARTESIAN_POINT ( 'NONE',  ( 6.777912011469600095, -7.189630408300057951, -6.776323704810597981 ) ) ;
#148698=CARTESIAN_POINT ( 'NONE',  ( 0.07933194154487524519, -9.900000000000005684, 9.499668754385634628 ) ) ;
#148777=CARTESIAN_POINT ( 'NONE',  ( 0.000000000000000000, -8.407420853759283830, 10.91970695577495931 ) ) ;
#148839=CARTESIAN_POINT ( 'NONE',  ( -0.4373225248172993851, -5.223431457505089526, -10.96785329849811497 ) ) ;
#148852=EDGE_CURVE ( 'NONE', #71330, #201806, #170721, .T. ) ;
#148871=FACE_OUTER_BOUND ( 'NONE', #150582, .T. ) ;
#148901=VERTEX_POINT ( 'NONE', #91864 ) ;
#148908=VECTOR ( 'NONE', #105881, 1000.000000000000000 ) ;
#148930=VERTEX_POINT ( 'NONE', #61463 ) ;
#148933=CARTESIAN_POINT ( 'NONE',  ( -2.331034670843834533E-15, -7.287292266289724374, 9.765991025965632844 ) ) ;
#148949=CARTESIAN_POINT ( 'NONE',  ( 0.3852658704378412735, -6.836271227032193032, 10.85717823004580751 ) ) ;
#148954=CARTESIAN_POINT ( 'NONE',  ( 7.777967379493318845, -6.134628647623484810, 7.744830294503448620 ) ) ;
#148998=CARTESIAN_POINT ( 'NONE',  ( -4.900932632813380184E-15, -5.758458176070767820, -10.93186801223269811 ) ) ;
#149009=CYLINDRICAL_SURFACE ( 'NONE', #112881, 10.99999999999999112 ) ;
#149055=CARTESIAN_POINT ( 'NONE',  ( -1.138412281109779656E-15, -9.181223591647238891, 10.14523337821910864 ) ) ;
#149095=DIRECTION ( 'NONE',  ( 0.000000000000000000, 0.000000000000000000, -1.000000000000000000 ) ) ;
#149119=VERTEX_POINT ( 'NONE', #28971 ) ;
#149127=CARTESIAN_POINT ( 'NONE',  ( -7.721398836998370818, -6.134628647623487474, 7.721398836998398352 ) ) ;
#149131=CARTESIAN_POINT ( 'NONE',  ( -7.721398836998405457, -6.134628647623499909, -7.721398836998363713 ) ) ;
#149155=LINE ( 'NONE', #137199, #52257 ) ;
#149198=AXIS2_PLACEMENT_3D ( 'NONE', #13051, #196095, #178786 ) ;
#149231=B_SPLINE_CURVE_WITH_KNOTS ( 'NONE', 3,
 ( #158120, #193788, #125686, #142959, #177560, #62721, #27019 ),
 .UNSPECIFIED., .F., .F.,
 ( 4, 3, 4 ),
 ( 8.673617379884018139E-19, 0.0008000000000005095049, 0.002977368225425563401 ),
 .UNSPECIFIED. ) ;
#149300=ORIENTED_EDGE ( 'NONE', *, *, #183636, .F. ) ;
#149339=FACE_OUTER_BOUND ( 'NONE', #29385, .T. ) ;
#149394=CARTESIAN_POINT ( 'NONE',  ( -2.494940289813118994, 3.447199233515649386, 11.73777120880565583 ) ) ;
#149419=CARTESIAN_POINT ( 'NONE',  ( 0.000000000000000000, 3.079999999999999183, -6.329999999999995630 ) ) ;
#149431=ADVANCED_FACE ( 'NONE', ( #24665 ), #95870, .T. ) ;
#149447=EDGE_LOOP ( 'NONE', ( #166843, #105972, #76761, #156661 ) ) ;
#149450=DIRECTION ( 'NONE',  ( -0.000000000000000000, -1.000000000000000000, -0.000000000000000000 ) ) ;
#149497=CARTESIAN_POINT ( 'NONE',  ( 9.858406733136186526E-16, 7.849261790823902629, -8.049999999999993605 ) ) ;
#149504=DIRECTION ( 'NONE',  ( 0.000000000000000000, 1.000000000000000000, 0.000000000000000000 ) ) ;
#149505=DIRECTION ( 'NONE',  ( 0.9510565162951521989, 0.000000000000000000, -0.3090169943749515591 ) ) ;
#149524=VERTEX_POINT ( 'NONE', #190365 ) ;
#149530=FACE_OUTER_BOUND ( 'NONE', #120038, .T. ) ;
#149552=CIRCLE ( 'NONE', #211847, 10.91999999999999105 ) ;
#149600=B_SPLINE_CURVE_WITH_KNOTS ( 'NONE', 3,
 ( #57552, #89000, #138813, #122645 ),
 .UNSPECIFIED., .F., .F.,
 ( 4, 4 ),
 ( 0.0005671806269306093424, 0.0008743016172331036749 ),
 .UNSPECIFIED. ) ;
#149616=DIRECTION ( 'NONE',  ( 0.000000000000000000, -1.000000000000000000, 0.000000000000000000 ) ) ;
#149632=CIRCLE ( 'NONE', #204951, 0.08000000000000020983 ) ;
#149649=EDGE_LOOP ( 'NONE', ( #113912, #114344, #54328, #105383 ) ) ;
#149655=CARTESIAN_POINT ( 'NONE',  ( 9.493819324367764878, -9.279866070759380747, -0.3645580569637754120 ) ) ;
#149658=B_SPLINE_CURVE_WITH_KNOTS ( 'NONE', 3,
 ( #180624, #85257, #80996, #164383, #66836, #130881, #148144, #67909, #184880, #35436 ),
 .UNSPECIFIED., .F., .F.,
 ( 4, 2, 2, 2, 4 ),
 ( 0.000000000000000000, 0.0002598598948551708457, 0.0005197197897103416914, 0.0007795796845655125372, 0.001039439579420683383 ),
 .UNSPECIFIED. ) ;
#149720=ORIENTED_EDGE ( 'NONE', *, *, #143030, .F. ) ;
#149723=EDGE_LOOP ( 'NONE', ( #3160, #34775, #156820, #76278 ) ) ;
#149727=CARTESIAN_POINT ( 'NONE',  ( 9.579603127937247109, 7.849261790823902629, -0.08720040834114990702 ) ) ;
#149735=CARTESIAN_POINT ( 'NONE',  ( -6.764644832400126262, -7.632775601084264672, -6.764644832402675334 ) ) ;
#149739=CARTESIAN_POINT ( 'NONE',  ( 9.499610831742323569, -9.904389604292740401, -0.08598863555141049442 ) ) ;
#149753=ORIENTED_EDGE ( 'NONE', *, *, #190504, .F. ) ;
#149794=CARTESIAN_POINT ( 'NONE',  ( -9.499640643549723151, -8.037485387949200089, 0.09382487309180524704 ) ) ;
#149833=CARTESIAN_POINT ( 'NONE',  ( 10.39230484541318589, 3.038454817776199857, -6.000000000000105693 ) ) ;
#149853=CARTESIAN_POINT ( 'NONE',  ( 0.4294077647110511320, -6.532648833121157850, 9.469892045836672878 ) ) ;
#149854=FILL_AREA_STYLE ('',( #118471 ) ) ;
#149866=SURFACE_SIDE_STYLE ('',( #134699 ) ) ;
#149874=DIRECTION ( 'NONE',  ( 0.000000000000000000, 1.000000000000000000, 0.000000000000000000 ) ) ;
#149951=CIRCLE ( 'NONE', #143031, 0.08000000000000020983 ) ;
#149959=CARTESIAN_POINT ( 'NONE',  ( -10.97093617010560429, -5.223179855899848789, 0.3663205537282924751 ) ) ;
#149988=EDGE_CURVE ( 'NONE', #74967, #184212, #160368, .T. ) ;
#150001=EDGE_LOOP ( 'NONE', ( #140413, #140175, #72793, #152833, #19833, #170749, #207888, #64527, #43963, #211633, #55952, #182858, #10974, #59213, #43457, #124903, #91388, #38710, #63429, #39986, #159383, #22883, #164633, #147486, #87906 ) ) ;
#150002=CARTESIAN_POINT ( 'NONE',  ( 9.481437597266046069, -6.708819892820501174, -0.4299312922663391379 ) ) ;
#150013=ORIENTED_EDGE ( 'NONE', *, *, #7856, .T. ) ;
#150016=FACE_OUTER_BOUND ( 'NONE', #14329, .T. ) ;
#150023=AXIS2_PLACEMENT_3D ( 'NONE', #173661, #25234, #58811 ) ;
#150029=CARTESIAN_POINT ( 'NONE',  ( -0.07933194154488912297, -7.246166700194011767, 9.499668754385634628 ) ) ;
#150066=CARTESIAN_POINT ( 'NONE',  ( -9.499606442108964544, -9.746166700193986898, 0.08647222121513538362 ) ) ;
#150135=ADVANCED_FACE ( 'NONE', ( #208982 ), #43332, .F. ) ;
#150146=AXIS2_PLACEMENT_3D ( 'NONE', #34242, #211923, #33184 ) ;
#150154=EDGE_CURVE ( 'NONE', #26009, #28024, #116618, .T. ) ;
#150171=UNCERTAINTY_MEASURE_WITH_UNIT (LENGTH_MEASURE( 1.000000000000000082E-05 ), #7069, 'distance_accuracy_value', 'NONE');
#150173=DIRECTION ( 'NONE',  ( 0.000000000000000000, 1.000000000000000000, 0.000000000000000000 ) ) ;
#150209=DIRECTION ( 'NONE',  ( 1.544526636936600361E-14, -1.000000000000000000, 1.522060196430166414E-14 ) ) ;
#150214=CARTESIAN_POINT ( 'NONE',  ( -7.886602582589937960, -6.765616048178459963, 7.668547801473422965 ) ) ;
#150283=ORIENTED_EDGE ( 'NONE', *, *, #80621, .T. ) ;
#150284=DIRECTION ( 'NONE',  ( 0.000000000000000000, 0.000000000000000000, 1.000000000000000000 ) ) ;
#150329=SURFACE_SIDE_STYLE ('',( #1896 ) ) ;
#150412=FILL_AREA_STYLE ('',( #84326 ) ) ;
#150419=VECTOR ( 'NONE', #172156, 1000.000000000000000 ) ;
#150530=ORIENTED_EDGE ( 'NONE', *, *, #97346, .F. ) ;
#150533=CARTESIAN_POINT ( 'NONE',  ( -0.09770433987277686583, -9.919999999999998153, -9.499497670693795470 ) ) ;
#150543=CARTESIAN_POINT ( 'NONE',  ( 0.07999999999998980149, -9.999999999999994671, -10.91970695577493977 ) ) ;
#150550=MECHANICAL_DESIGN_GEOMETRIC_PRESENTATION_REPRESENTATION('',(#12153),#188568);
#150582=EDGE_LOOP ( 'NONE', ( #17451, #15426, #174173, #144251 ) ) ;
#150588=CARTESIAN_POINT ( 'NONE',  ( -10.39230484541327826, 3.447199233515649386, -5.999999999999975131 ) ) ;
#150609=DIRECTION ( 'NONE',  ( 0.000000000000000000, 0.000000000000000000, 1.000000000000000000 ) ) ;
#150622=EDGE_LOOP ( 'NONE', ( #158688, #111960, #24373, #55674 ) ) ;
#150639=PRESENTATION_STYLE_ASSIGNMENT (( #151704 ) ) ;
#150679=CARTESIAN_POINT ( 'NONE',  ( 11.38999389752405023, 1.405705671057797534, -3.777644806142902656 ) ) ;
#150735=CARTESIAN_POINT ( 'NONE',  ( 9.498763045328258769, -9.581505939640273084, -0.1791256580993725867 ) ) ;
#150746=AXIS2_PLACEMENT_3D ( 'NONE', #204007, #172624, #55655 ) ;
#150748=CARTESIAN_POINT ( 'NONE',  ( -9.797921721691023933, 3.956598013261175772, -6.103348209225892163 ) ) ;
#150753=CARTESIAN_POINT ( 'NONE',  ( 0.2897211420239304558, -7.754973434576989177, -10.97056425546336023 ) ) ;
#150785=CARTESIAN_POINT ( 'NONE',  ( 10.98997987423604172, -6.893137084989842123, -0.4694063952341842594 ) ) ;
#150828=ORIENTED_EDGE ( 'NONE', *, *, #158729, .F. ) ;
#150834=CARTESIAN_POINT ( 'NONE',  ( 0.06856108760741723429, -7.850763007174482055, 9.549252947205623343 ) ) ;
#150843=CARTESIAN_POINT ( 'NONE',  ( 10.99944587961300257, -9.906575223978485667, -0.1104109902703103996 ) ) ;
#150870=VERTEX_POINT ( 'NONE', #67544 ) ;
#150918=CARTESIAN_POINT ( 'NONE',  ( -2.373851744317279522, 1.000000000000000888, 11.76285798163022100 ) ) ;
#150925=DIRECTION ( 'NONE',  ( -0.6691306063588566833, 0.000000000000000000, 0.7431448254773955764 ) ) ;
#150966=DIRECTION ( 'NONE',  ( 0.000000000000000000, 0.000000000000000000, -1.000000000000000000 ) ) ;
#150981=AXIS2_PLACEMENT_3D ( 'NONE', #147300, #48732, #180843 ) ;
#151033=( LENGTH_UNIT ( ) NAMED_UNIT ( * ) SI_UNIT ( .MILLI., .METRE. ) );
#151074=ORIENTED_EDGE ( 'NONE', *, *, #165074, .F. ) ;
#151081=CARTESIAN_POINT ( 'NONE',  ( 6.701130152864326561, -6.864242550357417372, -6.729185449012855535 ) ) ;
#151092=CARTESIAN_POINT ( 'NONE',  ( 0.4294425147611369287, -9.006862915010142245, -9.490288674561773163 ) ) ;
#151093=CARTESIAN_POINT ( 'NONE',  ( 6.845108005540235574, -7.986884274785875704, -6.643335646896346702 ) ) ;
#151102=FACE_OUTER_BOUND ( 'NONE', #163706, .T. ) ;
#151122=B_SPLINE_CURVE_WITH_KNOTS ( 'NONE', 3,
 ( #16008, #65816, #50671, #53881, #37624, #82094, #148187 ),
 .UNSPECIFIED., .F., .F.,
 ( 4, 3, 4 ),
 ( 0.0001788552925466792450, 0.0009000000022260257627, 0.002103779968145169134 ),
 .UNSPECIFIED. ) ;
#151174=PRODUCT_CONTEXT ( 'NONE', #144661, 'mechanical' ) ;
#151210=EDGE_CURVE ( 'NONE', #66793, #180510, #10040, .T. ) ;
#151217=CIRCLE ( 'NONE', #109839, 10.99999999999999112 ) ;
#151231=CARTESIAN_POINT ( 'NONE',  ( 9.581975256308805200, -7.217880409008743392, 3.332261557277432708E-13 ) ) ;
#151257=CARTESIAN_POINT ( 'NONE',  ( -6.735605996566196296E-15, -9.900000000000005684, 9.579665964948942403 ) ) ;
#151277=CARTESIAN_POINT ( 'NONE',  ( -7.966449380362737642, -6.654700410849496706, 7.586197045692401275 ) ) ;
#151294=ORIENTED_EDGE ( 'NONE', *, *, #140838, .T. ) ;
#151305=VECTOR ( 'NONE', #40743, 1000.000000000000000 ) ;
#151317=CARTESIAN_POINT ( 'NONE',  ( 10.96028113393447256, -5.411711732698798905, -0.1309013025973228828 ) ) ;
#151339=AXIS2_PLACEMENT_3D ( 'NONE', #45516, #110566, #108436 ) ;
#151348=CARTESIAN_POINT ( 'NONE',  ( -9.612297698795947198, -6.674536912880607353, 0.2039282260588225759 ) ) ;
#151349=DIRECTION ( 'NONE',  ( -1.535693738322999099E-12, 1.000000000000000000, 1.561558963378103181E-12 ) ) ;
#151352=DIRECTION ( 'NONE',  ( 0.000000000000000000, 0.000000000000000000, -1.000000000000000000 ) ) ;
#151408=CARTESIAN_POINT ( 'NONE',  ( -10.99861980075107937, -9.900000000000074962, 0.1919816227428194633 ) ) ;
#151460=DIRECTION ( 'NONE',  ( 0.000000000000000000, 0.000000000000000000, 1.000000000000000000 ) ) ;
#151464=COLOUR_RGB ( '', 0.66274510, 0.83137255, 0.94901961) ;
#151478=PRESENTATION_STYLE_ASSIGNMENT (( #167713 ) ) ;
#151530=CARTESIAN_POINT ( 'NONE',  ( 8.748013565000626102, 3.829536045110815135, 7.724821879577326911 ) ) ;
#151542=AXIS2_PLACEMENT_3D ( 'NONE', #6402, #187303, #8550 ) ;
#151555=DIRECTION ( 'NONE',  ( -0.000000000000000000, -1.000000000000000000, -0.000000000000000000 ) ) ;
#151564=CARTESIAN_POINT ( 'NONE',  ( 8.758160245764852192, 1.972237431423702114, 7.885882905890388095 ) ) ;
#151596=CARTESIAN_POINT ( 'NONE',  ( 0.07933194154487524519, 7.849261790823902629, -9.499668754385622194 ) ) ;
#151604=CARTESIAN_POINT ( 'NONE',  ( 0.1969747848976802496, -6.717152734873738318, 10.87166355890666480 ) ) ;
#151622=CARTESIAN_POINT ( 'NONE',  ( -9.495541471879707984, -9.135662283479117463, 0.2985557471763422566 ) ) ;
#151627=ADVANCED_FACE ( 'NONE', ( #200537 ), #48800, .T. ) ;
#151646=CARTESIAN_POINT ( 'NONE',  ( 9.567965691386879357, -9.756398209953340839, -0.1670094623740806250 ) ) ;
#151656=AXIS2_PLACEMENT_3D ( 'NONE', #191019, #59969, #123997 ) ;
#151664=FILL_AREA_STYLE_COLOUR ( '', #137861 ) ;
#151703=ORIENTED_EDGE ( 'NONE', *, *, #49463, .T. ) ;
#151704=SURFACE_STYLE_USAGE ( .BOTH. , #71478 ) ;
#151739=CARTESIAN_POINT ( 'NONE',  ( 7.860745937262095140, -5.389939693150812339, -7.694877102302460692 ) ) ;
#151754=VERTEX_POINT ( 'NONE', #192823 ) ;
#151756=CARTESIAN_POINT ( 'NONE',  ( 9.797921721691059460, 3.956598013261175772, 6.103348209225848642 ) ) ;
#151827=CARTESIAN_POINT ( 'NONE',  ( -7.401194801147281233, -6.836289462023139585, -7.952857047017147352 ) ) ;
#151857=EDGE_CURVE ( 'NONE', #35104, #214101, #199717, .T. ) ;
#151866=CARTESIAN_POINT ( 'NONE',  ( 7.834948825496932834, -9.999999999999994671, 7.720982897393586342 ) ) ;
#151870=CARTESIAN_POINT ( 'NONE',  ( -6.761669295867164031, -7.008190897455700785, -6.673079560224742579 ) ) ;
#151875=CARTESIAN_POINT ( 'NONE',  ( -6.773376336900938099, -7.645781813054123965, -6.661184053808324457 ) ) ;
#151894=CARTESIAN_POINT ( 'NONE',  ( 6.776370306708059843, -7.161464053357565973, 6.781144757626057284 ) ) ;
#151896=B_SPLINE_CURVE_WITH_KNOTS ( 'NONE', 3,
 ( #64497, #196631, #145791, #99139, #180380, #181431 ),
 .UNSPECIFIED., .F., .F.,
 ( 4, 2, 4 ),
 ( 0.000000000000000000, 0.0003147459536107448494, 0.0006294919072214896988 ),
 .UNSPECIFIED. ) ;
#151898=DIRECTION ( 'NONE',  ( 0.03984146075563036599, -3.484297484818016589E-16, 0.9992060137953822085 ) ) ;
#151902=CARTESIAN_POINT ( 'NONE',  ( 10.99952653502853117, -9.917017194762472343, -0.1020740558599437658 ) ) ;
#151906=CARTESIAN_POINT ( 'NONE',  ( 6.903494779225153977, -6.732807188596972026, -6.688963559358321653 ) ) ;
#151933=CARTESIAN_POINT ( 'NONE',  ( -10.48884024596653397, 1.000000000000000888, 5.608780650328914597 ) ) ;
#151935=EDGE_CURVE ( 'NONE', #139509, #119003, #75281, .T. ) ;
#151941=B_SPLINE_CURVE_WITH_KNOTS ( 'NONE', 3,
 ( #45230, #109220, #191440, #42034, #92919, #60382, #208757, #128682 ),
 .UNSPECIFIED., .F., .F.,
 ( 4, 2, 2, 4 ),
 ( 0.000000000000000000, 0.0001985720215089326513, 0.0003971440430178653025, 0.0007942880860357295209 ),
 .UNSPECIFIED. ) ;
#151992=FILL_AREA_STYLE ('',( #21943 ) ) ;
#151998=ADVANCED_FACE ( 'NONE', ( #139853 ), #33597, .F. ) ;
#152034=CARTESIAN_POINT ( 'NONE',  ( 7.777967379493318845, -5.907420853759296264, 7.664830294503448549 ) ) ;
#152036=ORIENTED_EDGE ( 'NONE', *, *, #165074, .T. ) ;
#152052=CARTESIAN_POINT ( 'NONE',  ( -0.07933194154489606187, -9.746166700180788567, -9.499668754385620417 ) ) ;
#152080=EDGE_CURVE ( 'NONE', #144861, #135108, #110919, .T. ) ;
#152090=CARTESIAN_POINT ( 'NONE',  ( 6.794158526849249924, -7.616254850791396969, 7.451274665340253733 ) ) ;
#152104=ORIENTED_EDGE ( 'NONE', *, *, #183643, .T. ) ;
#152131=CARTESIAN_POINT ( 'NONE',  ( 9.612297698795886802, -6.674536912880676631, -0.2039282260587966522 ) ) ;
#152181=CARTESIAN_POINT ( 'NONE',  ( 11.00029519899100627, -5.907420853759282942, 5.448115916739660570E-15 ) ) ;
#152214=CARTESIAN_POINT ( 'NONE',  ( 10.91970695577495043, -5.907420853759282053, 8.673617379884035472E-15 ) ) ;
#152235=FACE_OUTER_BOUND ( 'NONE', #4739, .T. ) ;
#152263=CIRCLE ( 'NONE', #96941, 0.08000000000000020983 ) ;
#152267=( BOUNDED_SURFACE ( )  B_SPLINE_SURFACE ( 3, 2, ( 
 ( #143979, #107234, #73592 ),
 ( #175381, #176437, #174324 ),
 ( #205716, #192659, #76784 ),
 ( #209970, #11782, #24836 ) ),
 .UNSPECIFIED., .F., .F., .T. ) 
 B_SPLINE_SURFACE_WITH_KNOTS ( ( 4, 4 ),
 ( 3, 3 ),
 ( 0.005241070803109276581, 0.008267458746840841005 ),
 ( 0.000000000000000000, 1.000000000000000000 ),
 .UNSPECIFIED. ) 
 GEOMETRIC_REPRESENTATION_ITEM ( )  RATIONAL_B_SPLINE_SURFACE ( (
 ( 1.000000000000000000, 0.7184380228464076756, 1.000000000000000000),
 ( 1.000000000000000000, 0.7185467277397525887, 1.000000000000000000),
 ( 1.000000000000000000, 0.7186585579881041852, 1.000000000000000000),
 ( 1.000000000000000000, 0.7187737999613678097, 1.000000000000000000) ) ) 
 REPRESENTATION_ITEM ( '' )  SURFACE ( )  );
#152287=SURFACE_STYLE_FILL_AREA ( #21181 ) ;
#152338=CARTESIAN_POINT ( 'NONE',  ( -10.75419052074085080, -7.927673425445466826, 0.6248749548428326195 ) ) ;
#152359=EDGE_LOOP ( 'NONE', ( #39723, #41200, #75005, #20615 ) ) ;
#152378=ORIENTED_EDGE ( 'NONE', *, *, #3571, .T. ) ;
#152407=( NAMED_UNIT ( * ) PLANE_ANGLE_UNIT ( ) SI_UNIT ( $, .RADIAN. ) );
#152513=DIRECTION ( 'NONE',  ( -0.6123724356957848114, 0.7071067811865540120, 0.3535533905932775611 ) ) ;
#152537=CARTESIAN_POINT ( 'NONE',  ( -9.499633399276474321, -8.038540703696495981, 0.09463244300327114389 ) ) ;
#152559=CARTESIAN_POINT ( 'NONE',  ( -0.4368516432692234330, -5.631911363926715985, -10.55905904256945860 ) ) ;
#152607=ORIENTED_EDGE ( 'NONE', *, *, #175600, .T. ) ;
#152609=AXIS2_PLACEMENT_3D ( 'NONE', #122653, #57560, #202713 ) ;
#152653=CIRCLE ( 'NONE', #190825, 10.24999999999998934 ) ;
#152656=CARTESIAN_POINT ( 'NONE',  ( -7.142181811248260459E-15, -6.134628647623513231, 11.00029519899099917 ) ) ;
#152689=CARTESIAN_POINT ( 'NONE',  ( 0.001745240643721140961, -9.900000000000005684, 0.09998476951564826132 ) ) ;
#152697=CARTESIAN_POINT ( 'NONE',  ( -1.138412281109779656E-15, -6.681160345272285639, -10.14529669463342820 ) ) ;
#152702=LINE ( 'NONE', #200363, #209115 ) ;
#152712=VECTOR ( 'NONE', #170153, 1000.000000000000000 ) ;
#152739=CIRCLE ( 'NONE', #170046, 0.08000000000000020983 ) ;
#152751=ORIENTED_EDGE ( 'NONE', *, *, #89522, .T. ) ;
#152763=ADVANCED_FACE ( 'NONE', ( #106351 ), #122267, .F. ) ;
#152781=EDGE_CURVE ( 'NONE', #133641, #209973, #206831, .T. ) ;
#152790=FACE_OUTER_BOUND ( 'NONE', #191535, .T. ) ;
#152831=EDGE_CURVE ( 'NONE', #172003, #72609, #149600, .T. ) ;
#152833=ORIENTED_EDGE ( 'NONE', *, *, #7723, .T. ) ;
#152838=CARTESIAN_POINT ( 'NONE',  ( -1.040834085586084257E-14, -9.746166700180788567, -9.579665964948867796 ) ) ;
#152878=CARTESIAN_POINT ( 'NONE',  ( -7.586197045692500751, -6.654700410849692993, -7.966449380362629284 ) ) ;
#152899=EDGE_CURVE ( 'NONE', #14256, #107724, #96171, .T. ) ;
#152922=CARTESIAN_POINT ( 'NONE',  ( -6.447267651612378359, -6.532648833121157850, -6.949925879317520483 ) ) ;
#152927=FACE_OUTER_BOUND ( 'NONE', #91557, .T. ) ;
#152929=CARTESIAN_POINT ( 'NONE',  ( 9.499734081922104778, -9.919612995835008107, -0.07111086427374714580 ) ) ;
#152940=EDGE_CURVE ( 'NONE', #200355, #50012, #199862, .T. ) ;
#152956=DIRECTION ( 'NONE',  ( 0.01745240643728004568, 0.000000000000000000, 0.9998476951563912696 ) ) ;
#152963=CARTESIAN_POINT ( 'NONE',  ( 6.796206128891365772, -7.030236945367178691, -6.776587425048098190 ) ) ;
#152966=CIRCLE ( 'NONE', #208297, 0.08000000000000020983 ) ;
#152986=CARTESIAN_POINT ( 'NONE',  ( -0.02191154088443912629, -9.962467531990274239, -9.579628365760338937 ) ) ;
#153014=ORIENTED_EDGE ( 'NONE', *, *, #197793, .F. ) ;
#153018=ADVANCED_FACE ( 'NONE', ( #191792, #95409 ), #75929, .T. ) ;
#153026=VECTOR ( 'NONE', #185040, 1000.000000000000000 ) ;
#153044=CARTESIAN_POINT ( 'NONE',  ( 6.717278222822382183, -7.473374494058092843, -6.750415307812249743 ) ) ;
#153107=ORIENTED_EDGE ( 'NONE', *, *, #73338, .F. ) ;
#153112=FILL_AREA_STYLE ('',( #122848 ) ) ;
#153113=ORIENTED_EDGE ( 'NONE', *, *, #73338, .T. ) ;
#153115=( GEOMETRIC_REPRESENTATION_CONTEXT ( 3 ) GLOBAL_UNCERTAINTY_ASSIGNED_CONTEXT ( ( #192988 ) ) GLOBAL_UNIT_ASSIGNED_CONTEXT ( ( #110478, #160225, #126742 ) ) REPRESENTATION_CONTEXT ( 'NONE', 'WORKASPACE' ) );
#153193=ORIENTED_EDGE ( 'NONE', *, *, #7856, .F. ) ;
#153200=ORIENTED_EDGE ( 'NONE', *, *, #40921, .F. ) ;
#153215=EDGE_CURVE ( 'NONE', #65129, #103298, #210232, .T. ) ;
#153295=FACE_BOUND ( 'NONE', #212277, .T. ) ;
#153318=CARTESIAN_POINT ( 'NONE',  ( -2.173285075505815599E-15, -8.011313137147263674, 11.00000000000000178 ) ) ;
#153325=MECHANICAL_DESIGN_GEOMETRIC_PRESENTATION_REPRESENTATION('',(#35651),#84054);
#153346=AXIS2_PLACEMENT_3D ( 'NONE', #106781, #124138, #137106 ) ;
#153350=ORIENTED_EDGE ( 'NONE', *, *, #174069, .F. ) ;
#153353=CARTESIAN_POINT ( 'NONE',  ( -10.18278199833531517, 3.974415841077576950, 5.432519183637573690 ) ) ;
#153360=CARTESIAN_POINT ( 'NONE',  ( -10.20626665084797580, 3.700502905159950728, -5.921468070729088318 ) ) ;
#153369=CARTESIAN_POINT ( 'NONE',  ( 10.99529341469513533, -7.794776013890245991, -0.3288329489799977634 ) ) ;
#153405=EDGE_CURVE ( 'NONE', #195316, #127089, #38336, .T. ) ;
#153407=CARTESIAN_POINT ( 'NONE',  ( 0.000000000000000000, -6.583980363594990948, 0.000000000000000000 ) ) ;
#153420=EDGE_CURVE ( 'NONE', #172181, #173465, #99636, .T. ) ;
#153430=ORIENTED_EDGE ( 'NONE', *, *, #165205, .F. ) ;
#153432=CARTESIAN_POINT ( 'NONE',  ( -10.91864124492992616, -9.978085788838701120, 0.1530507449821368049 ) ) ;
#153438=B_SPLINE_CURVE_WITH_KNOTS ( 'NONE', 3,
 ( #203687, #59589, #190642, #8702 ),
 .UNSPECIFIED., .F., .F.,
 ( 4, 4 ),
 ( 0.000000000000000000, 6.033646489354572420E-05 ),
 .UNSPECIFIED. ) ;
#153461=ORIENTED_EDGE ( 'NONE', *, *, #147708, .F. ) ;
#153463=FACE_OUTER_BOUND ( 'NONE', #72987, .T. ) ;
#153487=AXIS2_PLACEMENT_3D ( 'NONE', #17232, #83307, #67042 ) ;
#153565=B_SPLINE_CURVE_WITH_KNOTS ( 'NONE', 3,
 ( #208554, #164892, #110082, #132438, #175035, #27693, #143625 ),
 .UNSPECIFIED., .F., .F.,
 ( 4, 3, 4 ),
 ( 0.0001126021369352535047, 0.001495765174703663240, 0.002006790696433110015 ),
 .UNSPECIFIED. ) ;
#153580=ORIENTED_EDGE ( 'NONE', *, *, #7723, .F. ) ;
#153585=CARTESIAN_POINT ( 'NONE',  ( 9.499606442108964544, -9.900000000000005684, -0.08647222121513538362 ) ) ;
#153590=DIRECTION ( 'NONE',  ( 0.7384114592165670343, 0.000000000000000000, -0.6743504407188151140 ) ) ;
#153607=CARTESIAN_POINT ( 'NONE',  ( -3.371191130072114856E-16, 3.975933801733733564, -11.54759062144378845 ) ) ;
#153626=CARTESIAN_POINT ( 'NONE',  ( 0.000000000000000000, 0.000000000000000000, 0.000000000000000000 ) ) ;
#153644=DIRECTION ( 'NONE',  ( 1.000000000000000000, 0.000000000000000000, -1.224646799147353207E-16 ) ) ;
#153661=CYLINDRICAL_SURFACE ( 'NONE', #82964, 6.249999999999995559 ) ;
#153664=CARTESIAN_POINT ( 'NONE',  ( -6.280867513185877376E-15, -8.256136661604328353, 10.93205753685578330 ) ) ;
#153685=EDGE_LOOP ( 'NONE', ( #130248, #85673, #62007, #87751 ) ) ;
#153693=AXIS2_PLACEMENT_3D ( 'NONE', #67809, #51613, #1753 ) ;
#153707=DIRECTION ( 'NONE',  ( 0.000000000000000000, 0.000000000000000000, 1.000000000000000000 ) ) ;
#153719=ORIENTED_EDGE ( 'NONE', *, *, #50950, .F. ) ;
#153728=CARTESIAN_POINT ( 'NONE',  ( 0.4694063952341809287, -6.700000000000007283, 10.98997987423604172 ) ) ;
#153750=CARTESIAN_POINT ( 'NONE',  ( 0.08058608058606961388, -6.134628647623513231, -10.99970480893079738 ) ) ;
#153751=ORIENTED_EDGE ( 'NONE', *, *, #107978, .F. ) ;
#153769=CARTESIAN_POINT ( 'NONE',  ( -1.138412281109779656E-15, -5.530538574611999714, -11.29689844398641974 ) ) ;
#153789=CIRCLE ( 'NONE', #57000, 0.08000000000000002942 ) ;
#153800=CARTESIAN_POINT ( 'NONE',  ( -10.39230484541327648, 3.499999999999989342, -5.999999999999976019 ) ) ;
#153819=CARTESIAN_POINT ( 'NONE',  ( 9.499640643549723151, -8.037485387949198312, -0.09382487309179397827 ) ) ;
#153840=CARTESIAN_POINT ( 'NONE',  ( -11.41267819554183127, 3.447199233515635619, 3.708203932499423150 ) ) ;
#153910=CARTESIAN_POINT ( 'NONE',  ( -8.081892667527540652, -5.166862915010159263, 7.462104991928526054 ) ) ;
#153923=CARTESIAN_POINT ( 'NONE',  ( 0.000000000000000000, 0.03624871340549007392, 0.000000000000000000 ) ) ;
#153926=CARTESIAN_POINT ( 'NONE',  ( 9.537847510268184337, -7.985988503423661733, -0.1421055763938764704 ) ) ;
#153930=CARTESIAN_POINT ( 'NONE',  ( 0.000000000000000000, 4.000000000000003553, 0.000000000000000000 ) ) ;
#153949=CIRCLE ( 'NONE', #198898, 11.99999999999999112 ) ;
#153953=CARTESIAN_POINT ( 'NONE',  ( -7.455003611050273982, -6.808400134080597965, -7.905503641038500895 ) ) ;
#153987=CARTESIAN_POINT ( 'NONE',  ( 0.000000000000000000, -2.000000000000001776, 0.000000000000000000 ) ) ;
#154025=CARTESIAN_POINT ( 'NONE',  ( 6.770610912236884715, -7.154544010627095219, 6.663994888585883736 ) ) ;
#154057=CARTESIAN_POINT ( 'NONE',  ( -8.915975476025518986, 3.467171072964058354, -8.027980377473689089 ) ) ;
#154111=CARTESIAN_POINT ( 'NONE',  ( 0.04536292375656306164, -10.00000000000004441, 10.91964218157388267 ) ) ;
#154151=DIRECTION ( 'NONE',  ( 0.000000000000000000, 1.000000000000000000, 0.000000000000000000 ) ) ;
#154161=CIRCLE ( 'NONE', #181808, 6.249999999999995559 ) ;
#154170=ORIENTED_EDGE ( 'NONE', *, *, #110743, .T. ) ;
#154186=ORIENTED_EDGE ( 'NONE', *, *, #119166, .T. ) ;
#154192=CARTESIAN_POINT ( 'NONE',  ( -6.725445687907775749, -7.162053774861877997, 6.710127771514615702 ) ) ;
#154244=CARTESIAN_POINT ( 'NONE',  ( -0.07933194154488912297, 7.849261790823902629, 9.499668754385634628 ) ) ;
#154282=DIRECTION ( 'NONE',  ( 0.000000000000000000, 0.000000000000000000, 1.000000000000000000 ) ) ;
#154289=CARTESIAN_POINT ( 'NONE',  ( 0.07933194154487524519, -9.609467486116976431, 9.499668754385634628 ) ) ;
#154316=CARTESIAN_POINT ( 'NONE',  ( -7.721398836998398352, -5.907420853759296264, -7.721398836998357496 ) ) ;
#154326=CARTESIAN_POINT ( 'NONE',  ( 0.000000000000000000, -0.9200000000000041478, -10.91999999999999105 ) ) ;
#154344=CARTESIAN_POINT ( 'NONE',  ( -10.99866081003794882, -6.614835951978810691, 0.2118258318329558909 ) ) ;
#154365=EDGE_CURVE ( 'NONE', #175139, #31187, #142582, .T. ) ;
#154368=STYLED_ITEM ( 'NONE', ( #192294 ), #15528 ) ;
#154407=EDGE_LOOP ( 'NONE', ( #50278, #146418, #48920, #88438 ) ) ;
#154432=PLANE ( 'NONE',  #18103 ) ;
#154467=AXIS2_PLACEMENT_3D ( 'NONE', #46207, #163148, #47280 ) ;
#154503=CARTESIAN_POINT ( 'NONE',  ( -10.91893890296302772, -9.990657656777852225, 0.1342453211083811382 ) ) ;
#154559=EDGE_CURVE ( 'NONE', #199252, #69312, #151896, .T. ) ;
#154576=CARTESIAN_POINT ( 'NONE',  ( 10.08385610902499963, -7.605490242282785474, -0.4645879755154048718 ) ) ;
#154683=ORIENTED_EDGE ( 'NONE', *, *, #82531, .F. ) ;
#154718=FACE_OUTER_BOUND ( 'NONE', #199654, .T. ) ;
#154727=CARTESIAN_POINT ( 'NONE',  ( -7.821934338880100590, -6.709380320845385270, 7.553974597844393735 ) ) ;
#154781=CARTESIAN_POINT ( 'NONE',  ( -1.730579034767993219E-05, -9.953931234596399946, -9.500331159997283947 ) ) ;
#154795=FACE_OUTER_BOUND ( 'NONE', #92353, .T. ) ;
#154801=CARTESIAN_POINT ( 'NONE',  ( 2.494940289813108780, 3.447199233515649386, -11.73777120880564695 ) ) ;
#154856=AXIS2_PLACEMENT_3D ( 'NONE', #44255, #176381, #94083 ) ;
#154933=ORIENTED_EDGE ( 'NONE', *, *, #207563, .F. ) ;
#154948=CARTESIAN_POINT ( 'NONE',  ( 0.1236583036082015280, 1.000000000000000888, -11.99936284241577233 ) ) ;
#154963=CARTESIAN_POINT ( 'NONE',  ( 0.000000000000000000, 0.000000000000000000, 0.000000000000000000 ) ) ;
#154983=CARTESIAN_POINT ( 'NONE',  ( 0.08058608058606961388, -6.134628647623513231, -10.99970480893079738 ) ) ;
#154988=CARTESIAN_POINT ( 'NONE',  ( 9.512045263456263555, -8.176568542494905500, -0.4655551865852067817 ) ) ;
#154990=CARTESIAN_POINT ( 'NONE',  ( 0.000000000000000000, -9.919999999999998153, 0.000000000000000000 ) ) ;
#155013=FACE_OUTER_BOUND ( 'NONE', #99391, .T. ) ;
#155014=CARTESIAN_POINT ( 'NONE',  ( -4.218316008240990271E-13, -9.350066838357692589, -9.500000000000001776 ) ) ;
#155019=ORIENTED_EDGE ( 'NONE', *, *, #135163, .F. ) ;
#155087=ORIENTED_EDGE ( 'NONE', *, *, #132620, .F. ) ;
#155092=CARTESIAN_POINT ( 'NONE',  ( 6.729185449012857312, -6.864242550357277040, 6.701130152864321232 ) ) ;
#155116=ADVANCED_FACE ( 'NONE', ( #150016 ), #111460, .T. ) ;
#155128=DIRECTION ( 'NONE',  ( 0.000000000000000000, 0.000000000000000000, 1.000000000000000000 ) ) ;
#155215=EDGE_CURVE ( 'NONE', #38980, #103298, #120653, .T. ) ;
#155217=CARTESIAN_POINT ( 'NONE',  ( -9.499668754385632852, -7.246166700194470067, -0.07933194154487524519 ) ) ;
#155244=DIRECTION ( 'NONE',  ( -0.04529798058948674572, 1.504112749676232550E-16, -0.9989735196462989908 ) ) ;
#155252=ORIENTED_EDGE ( 'NONE', *, *, #161057, .T. ) ;
#155258=CARTESIAN_POINT ( 'NONE',  ( 0.000000000000000000, -7.473374494045017968, 9.579665964948883783 ) ) ;
#155297=CARTESIAN_POINT ( 'NONE',  ( -6.717748655459638840, -7.246166700180801001, -6.717748655459603313 ) ) ;
#155303=ORIENTED_EDGE ( 'NONE', *, *, #38423, .T. ) ;
#155326=ORIENTED_EDGE ( 'NONE', *, *, #183561, .F. ) ;
#155350=CARTESIAN_POINT ( 'NONE',  ( 0.07933194154487524519, -9.746166700180788567, 9.499668754385634628 ) ) ;
#155359=CARTESIAN_POINT ( 'NONE',  ( 0.08172171391242558092, -9.906619969460795261, 10.99969643042367018 ) ) ;
#155378=( GEOMETRIC_REPRESENTATION_CONTEXT ( 3 ) GLOBAL_UNCERTAINTY_ASSIGNED_CONTEXT ( ( #3806 ) ) GLOBAL_UNIT_ASSIGNED_CONTEXT ( ( #124958, #174717, #76120 ) ) REPRESENTATION_CONTEXT ( 'NONE', 'WORKASPACE' ) );
#155393=VERTEX_POINT ( 'NONE', #180917 ) ;
#155423=DIRECTION ( 'NONE',  ( 0.000000000000000000, 1.000000000000000000, 0.000000000000000000 ) ) ;
#155445=PRESENTATION_STYLE_ASSIGNMENT (( #43858 ) ) ;
#155466=B_SPLINE_CURVE_WITH_KNOTS ( 'NONE', 3,
 ( #43358, #173359, #26006, #11889 ),
 .UNSPECIFIED., .F., .F.,
 ( 4, 4 ),
 ( 0.000000000000000000, 0.0002908967400263835030 ),
 .UNSPECIFIED. ) ;
#155504=CARTESIAN_POINT ( 'NONE',  ( -9.499685679921610060, -9.917013740047297077, 0.07729799388535862903 ) ) ;
#155505=CARTESIAN_POINT ( 'NONE',  ( 10.99665086521320845, -7.860092950639685938, -0.2746580110251511386 ) ) ;
#155523=CARTESIAN_POINT ( 'NONE',  ( 6.773846765307987461, -7.473374494058229622, 6.773846765307971474 ) ) ;
#155547=FACE_OUTER_BOUND ( 'NONE', #47985, .T. ) ;
#155599=DIRECTION ( 'NONE',  ( 0.000000000000000000, -1.000000000000000000, 0.000000000000000000 ) ) ;
#155612=FACE_OUTER_BOUND ( 'NONE', #201662, .T. ) ;
#155615=SURFACE_SIDE_STYLE ('',( #40813 ) ) ;
#155637=DIRECTION ( 'NONE',  ( -0.9992060137953822085, 8.739303527495176105E-16, -0.03984146075563037293 ) ) ;
#155651=CARTESIAN_POINT ( 'NONE',  ( -6.922231005658575853, -8.202869699938529990, 6.506745451169506644 ) ) ;
#155659=DIRECTION ( 'NONE',  ( -1.000000000000000000, -0.000000000000000000, -0.000000000000000000 ) ) ;
#155669=AXIS2_PLACEMENT_3D ( 'NONE', #74185, #91519, #24331 ) ;
#155688=( BOUNDED_SURFACE ( )  B_SPLINE_SURFACE ( 3, 2, ( 
 ( #138837, #104196, #171311 ),
 ( #89022, #6663, #73818 ),
 ( #79144, #14119, #93297 ),
 ( #13065, #43478, #193957 ) ),
 .UNSPECIFIED., .F., .F., .T. ) 
 B_SPLINE_SURFACE_WITH_KNOTS ( ( 4, 4 ),
 ( 3, 3 ),
 ( 0.000000000000000000, 9.170893477967426329E-05 ),
 ( 0.000000000000000000, 1.000000000000000000 ),
 .UNSPECIFIED. ) 
 GEOMETRIC_REPRESENTATION_ITEM ( )  RATIONAL_B_SPLINE_SURFACE ( (
 ( 1.000000000000000000, 0.6787756258918241636, 1.000000000000000000),
 ( 1.000000000000000000, 0.6894756946173401513, 1.000000000000000000),
 ( 1.000000000000000000, 0.6998898451713442270, 1.000000000000000000),
 ( 1.000000000000000000, 0.7100530722072168066, 1.000000000000000000) ) ) 
 REPRESENTATION_ITEM ( '' )  SURFACE ( )  );
#155795=CARTESIAN_POINT ( 'NONE',  ( -9.481348452320357723, -9.199999999999983302, 0.5950054837414385789 ) ) ;
#155817=DIRECTION ( 'NONE',  ( -0.000000000000000000, 1.000000000000000000, -0.000000000000000000 ) ) ;
#155862=CARTESIAN_POINT ( 'NONE',  ( 0.2970643657731242282, -6.863149499369272988, 10.99622371251743225 ) ) ;
#155868=CARTESIAN_POINT ( 'NONE',  ( -1.958975448762383504E-15, -9.746166700180790343, -9.500331257164614129 ) ) ;
#155869=CARTESIAN_POINT ( 'NONE',  ( 10.94228617828407124, -8.109732095436330113, -0.2200370843778234053 ) ) ;
#155877=CARTESIAN_POINT ( 'NONE',  ( -10.94228617828407302, -8.109732095436331889, 0.2200370843778256258 ) ) ;
#155879=CARTESIAN_POINT ( 'NONE',  ( -8.103009739377986520, -6.893137084989842123, 7.439168848974023973 ) ) ;
#155887=CARTESIAN_POINT ( 'NONE',  ( -6.922777049148908013, -8.203199116536525892, 6.506163559800182128 ) ) ;
#155896=DIRECTION ( 'NONE',  ( 0.000000000000000000, 1.000000000000000000, 0.000000000000000000 ) ) ;
#155903=ADVANCED_FACE ( 'NONE', ( #5011 ), #71084, .T. ) ;
#155904=CARTESIAN_POINT ( 'NONE',  ( 10.39398850336073643, -8.287668210030899374, -0.6181847325714995289 ) ) ;
#155923=CARTESIAN_POINT ( 'NONE',  ( 0.4370080631058587683, -8.003595416197011758, -10.68747925529770271 ) ) ;
#155951=UNCERTAINTY_MEASURE_WITH_UNIT (LENGTH_MEASURE( 1.000000000000000082E-05 ), #39291, 'distance_accuracy_value', 'NONE');
#156027=CARTESIAN_POINT ( 'NONE',  ( 0.07538891330675548397, -7.154544010627095219, -9.499700864329911454 ) ) ;
#156031=CARTESIAN_POINT ( 'NONE',  ( 10.90207482560801999, -7.666862915010147717, -0.6254314485565921622 ) ) ;
#156034=EDGE_CURVE ( 'NONE', #181416, #82411, #209023, .T. ) ;
#156054=MANIFOLD_SOLID_BREP ( 'Fillet7', #146810 ) ;
#156061=DIRECTION ( 'NONE',  ( -0.9980366791916180924, 0.000000000000000000, 0.06263215618328135670 ) ) ;
#156085=CARTESIAN_POINT ( 'NONE',  ( -8.845566791370137238, 3.603011019375353285, -7.955782632700151069 ) ) ;
#156087=EDGE_CURVE ( 'NONE', #180510, #22857, #198271, .T. ) ;
#156126=FACE_OUTER_BOUND ( 'NONE', #167467, .T. ) ;
#156127=EDGE_LOOP ( 'NONE', ( #77056, #153200, #135601, #5439, #123701 ) ) ;
#156148=CARTESIAN_POINT ( 'NONE',  ( 7.100579091573050228, -6.583980363594990948, -6.484567079770450881 ) ) ;
#156151=FACE_OUTER_BOUND ( 'NONE', #95694, .T. ) ;
#156157=EDGE_CURVE ( 'NONE', #131570, #157711, #188053, .T. ) ;
#156172=ORIENTED_EDGE ( 'NONE', *, *, #208381, .F. ) ;
#156260=CARTESIAN_POINT ( 'NONE',  ( 0.000000000000000000, -9.746166700180788567, 9.579665964948883783 ) ) ;
#156264=PRESENTATION_STYLE_ASSIGNMENT (( #141111 ) ) ;
#156276=EDGE_LOOP ( 'NONE', ( #132069, #33372, #98820, #47485, #179907, #90324, #127529, #186353, #24470, #98614, #141163, #134995, #131880, #49210, #48927, #38609, #47087, #94505, #42225, #151703, #209664 ) ) ;
#156326=DIRECTION ( 'NONE',  ( 0.000000000000000000, 0.000000000000000000, -1.000000000000000000 ) ) ;
#156348=CARTESIAN_POINT ( 'NONE',  ( -0.07804503809600779607, -9.997560133496188328, -10.91958144425261423 ) ) ;
#156377=STYLED_ITEM ( 'NONE', ( #60584 ), #62018 ) ;
#156385=CARTESIAN_POINT ( 'NONE',  ( -0.3852658704378487120, -6.836271227032193032, -10.85717823004578264 ) ) ;
#156404=LINE ( 'NONE', #170499, #56217 ) ;
#156415=CIRCLE ( 'NONE', #38751, 9.499999999999992895 ) ;
#156429=CARTESIAN_POINT ( 'NONE',  ( -0.06269018847469841338, -7.008739397177404129, 9.499801640457409491 ) ) ;
#156473=DIRECTION ( 'NONE',  ( 0.000000000000000000, 1.000000000000000000, 0.000000000000000000 ) ) ;
#156490=CARTESIAN_POINT ( 'NONE',  ( -10.87166355890668790, -6.717152734873728548, 0.1969747848976953764 ) ) ;
#156531=AXIS2_PLACEMENT_3D ( 'NONE', #134260, #151555, #69192 ) ;
#156545=CARTESIAN_POINT ( 'NONE',  ( -0.09775709102117645377, -9.919835437265268396, -10.99956570265432454 ) ) ;
#156550=ORIENTED_EDGE ( 'NONE', *, *, #148852, .F. ) ;
#156555=LINE ( 'NONE', #190097, #142549 ) ;
#156595=( GEOMETRIC_REPRESENTATION_CONTEXT ( 3 ) GLOBAL_UNCERTAINTY_ASSIGNED_CONTEXT ( ( #95231 ) ) GLOBAL_UNIT_ASSIGNED_CONTEXT ( ( #120207, #165559, #198048 ) ) REPRESENTATION_CONTEXT ( 'NONE', 'WORKASPACE' ) );
#156599=CARTESIAN_POINT ( 'NONE',  ( 6.643335646896344038, -7.986884274785886362, 6.845108005540233798 ) ) ;
#156627=CIRCLE ( 'NONE', #104828, 10.99999999999999112 ) ;
#156657=B_SPLINE_CURVE_WITH_KNOTS ( 'NONE', 3,
 ( #175621, #126943, #27208, #93314, #159350, #12025, #207024, #173499, #56525, #157236 ),
 .UNSPECIFIED., .F., .F.,
 ( 4, 2, 2, 2, 4 ),
 ( 2.453269466693236920E-18, 0.0002503535593264603985, 0.0005007071186529184117, 0.0007510606779793763165, 0.001001414237305834221 ),
 .UNSPECIFIED. ) ;
#156661=ORIENTED_EDGE ( 'NONE', *, *, #212430, .F. ) ;
#156688=CARTESIAN_POINT ( 'NONE',  ( -11.41267819554183127, 3.447199233515635619, 3.708203932499423150 ) ) ;
#156758=EDGE_CURVE ( 'NONE', #56213, #182554, #139968, .T. ) ;
#156791=VERTEX_POINT ( 'NONE', #179303 ) ;
#156801=CARTESIAN_POINT ( 'NONE',  ( -0.1000000000000028644, -9.999999999999994671, -9.579478065113972818 ) ) ;
#156808=CARTESIAN_POINT ( 'NONE',  ( -0.2435857797690326454, -7.709701271428947678, 10.99755231369147523 ) ) ;
#156820=ORIENTED_EDGE ( 'NONE', *, *, #186606, .T. ) ;
#156839=CONICAL_SURFACE ( 'NONE', #143108, 11.53746066217574473, 0.1181278931043537039 ) ;
#156849=CARTESIAN_POINT ( 'NONE',  ( -6.701130199342137495, -6.864242587301023768, 6.729185404178084084 ) ) ;
#156873=CARTESIAN_POINT ( 'NONE',  ( -0.2721095781817652881, -7.697284395437295146, 10.99684423689256008 ) ) ;
#156878=CARTESIAN_POINT ( 'NONE',  ( -0.2897211420239401147, -7.754973434576984737, 10.97056425546335845 ) ) ;
#156952=( NAMED_UNIT ( * ) SI_UNIT ( $, .STERADIAN. ) SOLID_ANGLE_UNIT ( ) );
#156955=SURFACE_STYLE_FILL_AREA ( #141802 ) ;
#156956=CARTESIAN_POINT ( 'NONE',  ( 4.593150236022219428E-15, -8.011313137147251240, -11.00000000000000178 ) ) ;
#156957=ADVANCED_FACE ( 'NONE', ( #98059 ), #197654, .F. ) ;
#156962=CARTESIAN_POINT ( 'NONE',  ( -6.661184053808019812, -7.645781813054106202, 6.773376336901249850 ) ) ;
#156964=ORIENTED_EDGE ( 'NONE', *, *, #176622, .T. ) ;
#156972=CARTESIAN_POINT ( 'NONE',  ( -9.569423160901790126, -7.256398209936431698, 1.138412281109779656E-15 ) ) ;
#156973=DIRECTION ( 'NONE',  ( 0.000000000000000000, -1.000000000000000000, 0.000000000000000000 ) ) ;
#157116=CARTESIAN_POINT ( 'NONE',  ( -7.893838479094924310, -5.325441678136489720, 7.661067326845521386 ) ) ;
#157131=CARTESIAN_POINT ( 'NONE',  ( -10.07455280567990563, 1.264806443676224301, -6.263461699855405129 ) ) ;
#157133=CARTESIAN_POINT ( 'NONE',  ( -6.773846765317318663, 0.000000000000000000, 6.773846765317342644 ) ) ;
#157147=CARTESIAN_POINT ( 'NONE',  ( 0.008366613517340512618, 2.629643693813621397, -12.00001160347414775 ) ) ;
#157153=ORIENTED_EDGE ( 'NONE', *, *, #33674, .F. ) ;
#157184=ORIENTED_EDGE ( 'NONE', *, *, #194076, .F. ) ;
#157192=CARTESIAN_POINT ( 'NONE',  ( 0.000000000000000000, 3.956598013261175772, 0.000000000000000000 ) ) ;
#157211=CARTESIAN_POINT ( 'NONE',  ( -10.99943592164172834, -9.900000000000005684, 0.1113975120798846308 ) ) ;
#157235=CARTESIAN_POINT ( 'NONE',  ( 0.06258739273032451478, -9.383611379567494026, -9.609645335164882951 ) ) ;
#157236=CARTESIAN_POINT ( 'NONE',  ( -7.834948825496938163, -5.907420853759296264, -7.720982897393569466 ) ) ;
#157240=CARTESIAN_POINT ( 'NONE',  ( 10.91970695577495754, -6.134628647623513231, 1.924458856161770370E-15 ) ) ;
#157254=CIRCLE ( 'NONE', #5053, 6.249999999999995559 ) ;
#157260=VERTEX_POINT ( 'NONE', #164694 ) ;
#157312=ORIENTED_EDGE ( 'NONE', *, *, #6621, .T. ) ;
#157325=CARTESIAN_POINT ( 'NONE',  ( 0.000000000000000000, 1.000000000000000888, 0.000000000000000000 ) ) ;
#157333=VERTEX_POINT ( 'NONE', #87702 ) ;
#157335=AXIS2_PLACEMENT_3D ( 'NONE', #192695, #173287, #205754 ) ;
#157383=( BOUNDED_SURFACE ( )  B_SPLINE_SURFACE ( 3, 2, ( 
 ( #194863, #109428, #25957 ),
 ( #178630, #9711, #190585 ),
 ( #30242, #93127, #58472 ),
 ( #110490, #124627, #75787 ),
 ( #207905, #60594, #126752 ),
 ( #59526, #44367, #176489 ),
 ( #28100, #87254, #4893 ),
 ( #3829, #214264, #185797 ) ),
 .UNSPECIFIED., .F., .F., .T. ) 
 B_SPLINE_SURFACE_WITH_KNOTS ( ( 4, 2, 2, 4 ),
 ( 3, 3 ),
 ( -2.710505431213761085E-20, 0.0002475938981900015407, 0.0004951877963800030815, 0.0009903755927600061629 ),
 ( 0.000000000000000000, 1.000000000000000000 ),
 .UNSPECIFIED. ) 
 GEOMETRIC_REPRESENTATION_ITEM ( )  RATIONAL_B_SPLINE_SURFACE ( (
 ( 1.000000000000000000, 0.9238795325112871826, 1.000000000000000000),
 ( 1.000000000000000000, 0.9248499699754035852, 1.000000000000000000),
 ( 1.000000000000000000, 0.9171047238582761274, 1.000000000000000000),
 ( 1.000000000000000000, 0.8907236462370136110, 1.000000000000000000),
 ( 1.000000000000000000, 0.8725411758594030509, 1.000000000000000000),
 ( 1.000000000000000000, 0.8105159241144254123, 1.000000000000000000),
 ( 1.000000000000000000, 0.7599483315139430317, 1.000000000000000000),
 ( 1.000000000000000000, 0.7045118851637766078, 1.000000000000000000) ) ) 
 REPRESENTATION_ITEM ( '' )  SURFACE ( )  );
#157384=VECTOR ( 'NONE', #16358, 1000.000000000000000 ) ;
#157400=AXIS2_PLACEMENT_3D ( 'NONE', #41285, #6599, #39129 ) ;
#157451=CARTESIAN_POINT ( 'NONE',  ( -1.296982317953438165E-13, -8.296536394940860148, -10.41260094161052230 ) ) ;
#157458=EDGE_LOOP ( 'NONE', ( #20743, #53762, #19185 ) ) ;
#157486=CARTESIAN_POINT ( 'NONE',  ( 6.949550370340926264, -6.532648880269158909, -6.447678837262559526 ) ) ;
#157488=AXIS2_PLACEMENT_3D ( 'NONE', #200521, #171237, #119360 ) ;
#157499=CARTESIAN_POINT ( 'NONE',  ( 0.000000000000000000, -9.006862915010128035, 0.000000000000000000 ) ) ;
#157564=CARTESIAN_POINT ( 'NONE',  ( -2.554955805669734570, 1.016282880930316823, 12.02012201174058426 ) ) ;
#157630=VERTEX_POINT ( 'NONE', #123503 ) ;
#157668=AXIS2_PLACEMENT_3D ( 'NONE', #84878, #202870, #150966 ) ;
#157670=DIRECTION ( 'NONE',  ( -0.000000000000000000, -1.000000000000000000, -0.000000000000000000 ) ) ;
#157678=EDGE_CURVE ( 'NONE', #148901, #62943, #136146, .T. ) ;
#157682=CARTESIAN_POINT ( 'NONE',  ( -0.08058608058609216529, -8.407420853759283830, -10.99970480893080271 ) ) ;
#157694=CARTESIAN_POINT ( 'NONE',  ( 0.1376292675369541196, -5.401429653175749301, 10.96107445065239183 ) ) ;
#157701=( NAMED_UNIT ( * ) PLANE_ANGLE_UNIT ( ) SI_UNIT ( $, .RADIAN. ) );
#157711=VERTEX_POINT ( 'NONE', #188393 ) ;
#157721=SURFACE_STYLE_USAGE ( .BOTH. , #204280 ) ;
#157755=ORIENTED_EDGE ( 'NONE', *, *, #124443, .F. ) ;
#157797=CARTESIAN_POINT ( 'NONE',  ( 0.000000000000000000, 3.447199233515649386, 12.00000000000000178 ) ) ;
#157841=CARTESIAN_POINT ( 'NONE',  ( 7.047292192040121250, -5.787795860784306079, 7.664865541495959889 ) ) ;
#157857=AXIS2_PLACEMENT_3D ( 'NONE', #32759, #53275, #20747 ) ;
#157882=CARTESIAN_POINT ( 'NONE',  ( 7.873959529867758711, -5.295524846228442328, -7.681496476274664253 ) ) ;
#157898=EDGE_LOOP ( 'NONE', ( #84338, #183248, #137379 ) ) ;
#157907=CARTESIAN_POINT ( 'NONE',  ( -10.91970695577495931, -6.134628647623513231, 0.000000000000000000 ) ) ;
#157912=CARTESIAN_POINT ( 'NONE',  ( -9.183873789516530550, -7.868711957285995595, 1.138412281109779656E-15 ) ) ;
#157919=CARTESIAN_POINT ( 'NONE',  ( -6.949925879317538246, -6.532648833121172061, 6.447267651612382799 ) ) ;
#157921=CARTESIAN_POINT ( 'NONE',  ( 7.654042494670951690E-16, -13.99999999999999822, -6.249999999999995559 ) ) ;
#157926=EDGE_CURVE ( 'NONE', #401, #149119, #127831, .T. ) ;
#157940=SURFACE_SIDE_STYLE ('',( #158991 ) ) ;
#157943=CARTESIAN_POINT ( 'NONE',  ( -0.3610206255356728233, -7.699789852011537761, 10.99434576732824631 ) ) ;
#157946=CIRCLE ( 'NONE', #182178, 11.89429233241351902 ) ;
#157968=CIRCLE ( 'NONE', #78474, 6.277139874739035008 ) ;
#157972=( BOUNDED_SURFACE ( )  B_SPLINE_SURFACE ( 3, 2, ( 
 ( #2666, #131687, #197689 ),
 ( #17854, #200868, #52512 ),
 ( #36247, #115453, #205140 ),
 ( #203006, #138046, #74106 ),
 ( #57847, #120794, #186771 ),
 ( #107741, #140199, #124008 ),
 ( #23186, #38398, #156429 ),
 ( #206220, #54646, #189975 ) ),
 .UNSPECIFIED., .F., .F., .T. ) 
 B_SPLINE_SURFACE_WITH_KNOTS ( ( 4, 2, 2, 4 ),
 ( 3, 3 ),
 ( 0.000000000000000000, 0.0002204160392919288941, 0.0004408320785838577881, 0.0008816641571677155762 ),
 ( 0.000000000000000000, 1.000000000000000000 ),
 .UNSPECIFIED. ) 
 GEOMETRIC_REPRESENTATION_ITEM ( )  RATIONAL_B_SPLINE_SURFACE ( (
 ( 1.000000000000000000, 0.4127341956165084258, 1.000000000000000000),
 ( 1.000000000000000000, 0.4103180386332804241, 1.000000000000000000),
 ( 1.000000000000000000, 0.4223234233956687511, 1.000000000000000000),
 ( 1.000000000000000000, 0.4613847219400475375, 1.000000000000000000),
 ( 1.000000000000000000, 0.4878744032656874285, 1.000000000000000000),
 ( 1.000000000000000000, 0.5702658980232629959, 1.000000000000000000),
 ( 1.000000000000000000, 0.6280001242511515924, 1.000000000000000000),
 ( 1.000000000000000000, 0.6787756258918324903, 1.000000000000000000) ) ) 
 REPRESENTATION_ITEM ( '' )  SURFACE ( )  );
#157985=CARTESIAN_POINT ( 'NONE',  ( 7.462104991928526054, -5.166862915010159263, 8.081892667527535323 ) ) ;
#158088=AXIS2_PLACEMENT_3D ( 'NONE', #206563, #87754, #127555 ) ;
#158114=DIRECTION ( 'NONE',  ( 0.5000000000000041078, 0.000000000000000000, 0.8660254037844363761 ) ) ;
#158118=AXIS2_PLACEMENT_3D ( 'NONE', #130927, #99435, #197979 ) ;
#158120=CARTESIAN_POINT ( 'NONE',  ( -8.832353407160665526, 3.956598013261175772, -7.432338980325321920 ) ) ;
#158178=FACE_OUTER_BOUND ( 'NONE', #118922, .T. ) ;
#158192=CARTESIAN_POINT ( 'NONE',  ( 1.270994156678442596E-16, -6.530144695498194096, -11.00000000000000178 ) ) ;
#158227=CARTESIAN_POINT ( 'NONE',  ( 7.626074735689158501, -6.442483420751605294, 8.280982046698079913 ) ) ;
#158228=ORIENTED_EDGE ( 'NONE', *, *, #73977, .T. ) ;
#158236=CARTESIAN_POINT ( 'NONE',  ( -9.499771961674738918, -7.051679281653864706, -0.06642998979260299197 ) ) ;
#158238=EDGE_CURVE ( 'NONE', #86477, #114840, #164531, .T. ) ;
#158239=CARTESIAN_POINT ( 'NONE',  ( 0.07602376731354228145, -7.154544010627095219, -9.579698345292676720 ) ) ;
#158267=ORIENTED_EDGE ( 'NONE', *, *, #83921, .T. ) ;
#158271=DIRECTION ( 'NONE',  ( 0.000000000000000000, 0.000000000000000000, -1.000000000000000000 ) ) ;
#158272=CARTESIAN_POINT ( 'NONE',  ( -10.99931799034184365, -8.075210796978268490, 0.1485693272542949472 ) ) ;
#158308=CARTESIAN_POINT ( 'NONE',  ( 1.342212891865499298E-15, -2.000000000000001776, -10.92000000000000171 ) ) ;
#158314=DIRECTION ( 'NONE',  ( 8.881784197001252323E-16, 0.000000000000000000, 1.000000000000000000 ) ) ;
#158337=ORIENTED_EDGE ( 'NONE', *, *, #148852, .T. ) ;
#158444=SURFACE_STYLE_USAGE ( .BOTH. , #23076 ) ;
#158480=ADVANCED_FACE ( 'NONE', ( #181724 ), #68366, .F. ) ;
#158483=( NAMED_UNIT ( * ) SI_UNIT ( $, .STERADIAN. ) SOLID_ANGLE_UNIT ( ) );
#158511=VECTOR ( 'NONE', #4569, 1000.000000000000227 ) ;
#158520=CARTESIAN_POINT ( 'NONE',  ( -10.33293948230774184, 2.515145635913770494, 5.518992160705051830 ) ) ;
#158522=ORIENTED_EDGE ( 'NONE', *, *, #162808, .F. ) ;
#158543=B_SPLINE_CURVE_WITH_KNOTS ( 'NONE', 3,
 ( #146286, #125827, #79114, #9849, #113828, #75924, #76977, #94334 ),
 .UNSPECIFIED., .F., .F.,
 ( 4, 2, 2, 4 ),
 ( 0.000000000000000000, 0.0005156231957999833160, 0.0007734347936999757872, 0.001031246391599968367 ),
 .UNSPECIFIED. ) ;
#158552=AXIS2_PLACEMENT_3D ( 'NONE', #83424, #183060, #68223 ) ;
#158559=DIRECTION ( 'NONE',  ( 0.000000000000000000, 1.000000000000000000, 0.000000000000000000 ) ) ;
#158562=CARTESIAN_POINT ( 'NONE',  ( 6.849482339516208995, -6.938199013094656920, -6.234224025626343924 ) ) ;
#158609=EDGE_CURVE ( 'NONE', #45686, #133392, #10208, .T. ) ;
#158643=EDGE_LOOP ( 'NONE', ( #152104, #43345, #173715, #118963 ) ) ;
#158688=ORIENTED_EDGE ( 'NONE', *, *, #35615, .F. ) ;
#158704=DIRECTION ( 'NONE',  ( -1.000000000000000000, 0.000000000000000000, 0.000000000000000000 ) ) ;
#158729=EDGE_CURVE ( 'NONE', #201530, #6442, #41333, .T. ) ;
#158732=EDGE_CURVE ( 'NONE', #32900, #57699, #179689, .T. ) ;
#158747=CARTESIAN_POINT ( 'NONE',  ( 0.4373225248172846746, -5.223431457505083308, 10.96785329849814694 ) ) ;
#158775=FILL_AREA_STYLE_COLOUR ( '', #81182 ) ;
#158799=FACE_OUTER_BOUND ( 'NONE', #82706, .T. ) ;
#158807=CARTESIAN_POINT ( 'NONE',  ( 9.623628927379545672, -9.094708467121352058, -0.4567741993462098860 ) ) ;
#158813=CARTESIAN_POINT ( 'NONE',  ( -9.512045263456270661, -8.176568542494905500, 0.4655551865852137206 ) ) ;
#158814=CARTESIAN_POINT ( 'NONE',  ( 9.499386779316314033, -9.999529051968279347, -0.1207253440361106545 ) ) ;
#158855=VECTOR ( 'NONE', #50968, 1000.000000000000000 ) ;
#158865=EDGE_CURVE ( 'NONE', #214101, #194102, #110057, .T. ) ;
#158953=CARTESIAN_POINT ( 'NONE',  ( 10.91828647086817661, -9.953005061877725268, -0.1753736836078278460 ) ) ;
#158973=CARTESIAN_POINT ( 'NONE',  ( 0.07933194154487524519, -9.900000000000005684, 9.499668754385634628 ) ) ;
#158991=SURFACE_STYLE_FILL_AREA ( #172045 ) ;
#158998=ADVANCED_FACE ( 'NONE', ( #115386 ), #55068, .T. ) ;
#159016=VERTEX_POINT ( 'NONE', #117513 ) ;
#159026=DIRECTION ( 'NONE',  ( 0.000000000000000000, 0.000000000000000000, -1.000000000000000000 ) ) ;
#159031=SURFACE_SIDE_STYLE ('',( #94053 ) ) ;
#159059=CARTESIAN_POINT ( 'NONE',  ( 0.1329251406260184842, -9.135512438678594194, -9.499304248211862145 ) ) ;
#159078=CARTESIAN_POINT ( 'NONE',  ( -6.764644832401259578, -7.632775601084016870, 6.764644832398700736 ) ) ;
#159125=CARTESIAN_POINT ( 'NONE',  ( -10.79929312474869008, -8.526088927970988607, 0.1885023626713056288 ) ) ;
#159145=STYLED_ITEM ( 'NONE', ( #117404 ), #112039 ) ;
#159156=CARTESIAN_POINT ( 'NONE',  ( -0.003376046620573100454, -7.161464053357560644, -9.586610838029425707 ) ) ;
#159158=CARTESIAN_POINT ( 'NONE',  ( 0.000000000000000000, -1.000000000000000888, 0.000000000000000000 ) ) ;
#159192=CARTESIAN_POINT ( 'NONE',  ( 0.09463244300324949454, -8.038540703696430256, 9.499633399276474321 ) ) ;
#159217=( BOUNDED_SURFACE ( )  B_SPLINE_SURFACE ( 3, 2, ( 
 ( #183887, #104801, #86399 ),
 ( #170846, #169775, #5108 ),
 ( #37646, #201185, #54970 ),
 ( #118961, #151408, #121122 ) ),
 .UNSPECIFIED., .F., .F., .T. ) 
 B_SPLINE_SURFACE_WITH_KNOTS ( ( 4, 4 ),
 ( 3, 3 ),
 ( -1.355252715606880543E-20, 3.124373798652707124E-05 ),
 ( 0.000000000000000000, 1.000000000000000000 ),
 .UNSPECIFIED. ) 
 GEOMETRIC_REPRESENTATION_ITEM ( )  RATIONAL_B_SPLINE_SURFACE ( (
 ( 1.000000000000000000, 0.7071067811870692665, 1.000000000000000000),
 ( 1.000000000000000000, 0.7053575014263949727, 1.000000000000000000),
 ( 1.000000000000000000, 0.7044883013754549284, 1.000000000000000000),
 ( 1.000000000000000000, 0.7045118851643193958, 1.000000000000000000) ) ) 
 REPRESENTATION_ITEM ( '' )  SURFACE ( )  );
#159239=ADVANCED_FACE ( 'NONE', ( #165134 ), #46272, .F. ) ;
#159240=CARTESIAN_POINT ( 'NONE',  ( -9.797921721691023933, 3.956598013261175772, -6.103348209225892163 ) ) ;
#159269=CARTESIAN_POINT ( 'NONE',  ( -8.787802685836078709, 3.956598013261175772, -7.485281629513451662 ) ) ;
#159271=CARTESIAN_POINT ( 'NONE',  ( -9.855659161987910366, -6.334709917115479705, 0.4359479416626658166 ) ) ;
#159303=CARTESIAN_POINT ( 'NONE',  ( 0.09999999999999592548, -9.999999999999994671, 9.579478065113978147 ) ) ;
#159304=CARTESIAN_POINT ( 'NONE',  ( 6.984891963203275544, -8.199734048663231079, -6.439526774796777708 ) ) ;
#159306=ORIENTED_EDGE ( 'NONE', *, *, #208716, .F. ) ;
#159320=ORIENTED_EDGE ( 'NONE', *, *, #44682, .F. ) ;
#159328=CARTESIAN_POINT ( 'NONE',  ( 0.000000000000000000, -1.000000000000000888, 10.24999999999998934 ) ) ;
#159341=B_SPLINE_CURVE_WITH_KNOTS ( 'NONE', 3,
 ( #42610, #121786, #89220, #156348, #108719, #7932, #205061, #24175, #142251, #208263, #192011, #43674, #40466, #64176, #78275, #176854 ),
 .UNSPECIFIED., .F., .F.,
 ( 4, 3, 3, 3, 3, 4 ),
 ( 0.000000000000000000, 2.209015272824978271E-05, 5.594181769345698359E-05, 8.979300607464787737E-05, 0.0001236442050441801050, 0.0001574956163004470730 ),
 .UNSPECIFIED. ) ;
#159349=CARTESIAN_POINT ( 'NONE',  ( 0.03870269234684881043, -9.454881121928412568, -9.603712783164930045 ) ) ;
#159350=CARTESIAN_POINT ( 'NONE',  ( -7.719547554928817945, -5.360178282914185743, -7.836475020641948674 ) ) ;
#159358=DIRECTION ( 'NONE',  ( 0.000000000000000000, 0.000000000000000000, 1.000000000000000000 ) ) ;
#159375=ORIENTED_EDGE ( 'NONE', *, *, #63361, .T. ) ;
#159380=CARTESIAN_POINT ( 'NONE',  ( -7.808923410443597390, -5.575271019048065213, -7.747753938335034007 ) ) ;
#159383=ORIENTED_EDGE ( 'NONE', *, *, #197793, .T. ) ;
#159411=EDGE_LOOP ( 'NONE', ( #146620, #60293, #62055, #152751 ) ) ;
#159427=EDGE_CURVE ( 'NONE', #1801, #113056, #62178, .T. ) ;
#159434=ADVANCED_FACE ( 'NONE', ( #143642 ), #13584, .F. ) ;
#159448=UNCERTAINTY_MEASURE_WITH_UNIT (LENGTH_MEASURE( 1.000000000000000082E-05 ), #213381, 'distance_accuracy_value', 'NONE');
#159480=VERTEX_POINT ( 'NONE', #127438 ) ;
#159573=EDGE_LOOP ( 'NONE', ( #39441, #180049, #91988, #164757 ) ) ;
#159574=AXIS2_PLACEMENT_3D ( 'NONE', #138821, #35964, #169169 ) ;
#159583=VERTEX_POINT ( 'NONE', #47189 ) ;
#159594=CARTESIAN_POINT ( 'NONE',  ( -10.91944002402978775, -9.999999999999994671, 0.1905873483556694281 ) ) ;
#159634=CARTESIAN_POINT ( 'NONE',  ( 0.09630943990283219458, -9.919512026728389387, 10.99957837791002468 ) ) ;
#159645=EDGE_CURVE ( 'NONE', #96467, #149119, #51827, .T. ) ;
#159818=ORIENTED_EDGE ( 'NONE', *, *, #17272, .F. ) ;
#159838=DIRECTION ( 'NONE',  ( 0.01745240643728004568, 0.000000000000000000, 0.9998476951563913806 ) ) ;
#159862=CARTESIAN_POINT ( 'NONE',  ( -0.4265819271709386240, -6.701306620466009889, -10.99180900346563661 ) ) ;
#159935=CARTESIAN_POINT ( 'NONE',  ( 0.05648045292896410746, -9.990726591626527764, 10.91961852020055979 ) ) ;
#159936=ORIENTED_EDGE ( 'NONE', *, *, #54326, .T. ) ;
#159960=CARTESIAN_POINT ( 'NONE',  ( -0.07933194154558138866, -7.215597533182092960, 9.499668754385638181 ) ) ;
#159987=CARTESIAN_POINT ( 'NONE',  ( 10.98194350564910415, -7.666862915010147717, -0.6300133639306100264 ) ) ;
#160000=DIRECTION ( 'NONE',  ( 0.000000000000000000, 1.000000000000000000, 0.000000000000000000 ) ) ;
#160078=EDGE_CURVE ( 'NONE', #35104, #71781, #130126, .T. ) ;
#160094=CARTESIAN_POINT ( 'NONE',  ( 7.834948825496931057, -5.823938088759704534, 7.720982897393584565 ) ) ;
#160146=CARTESIAN_POINT ( 'NONE',  ( -6.958662999125652782, -8.148356111791692058, 6.505896022970778958 ) ) ;
#160162=CARTESIAN_POINT ( 'NONE',  ( 0.3656762941044484627, -7.723177556210781169, -10.97096416026298904 ) ) ;
#160212=DIRECTION ( 'NONE',  ( 0.000000000000000000, -1.000000000000000000, 0.000000000000000000 ) ) ;
#160213=CYLINDRICAL_SURFACE ( 'NONE', #4030, 0.08000000000000020983 ) ;
#160219=VERTEX_POINT ( 'NONE', #109333 ) ;
#160225=( NAMED_UNIT ( * ) PLANE_ANGLE_UNIT ( ) SI_UNIT ( $, .RADIAN. ) );
#160236=ORIENTED_EDGE ( 'NONE', *, *, #3792, .F. ) ;
#160304=VECTOR ( 'NONE', #182026, 1000.000000000000227 ) ;
#160339=ADVANCED_FACE ( 'NONE', ( #176398 ), #76740, .T. ) ;
#160368=B_SPLINE_CURVE_WITH_KNOTS ( 'NONE', 3,
 ( #160791, #133381, #184211, #167977, #51032, #197267, #144582, #49963 ),
 .UNSPECIFIED., .F., .F.,
 ( 4, 2, 2, 4 ),
 ( 6.599180864910166611E-16, 0.0002305131806121978120, 0.0004610263612237356702, 0.0009220527224468131212 ),
 .UNSPECIFIED. ) ;
#160376=CARTESIAN_POINT ( 'NONE',  ( 7.565242077046510971, -6.863172033216027756, 7.985752187169479654 ) ) ;
#160377=CARTESIAN_POINT ( 'NONE',  ( -7.487360338304412721, -6.465328379374280843, -7.487360338304378971 ) ) ;
#160381=CIRCLE ( 'NONE', #139678, 0.08000000000000001554 ) ;
#160398=( NAMED_UNIT ( * ) SI_UNIT ( $, .STERADIAN. ) SOLID_ANGLE_UNIT ( ) );
#160413=ORIENTED_EDGE ( 'NONE', *, *, #165205, .T. ) ;
#160442=AXIS2_PLACEMENT_3D ( 'NONE', #153407, #119906, #52696 ) ;
#160452=VERTEX_POINT ( 'NONE', #96226 ) ;
#160482=CARTESIAN_POINT ( 'NONE',  ( 6.506163559800162588, -8.203199116536543656, 6.922777049148927553 ) ) ;
#160496=ORIENTED_EDGE ( 'NONE', *, *, #64003, .F. ) ;
#160504=CARTESIAN_POINT ( 'NONE',  ( -9.499700864329909678, -7.154544010627095219, -0.07538891330675229208 ) ) ;
#160566=CARTESIAN_POINT ( 'NONE',  ( 6.758184431511291557, -6.900108348305955985, 6.825879202496260234 ) ) ;
#160574=CARTESIAN_POINT ( 'NONE',  ( 7.720982897393566802, -5.907420853759296264, -7.834948825496929281 ) ) ;
#160575=CARTESIAN_POINT ( 'NONE',  ( -8.002408263930261612, -6.836568542494980250, 7.346809171966449448 ) ) ;
#160577=( NAMED_UNIT ( * ) PLANE_ANGLE_UNIT ( ) SI_UNIT ( $, .RADIAN. ) );
#160601=DIRECTION ( 'NONE',  ( 0.000000000000000000, 0.000000000000000000, 1.000000000000000000 ) ) ;
#160605=CIRCLE ( 'NONE', #94908, 11.49999999999998934 ) ;
#160629=DIRECTION ( 'NONE',  ( 0.000000000000000000, 0.000000000000000000, 1.000000000000000000 ) ) ;
#160637=EDGE_CURVE ( 'NONE', #119366, #12329, #169462, .T. ) ;
#160676=CARTESIAN_POINT ( 'NONE',  ( -9.597801448743025432, -7.025535116234744137, 0.01424860406304543671 ) ) ;
#160742=CIRCLE ( 'NONE', #5003, 10.99999999999999112 ) ;
#160791=CARTESIAN_POINT ( 'NONE',  ( -7.346809171966454777, -6.836568542494980250, -8.002408263930250953 ) ) ;
#160832=PRESENTATION_STYLE_ASSIGNMENT (( #62261 ) ) ;
#160866=ADVANCED_FACE ( 'NONE', ( #26411 ), #76612, .F. ) ;
#160878=CARTESIAN_POINT ( 'NONE',  ( 10.10343170206398966, 2.974000657017692006, -5.833219012919978574 ) ) ;
#160908=CIRCLE ( 'NONE', #84681, 0.07999999999999990452 ) ;
#160923=ORIENTED_EDGE ( 'NONE', *, *, #159645, .F. ) ;
#160977=CARTESIAN_POINT ( 'NONE',  ( -7.725699985795401403, -5.832912386296871254, 7.725699985795430713 ) ) ;
#160981=CARTESIAN_POINT ( 'NONE',  ( -8.081892667527538876, -5.166862915010145052, 7.462104991928527831 ) ) ;
#161010=CARTESIAN_POINT ( 'NONE',  ( -6.493979434129342643, -7.868711957284892478, -6.493979434129312445 ) ) ;
#161057=EDGE_CURVE ( 'NONE', #210172, #118273, #42951, .T. ) ;
#161058=CIRCLE ( 'NONE', #95370, 0.07999999999999993228 ) ;
#161063=AXIS2_PLACEMENT_3D ( 'NONE', #175339, #8544, #73547 ) ;
#161091=DIRECTION ( 'NONE',  ( -0.5254827454987585078, 0.7071067811865536790, -0.4731467892558060551 ) ) ;
#161126=DIRECTION ( 'NONE',  ( 0.000000000000000000, 1.000000000000000000, 0.000000000000000000 ) ) ;
#161190=ORIENTED_EDGE ( 'NONE', *, *, #142193, .T. ) ;
#161193=CARTESIAN_POINT ( 'NONE',  ( 10.99976498415366954, -5.359187537802506895, -0.08336379702153423610 ) ) ;
#161244=CARTESIAN_POINT ( 'NONE',  ( 10.12536109763334125, -7.563986176625362212, -0.4645846211130729708 ) ) ;
#161266=DIRECTION ( 'NONE',  ( 1.000000000000000000, 0.000000000000000000, 0.000000000000000000 ) ) ;
#161322=CARTESIAN_POINT ( 'NONE',  ( 2.032879073410320814E-16, -7.630846356335640124, -9.566809970447321732 ) ) ;
#161334=DIRECTION ( 'NONE',  ( 0.9999580691339164940, 0.000000000000000000, -0.009157509157509348754 ) ) ;
#161397=CARTESIAN_POINT ( 'NONE',  ( 6.776370306708061619, -7.161464053357560644, 6.781144757626056396 ) ) ;
#161458=CARTESIAN_POINT ( 'NONE',  ( -7.253312916980337199, -6.796015482748900105, -7.253312916980295455 ) ) ;
#161460=ORIENTED_EDGE ( 'NONE', *, *, #14059, .T. ) ;
#161465=EDGE_LOOP ( 'NONE', ( #52215, #76987, #128520, #49289, #25878 ) ) ;
#161473=ORIENTED_EDGE ( 'NONE', *, *, #162808, .T. ) ;
#161495=ORIENTED_EDGE ( 'NONE', *, *, #17156, .T. ) ;
#161532=CARTESIAN_POINT ( 'NONE',  ( -7.524604700374180055, -5.166862990899345753, -8.024185963717888725 ) ) ;
#161536=ORIENTED_EDGE ( 'NONE', *, *, #31789, .T. ) ;
#161563=EDGE_LOOP ( 'NONE', ( #99870, #102102, #19502, #153193 ) ) ;
#161600=EDGE_LOOP ( 'NONE', ( #99205, #6592, #9476, #82280 ) ) ;
#161602=UNCERTAINTY_MEASURE_WITH_UNIT (LENGTH_MEASURE( 1.000000000000000082E-05 ), #201277, 'distance_accuracy_value', 'NONE');
#161645=LINE ( 'NONE', #108675, #19745 ) ;
#161685=PRESENTATION_STYLE_ASSIGNMENT (( #130317 ) ) ;
#161695=EDGE_CURVE ( 'NONE', #135683, #42950, #131685, .T. ) ;
#161721=CYLINDRICAL_SURFACE ( 'NONE', #69963, 0.07999999999999993228 ) ;
#161735=VERTEX_POINT ( 'NONE', #523 ) ;
#161755=ORIENTED_EDGE ( 'NONE', *, *, #200438, .F. ) ;
#161757=CARTESIAN_POINT ( 'NONE',  ( -9.605899910213580029, -6.890735599539922873, 0.05097232478521593335 ) ) ;
#161868=AXIS2_PLACEMENT_3D ( 'NONE', #172000, #24658, #126529 ) ;
#161977=EDGE_LOOP ( 'NONE', ( #95316, #16847, #110882, #59527, #188500, #202593 ) ) ;
#161985=CARTESIAN_POINT ( 'NONE',  ( -1.734723475976807094E-15, -9.900000000000005684, -10.91970695577494332 ) ) ;
#161999=CARTESIAN_POINT ( 'NONE',  ( -2.020417662918760016, 3.956598013261175772, 11.36521191596583336 ) ) ;
#162056=AXIS2_PLACEMENT_3D ( 'NONE', #166437, #84115, #162190 ) ;
#162069=CIRCLE ( 'NONE', #44573, 0.08000000000000025147 ) ;
#162086=FACE_OUTER_BOUND ( 'NONE', #211310, .T. ) ;
#162130=CARTESIAN_POINT ( 'NONE',  ( -0.4350533259329449343, -9.438199013093624856, 9.251577493846887990 ) ) ;
#162134=AXIS2_PLACEMENT_3D ( 'NONE', #124572, #10715, #141845 ) ;
#162142=VERTEX_POINT ( 'NONE', #77298 ) ;
#162145=DIRECTION ( 'NONE',  ( 1.084202172485362439E-14, -1.000000000000000000, 3.260636891504970529E-14 ) ) ;
#162155=DIRECTION ( 'NONE',  ( -7.610300982150707428E-15, -1.000000000000000000, 7.722633184682877167E-15 ) ) ;
#162170=CARTESIAN_POINT ( 'NONE',  ( -11.21553972792701259, 3.696394713403124754, 3.679259263401783553 ) ) ;
#162172=CARTESIAN_POINT ( 'NONE',  ( -9.501690547401159037, -8.186910008819943130, 0.4655726814551116033 ) ) ;
#162190=DIRECTION ( 'NONE',  ( 0.000000000000000000, 0.000000000000000000, 1.000000000000000000 ) ) ;
#162218=CIRCLE ( 'NONE', #75777, 0.07999999999999993228 ) ;
#162257=CARTESIAN_POINT ( 'NONE',  ( 9.492545994385622521, -8.199730735665681891, -0.3846410972799483852 ) ) ;
#162261=ADVANCED_FACE ( 'NONE', ( #93575 ), #48571, .T. ) ;
#162281=CARTESIAN_POINT ( 'NONE',  ( 8.103009739377979415, -6.893137084989842123, -7.439168848974011539 ) ) ;
#162283=EDGE_LOOP ( 'NONE', ( #121466, #96917, #73998, #134568, #153751 ) ) ;
#162301=CARTESIAN_POINT ( 'NONE',  ( 0.08202876420372311184, -7.861065518611666469, -10.99977341864973468 ) ) ;
#162318=CARTESIAN_POINT ( 'NONE',  ( 2.373851744317274193, 1.000000000000000888, -11.76285798163019969 ) ) ;
#162349=( GEOMETRIC_REPRESENTATION_CONTEXT ( 3 ) GLOBAL_UNCERTAINTY_ASSIGNED_CONTEXT ( ( #49407 ) ) GLOBAL_UNIT_ASSIGNED_CONTEXT ( ( #31107, #49471, #63588 ) ) REPRESENTATION_CONTEXT ( 'NONE', 'WORKASPACE' ) );
#162405=LINE ( 'NONE', #29197, #196337 ) ;
#162410=CARTESIAN_POINT ( 'NONE',  ( 0.3773006915670404915, -8.233136995002887204, 9.492905263954449779 ) ) ;
#162490=ORIENTED_EDGE ( 'NONE', *, *, #118098, .T. ) ;
#162537=COLOUR_RGB ( '', 0.40784314, 0.44705882, 0.49803922) ;
#162539=EDGE_CURVE ( 'NONE', #322, #50087, #138557, .T. ) ;
#162544=DIRECTION ( 'NONE',  ( 0.000000000000000000, 0.000000000000000000, 1.000000000000000000 ) ) ;
#162586=( NAMED_UNIT ( * ) PLANE_ANGLE_UNIT ( ) SI_UNIT ( $, .RADIAN. ) );
#162596=ORIENTED_EDGE ( 'NONE', *, *, #107493, .F. ) ;
#162597=CARTESIAN_POINT ( 'NONE',  ( 0.04277205541326366267, -9.414847940711716490, 9.500256024741366545 ) ) ;
#162624=CARTESIAN_POINT ( 'NONE',  ( 6.773376336902542150, -7.645781813054120413, 6.661184053806703531 ) ) ;
#162653=LINE ( 'NONE', #80319, #31197 ) ;
#162663=CARTESIAN_POINT ( 'NONE',  ( -6.781144757626061725, -7.161464053357567749, 6.776370306708065172 ) ) ;
#162664=CARTESIAN_POINT ( 'NONE',  ( -9.000007961041697868, 1.000000000000000888, -7.937244906211844864 ) ) ;
#162665=EDGE_LOOP ( 'NONE', ( #173602, #205459, #34352, #117167 ) ) ;
#162720=CARTESIAN_POINT ( 'NONE',  ( -1.938011383317839176E-15, -9.900000000000005684, -10.91970695577503214 ) ) ;
#162723=B_SPLINE_CURVE_WITH_KNOTS ( 'NONE', 3,
 ( #22784, #6540, #137650, #121470 ),
 .UNSPECIFIED., .F., .F.,
 ( 4, 4 ),
 ( 0.000000000000000000, 6.033646489354581229E-05 ),
 .UNSPECIFIED. ) ;
#162728=FACE_OUTER_BOUND ( 'NONE', #80142, .T. ) ;
#162735=CARTESIAN_POINT ( 'NONE',  ( 7.564733433744389224, -6.863455982311506887, 7.986233326679982092 ) ) ;
#162779=CARTESIAN_POINT ( 'NONE',  ( -6.716119544743476943, -7.217450603038121137, -6.719405205105408285 ) ) ;
#162787=DIRECTION ( 'NONE',  ( 0.000000000000000000, 0.000000000000000000, 1.000000000000000000 ) ) ;
#162790=CARTESIAN_POINT ( 'NONE',  ( 7.777446446097294519, -5.502990254781792601, -7.779015489124648575 ) ) ;
#162808=EDGE_CURVE ( 'NONE', #129260, #76748, #176973, .T. ) ;
#162811=VERTEX_POINT ( 'NONE', #24569 ) ;
#162824=ORIENTED_EDGE ( 'NONE', *, *, #12707, .F. ) ;
#162827=CARTESIAN_POINT ( 'NONE',  ( 0.08118383494905327680, -9.908729948657658326, 9.499653137018322369 ) ) ;
#162856=EDGE_CURVE ( 'NONE', #41100, #130351, #86755, .T. ) ;
#162861=CARTESIAN_POINT ( 'NONE',  ( -7.725699985795428049, -5.832912386296868590, -7.725699985795385416 ) ) ;
#162868=CARTESIAN_POINT ( 'NONE',  ( 7.221001870987139526, -6.414086731524418994, -6.604641253243922705 ) ) ;
#162880=TOROIDAL_SURFACE ( 'NONE', #69453, 6.330000000000000959, 0.08000000000000000167 ) ;
#162917=ORIENTED_EDGE ( 'NONE', *, *, #119057, .F. ) ;
#162980=CARTESIAN_POINT ( 'NONE',  ( 1.342212891865499298E-15, -1.000000000000000888, 10.92000000000000171 ) ) ;
#163017=CARTESIAN_POINT ( 'NONE',  ( 10.28586320583508495, 2.972657967447012162, -5.491880110201817544 ) ) ;
#163036=CIRCLE ( 'NONE', #48931, 0.07999999999999993228 ) ;
#163062=( BOUNDED_SURFACE ( )  B_SPLINE_SURFACE ( 3, 2, ( 
 ( #162720, #124160, #130287 ),
 ( #195209, #147533, #14292 ),
 ( #47922, #146483, #107889 ),
 ( #31649, #25491, #191178 ) ),
 .UNSPECIFIED., .F., .F., .F. ) 
 B_SPLINE_SURFACE_WITH_KNOTS ( ( 4, 4 ),
 ( 3, 3 ),
 ( 0.000000000000000000, 3.124373657233978183E-05 ),
 ( 0.000000000000000000, 1.000000000000000000 ),
 .UNSPECIFIED. ) 
 GEOMETRIC_REPRESENTATION_ITEM ( )  RATIONAL_B_SPLINE_SURFACE ( (
 ( 1.000000000000000000, 0.7045118851641303248, 1.000000000000000000),
 ( 1.000000000000000000, 0.7044892147945189809, 1.000000000000000000),
 ( 1.000000000000000000, 0.7053501046726613488, 1.000000000000000000),
 ( 1.000000000000000000, 0.7071067811869121700, 1.000000000000000000) ) ) 
 REPRESENTATION_ITEM ( '' )  SURFACE ( )  );
#163075=ORIENTED_EDGE ( 'NONE', *, *, #181317, .F. ) ;
#163082=CARTESIAN_POINT ( 'NONE',  ( 0.3459972005394982286, -9.006862989983986267, -9.494064636159277981 ) ) ;
#163144=EDGE_LOOP ( 'NONE', ( #166734, #122342, #169045, #87109 ) ) ;
#163148=DIRECTION ( 'NONE',  ( 0.7408284471490506062, -1.804614770759932615E-12, -0.6716942845482062330 ) ) ;
#163169=ADVANCED_FACE ( 'NONE', ( #179111 ), #65989, .T. ) ;
#163190=AXIS2_PLACEMENT_3D ( 'NONE', #24009, #74915, #190776 ) ;
#163208=B_SPLINE_CURVE_WITH_KNOTS ( 'NONE', 3,
 ( #168991, #35786, #117106, #135442, #186295, #153819, #201463, #136511, #86676, #21635 ),
 .UNSPECIFIED., .F., .F.,
 ( 4, 2, 2, 2, 4 ),
 ( 0.000000000000000000, 0.0002554020510936944391, 0.0005108041021873888782, 0.0007662061532810833173, 0.001021608204374777756 ),
 .UNSPECIFIED. ) ;
#163245=LINE ( 'NONE', #14828, #133598 ) ;
#163246=MECHANICAL_DESIGN_GEOMETRIC_PRESENTATION_REPRESENTATION('',(#114901),#529);
#163312=CARTESIAN_POINT ( 'NONE',  ( 0.000000000000000000, -9.900000000000005684, 9.579665964948883783 ) ) ;
#163321=EDGE_CURVE ( 'NONE', #157333, #166808, #100501, .T. ) ;
#163322=CARTESIAN_POINT ( 'NONE',  ( 9.495705940876563389, -8.203192640252447987, -0.2943368945747614762 ) ) ;
#163323=CARTESIAN_POINT ( 'NONE',  ( -1.040834085586084257E-14, -9.900000000000005684, -9.579665964948867796 ) ) ;
#163351=ORIENTED_EDGE ( 'NONE', *, *, #169868, .T. ) ;
#163367=AXIS2_PLACEMENT_3D ( 'NONE', #37822, #92992, #59398 ) ;
#163418=VECTOR ( 'NONE', #201478, 1000.000000000000000 ) ;
#163438=CARTESIAN_POINT ( 'NONE',  ( -9.499766273075886502, -9.919999999999998153, 0.06663900456894958357 ) ) ;
#163464=CARTESIAN_POINT ( 'NONE',  ( -10.16279779336428035, 3.829867255648772950, 5.736760595005079288 ) ) ;
#163465=CARTESIAN_POINT ( 'NONE',  ( -8.103009739377986520, -6.893137084989842123, 7.439168848974023973 ) ) ;
#163468=CARTESIAN_POINT ( 'NONE',  ( -10.71948157449083183, -8.605866298766125411, 0.1871092468795332309 ) ) ;
#163481=CIRCLE ( 'NONE', #177241, 10.99999999999999112 ) ;
#163484=MECHANICAL_DESIGN_GEOMETRIC_PRESENTATION_REPRESENTATION('',(#87406),#170422);
#163494=ORIENTED_EDGE ( 'NONE', *, *, #57019, .F. ) ;
#163527=CARTESIAN_POINT ( 'NONE',  ( -6.455298931196955969, -8.176227052203554280, -7.002681350352330192 ) ) ;
#163559=VERTEX_POINT ( 'NONE', #94979 ) ;
#163579=ORIENTED_EDGE ( 'NONE', *, *, #103623, .F. ) ;
#163581=AXIS2_PLACEMENT_3D ( 'NONE', #116011, #81321, #32567 ) ;
#163583=CARTESIAN_POINT ( 'NONE',  ( 0.01492019832702046536, -9.953727901176275594, 9.579640682430678567 ) ) ;
#163602=CARTESIAN_POINT ( 'NONE',  ( -10.38614328979761403, 3.507114751586604129, 5.996442624206741456 ) ) ;
#163613=CARTESIAN_POINT ( 'NONE',  ( 10.39025099420818776, 3.467171072964057910, 5.998814208453757679 ) ) ;
#163621=DIRECTION ( 'NONE',  ( 0.000000000000000000, 1.000000000000000000, 0.000000000000000000 ) ) ;
#163622=VERTEX_POINT ( 'NONE', #209749 ) ;
#163663=ORIENTED_EDGE ( 'NONE', *, *, #214161, .F. ) ;
#163666=CARTESIAN_POINT ( 'NONE',  ( 7.898971854500432636E-16, 4.000000000000003553, -6.450000000000003730 ) ) ;
#163678=CIRCLE ( 'NONE', #66678, 0.08000000000000001554 ) ;
#163690=CARTESIAN_POINT ( 'NONE',  ( -9.578932859269652766, -9.985077769980607698, 0.1209251627559742304 ) ) ;
#163693=DIRECTION ( 'NONE',  ( 0.000000000000000000, 0.000000000000000000, 1.000000000000000000 ) ) ;
#163701=AXIS2_PLACEMENT_3D ( 'NONE', #137352, #35550, #151460 ) ;
#163706=EDGE_LOOP ( 'NONE', ( #100250, #207499, #76437, #79730 ) ) ;
#163727=ORIENTED_EDGE ( 'NONE', *, *, #49388, .T. ) ;
#163740=ORIENTED_EDGE ( 'NONE', *, *, #100809, .F. ) ;
#163779=ORIENTED_EDGE ( 'NONE', *, *, #156034, .F. ) ;
#163781=CARTESIAN_POINT ( 'NONE',  ( 10.87247189006428272, -6.708723052947949128, -0.1888596022590607604 ) ) ;
#163786=CARTESIAN_POINT ( 'NONE',  ( 6.381095703207991576, -8.233137084989849086, 7.037870247915948063 ) ) ;
#163791=CARTESIAN_POINT ( 'NONE',  ( 10.91804383151480096, -9.900000000000005684, -0.1905751639681742271 ) ) ;
#163799=CARTESIAN_POINT ( 'NONE',  ( 7.439168848973994663, -6.893137084989842123, 8.103009739378013165 ) ) ;
#163807=ORIENTED_EDGE ( 'NONE', *, *, #162856, .F. ) ;
#163817=ORIENTED_EDGE ( 'NONE', *, *, #97172, .T. ) ;
#163824=CARTESIAN_POINT ( 'NONE',  ( -6.773376349083143566, -7.473374494058229622, -6.661184041420940005 ) ) ;
#163829=CARTESIAN_POINT ( 'NONE',  ( 0.2977236940312242286, -5.250949308401983373, 10.97067990664316284 ) ) ;
#163849=EDGE_LOOP ( 'NONE', ( #31338, #17623, #170078, #14979 ) ) ;
#163866=CIRCLE ( 'NONE', #153487, 0.08000000000000020983 ) ;
#163880=EDGE_LOOP ( 'NONE', ( #96477, #85541, #128367, #13075 ) ) ;
#163895=CARTESIAN_POINT ( 'NONE',  ( 0.07971467182324797063, -9.904506264776385294, 9.499665578938850885 ) ) ;
#163920=CARTESIAN_POINT ( 'NONE',  ( -9.488641820551102057, -8.233137084989836652, 0.4644097342743139234 ) ) ;
#163961=EDGE_CURVE ( 'NONE', #160452, #144836, #88934, .T. ) ;
#164009=EDGE_CURVE ( 'NONE', #102475, #18521, #188865, .T. ) ;
#164016=CIRCLE ( 'NONE', #170949, 6.277139874739035008 ) ;
#164113=CARTESIAN_POINT ( 'NONE',  ( 0.000000000000000000, -7.154544010627095219, 0.000000000000000000 ) ) ;
#164125=EDGE_CURVE ( 'NONE', #39263, #67222, #21002, .T. ) ;
#164129=LINE ( 'NONE', #145781, #209631 ) ;
#164131=CARTESIAN_POINT ( 'NONE',  ( -2.331034670843834533E-15, -6.124285368610726366, 10.93005900551663956 ) ) ;
#164144=CARTESIAN_POINT ( 'NONE',  ( 0.04208621775141611898, -6.437359833193938563, 10.89523958697327011 ) ) ;
#164147=DIRECTION ( 'NONE',  ( 0.000000000000000000, 1.000000000000000000, 0.000000000000000000 ) ) ;
#164174=CARTESIAN_POINT ( 'NONE',  ( -9.899039292890925879, 2.972657967447106309, -6.161878781003700567 ) ) ;
#164178=CARTESIAN_POINT ( 'NONE',  ( 10.99126615174919053, -5.166862915010145052, -0.4382560683119158251 ) ) ;
#164189=CARTESIAN_POINT ( 'NONE',  ( 6.775479680898690127, -7.217880409000396291, -6.775479680898708779 ) ) ;
#164205=CARTESIAN_POINT ( 'NONE',  ( -7.721398836998398352, 0.000000000000000000, -7.721398836998361936 ) ) ;
#164207=CARTESIAN_POINT ( 'NONE',  ( -9.597420367780070904, -7.030163990561721477, 0.01387835396683562671 ) ) ;
#164246=CARTESIAN_POINT ( 'NONE',  ( -0.3591838038534946875, -8.233137084989865073, -9.493791972417884750 ) ) ;
#164250=CARTESIAN_POINT ( 'NONE',  ( 5.301814855701348250, 1.000000000000000888, 1.561251128379126385E-14 ) ) ;
#164276=ORIENTED_EDGE ( 'NONE', *, *, #24925, .F. ) ;
#164280=CIRCLE ( 'NONE', #195512, 10.24999999999998934 ) ;
#164289=CARTESIAN_POINT ( 'NONE',  ( -10.91914056351827256, 3.934209603697781166, 3.813461610467995921 ) ) ;
#164291=CARTESIAN_POINT ( 'NONE',  ( -0.3870642018030946430, -8.176227079964629496, -9.516228778038646752 ) ) ;
#164300=CARTESIAN_POINT ( 'NONE',  ( 0.000000000000000000, -8.233137084989849086, 0.000000000000000000 ) ) ;
#164301=CIRCLE ( 'NONE', #88223, 6.277139874739035008 ) ;
#164306=AXIS2_PLACEMENT_3D ( 'NONE', #148164, #129854, #133000 ) ;
#164319=CARTESIAN_POINT ( 'NONE',  ( -8.002408263929950749, -6.836568542494915413, 7.346809171966868668 ) ) ;
#164346=SURFACE_STYLE_USAGE ( .BOTH. , #78815 ) ;
#164347=AXIS2_PLACEMENT_3D ( 'NONE', #9573, #83087, #48489 ) ;
#164350=EDGE_CURVE ( 'NONE', #201589, #148930, #119665, .T. ) ;
#164383=CARTESIAN_POINT ( 'NONE',  ( 10.99915817693633713, -6.765468805240992367, -0.1539349733294627931 ) ) ;
#164424=CARTESIAN_POINT ( 'NONE',  ( 0.4373225248172875057, -7.723431457505085085, -10.96785329849812385 ) ) ;
#164459=ORIENTED_EDGE ( 'NONE', *, *, #155215, .F. ) ;
#164494=CARTESIAN_POINT ( 'NONE',  ( -9.499386779316207452, -9.999529051968231386, 0.1207253440360574054 ) ) ;
#164504=ORIENTED_EDGE ( 'NONE', *, *, #183495, .F. ) ;
#164517=CARTESIAN_POINT ( 'NONE',  ( 0.000000000000000000, 4.000000000000003553, 0.000000000000000000 ) ) ;
#164527=VERTEX_POINT ( 'NONE', #77246 ) ;
#164531=B_SPLINE_CURVE_WITH_KNOTS ( 'NONE', 3,
 ( #84243, #213157, #180674, #19231, #134100, #85311, #133029, #50677, #116802, #48561, #196924, #200109, #98366, #130931, #65823, #199029 ),
 .UNSPECIFIED., .F., .F.,
 ( 4, 3, 3, 3, 3, 4 ),
 ( 0.000000000000000000, 3.357822776042542455E-05, 6.715700932737186327E-05, 0.0001007352753633149715, 0.0001343124815392907664, 0.0001562160020015795762 ),
 .UNSPECIFIED. ) ;
#164606=COLOUR_RGB ( '', 0.08235294, 0.09019608, 0.10196078) ;
#164629=CARTESIAN_POINT ( 'NONE',  ( -10.98997987423604172, -6.893137084989842123, 0.4694063952341877011 ) ) ;
#164633=ORIENTED_EDGE ( 'NONE', *, *, #111938, .T. ) ;
#164643=TOROIDAL_SURFACE ( 'NONE', #133449, 10.92000000000000171, 0.08000000000000000167 ) ;
#164648=LINE ( 'NONE', #83378, #135948 ) ;
#164675=ORIENTED_EDGE ( 'NONE', *, *, #38065, .F. ) ;
#164689=CARTESIAN_POINT ( 'NONE',  ( 10.85699613887011772, -6.836286050428144634, -0.3891817118475866533 ) ) ;
#164694=CARTESIAN_POINT ( 'NONE',  ( -10.85353573482952072, -6.836568542495036205, 0.4635785636673775967 ) ) ;
#164703=CARTESIAN_POINT ( 'NONE',  ( -0.09500528524172231759, -5.338246727548288995, -10.99984294789629935 ) ) ;
#164713=CARTESIAN_POINT ( 'NONE',  ( -0.1817359287055335115, -9.181675805132242019, 9.625413980971107009 ) ) ;
#164738=CARTESIAN_POINT ( 'NONE',  ( 6.637758778446686492, -7.996947095390841476, 6.849430810391425872 ) ) ;
#164741=DIRECTION ( 'NONE',  ( 0.000000000000000000, 1.000000000000000000, 0.000000000000000000 ) ) ;
#164748=EDGE_CURVE ( 'NONE', #105884, #32900, #65472, .T. ) ;
#164757=ORIENTED_EDGE ( 'NONE', *, *, #33674, .T. ) ;
#164791=ORIENTED_EDGE ( 'NONE', *, *, #153405, .T. ) ;
#164797=ORIENTED_EDGE ( 'NONE', *, *, #48830, .T. ) ;
#164832=CARTESIAN_POINT ( 'NONE',  ( 6.776587425048107960, -7.030236945366980628, 6.796206128891409293 ) ) ;
#164835=LINE ( 'NONE', #198377, #184243 ) ;
#164892=CARTESIAN_POINT ( 'NONE',  ( -9.905860218026552033, -6.920331743278818060, 1.138412281109779656E-15 ) ) ;
#164909=CARTESIAN_POINT ( 'NONE',  ( -6.773846765316632990, -7.473374494057232198, -6.773846765316600127 ) ) ;
#164924=ORIENTED_EDGE ( 'NONE', *, *, #183495, .T. ) ;
#164948=TOROIDAL_SURFACE ( 'NONE', #171755, 10.92000000000000348, 0.08000000000000000167 ) ;
#164963=CARTESIAN_POINT ( 'NONE',  ( 0.000000000000000000, 0.000000000000000000, 0.000000000000000000 ) ) ;
#164965=CARTESIAN_POINT ( 'NONE',  ( -9.499668754385632852, -7.473374494045003757, -0.07933194154487524519 ) ) ;
#165017=EDGE_CURVE ( 'NONE', #100589, #187284, #128437, .T. ) ;
#165019=( NAMED_UNIT ( * ) SI_UNIT ( $, .STERADIAN. ) SOLID_ANGLE_UNIT ( ) );
#165063=VECTOR ( 'NONE', #189110, 1000.000000000000000 ) ;
#165066=EDGE_CURVE ( 'NONE', #137099, #36083, #45319, .T. ) ;
#165074=EDGE_CURVE ( 'NONE', #60029, #96467, #52852, .T. ) ;
#165130=CARTESIAN_POINT ( 'NONE',  ( -10.99935770452674610, -5.294776013890323263, 0.1368885365587619307 ) ) ;
#165134=FACE_OUTER_BOUND ( 'NONE', #208726, .T. ) ;
#165149=VERTEX_POINT ( 'NONE', #20763 ) ;
#165173=CARTESIAN_POINT ( 'NONE',  ( 9.484513307599968357, -6.630981389236904278, -0.1588444833727744865 ) ) ;
#165190=FACE_OUTER_BOUND ( 'NONE', #66367, .T. ) ;
#165205=EDGE_CURVE ( 'NONE', #56213, #91101, #37106, .T. ) ;
#165224=SURFACE_SIDE_STYLE ('',( #111224 ) ) ;
#165227=FACE_OUTER_BOUND ( 'NONE', #131705, .T. ) ;
#165254=ORIENTED_EDGE ( 'NONE', *, *, #143150, .T. ) ;
#165260=CARTESIAN_POINT ( 'NONE',  ( -7.214015694910790089, -7.024005795613424752, -7.869907041762409960 ) ) ;
#165307=( NAMED_UNIT ( * ) SI_UNIT ( $, .STERADIAN. ) SOLID_ANGLE_UNIT ( ) );
#165319=ORIENTED_EDGE ( 'NONE', *, *, #187677, .T. ) ;
#165328=ORIENTED_EDGE ( 'NONE', *, *, #158729, .T. ) ;
#165378=FACE_OUTER_BOUND ( 'NONE', #61711, .T. ) ;
#165392=ORIENTED_EDGE ( 'NONE', *, *, #44272, .F. ) ;
#165445=DIRECTION ( 'NONE',  ( 0.000000000000000000, 0.000000000000000000, -1.000000000000000000 ) ) ;
#165460=CARTESIAN_POINT ( 'NONE',  ( 10.43434622977930637, 1.529612873802629336, -5.577395135400672110 ) ) ;
#165466=EDGE_LOOP ( 'NONE', ( #128053, #127819, #158267, #101467 ) ) ;
#165491=FILL_AREA_STYLE ('',( #99436 ) ) ;
#165521=ADVANCED_FACE ( 'NONE', ( #189679 ), #98775, .T. ) ;
#165559=( NAMED_UNIT ( * ) PLANE_ANGLE_UNIT ( ) SI_UNIT ( $, .RADIAN. ) );
#165584=ADVANCED_FACE ( 'NONE', ( #26109 ), #76535, .T. ) ;
#165585=DIRECTION ( 'NONE',  ( 0.000000000000000000, 1.000000000000000000, 0.000000000000000000 ) ) ;
#165594=EDGE_CURVE ( 'NONE', #36083, #144861, #38511, .T. ) ;
#165598=VECTOR ( 'NONE', #187698, 1000.000000000000000 ) ;
#165613=CARTESIAN_POINT ( 'NONE',  ( 0.07933194018404610137, -7.215568602689907074, -9.499668754396999759 ) ) ;
#165638=DIRECTION ( 'NONE',  ( 0.000000000000000000, 1.000000000000000000, 0.000000000000000000 ) ) ;
#165639=CARTESIAN_POINT ( 'NONE',  ( -10.39230484541327826, 4.000000000000003553, -5.999999999999975131 ) ) ;
#165644=DIRECTION ( 'NONE',  ( 0.000000000000000000, -0.06195440338563660415, 0.9980789807931683688 ) ) ;
#165669=SURFACE_SIDE_STYLE ('',( #166740 ) ) ;
#165678=ORIENTED_EDGE ( 'NONE', *, *, #53487, .F. ) ;
#165700=CARTESIAN_POINT ( 'NONE',  ( 7.346809171966453889, -6.836568542494980250, 8.002408263930263388 ) ) ;
#165718=CIRCLE ( 'NONE', #55023, 6.249999999999995559 ) ;
#165729=CARTESIAN_POINT ( 'NONE',  ( -8.673617379884035472E-15, 3.507114751586604129, -11.99288524841337455 ) ) ;
#165740=ORIENTED_EDGE ( 'NONE', *, *, #4542, .T. ) ;
#165743=B_SPLINE_CURVE_WITH_KNOTS ( 'NONE', 3,
 ( #142601, #110139, #143685, #11490, #209677, #61321, #155258 ),
 .UNSPECIFIED., .F., .F.,
 ( 4, 3, 4 ),
 ( 0.0001135037245265561694, 0.001517139415464327252, 0.002007692284160942763 ),
 .UNSPECIFIED. ) ;
#165782=CARTESIAN_POINT ( 'NONE',  ( -10.38614328979761403, 3.507114751586604129, 5.996442624206741456 ) ) ;
#165783=PRESENTATION_STYLE_ASSIGNMENT (( #132249 ) ) ;
#165785=CARTESIAN_POINT ( 'NONE',  ( 0.000000000000000000, -7.246166700194011767, 9.579665964935665912 ) ) ;
#165813=FACE_OUTER_BOUND ( 'NONE', #176113, .T. ) ;
#165845=CARTESIAN_POINT ( 'NONE',  ( 6.824425546749162130, -8.104785249476798015, -6.609253696060804373 ) ) ;
#165850=CARTESIAN_POINT ( 'NONE',  ( -0.4350687514514777199, -7.666862915010147717, 10.91132967064556603 ) ) ;
#165876=CIRCLE ( 'NONE', #127944, 0.08000000000000020983 ) ;
#165885=B_SPLINE_CURVE_WITH_KNOTS ( 'NONE', 3,
 ( #33676, #186317, #167948, #136531, #18482, #153840 ),
 .UNSPECIFIED., .F., .F.,
 ( 4, 2, 4 ),
 ( 0.000000000000000000, 0.001225895755212353007, 0.002451791510424706014 ),
 .UNSPECIFIED. ) ;
#165905=CARTESIAN_POINT ( 'NONE',  ( -2.269535221383012225, 3.870433085555832431, 11.40607948006776873 ) ) ;
#165915=CARTESIAN_POINT ( 'NONE',  ( 6.493979435825333546, -7.868711954889218596, -6.493979435825359303 ) ) ;
#165930=CARTESIAN_POINT ( 'NONE',  ( -9.132253115921022513, 1.016282880930314603, -8.222717639126782885 ) ) ;
#165979=CARTESIAN_POINT ( 'NONE',  ( -6.710064404886794343, -7.791858861492868549, -6.725651841507029438 ) ) ;
#165994=ORIENTED_EDGE ( 'NONE', *, *, #184771, .F. ) ;
#166000=CARTESIAN_POINT ( 'NONE',  ( -3.276785236921248415E-13, -7.217880409008451181, 9.581975256308824740 ) ) ;
#166010=CARTESIAN_POINT ( 'NONE',  ( 10.99947830037066510, -9.912501460265211506, -0.1071380031274375144 ) ) ;
#166016=EDGE_CURVE ( 'NONE', #74942, #82527, #69711, .T. ) ;
#166038=EDGE_CURVE ( 'NONE', #179210, #101997, #14084, .T. ) ;
#166070=CARTESIAN_POINT ( 'NONE',  ( 10.42871741020797494, 1.405922845961228962, -5.936700867306154983 ) ) ;
#166097=ORIENTED_EDGE ( 'NONE', *, *, #181792, .F. ) ;
#166138=DIRECTION ( 'NONE',  ( 0.000000000000000000, -1.000000000000000000, 0.000000000000000000 ) ) ;
#166198=ADVANCED_FACE ( 'NONE', ( #154795 ), #97511, .T. ) ;
#166203=CIRCLE ( 'NONE', #72805, 10.99999999999999112 ) ;
#166210=ORIENTED_EDGE ( 'NONE', *, *, #186483, .T. ) ;
#166214=EDGE_CURVE ( 'NONE', #74967, #71109, #8720, .T. ) ;
#166224=B_SPLINE_CURVE_WITH_KNOTS ( 'NONE', 3,
 ( #110815, #46843, #144369, #178968, #96665, #160566, #164832, #176820 ),
 .UNSPECIFIED., .F., .F.,
 ( 4, 2, 2, 4 ),
 ( 0.000000000000000000, 0.0001985720215089308081, 0.0003971440430178616162, 0.0007942880860357254009 ),
 .UNSPECIFIED. ) ;
#166238=CARTESIAN_POINT ( 'NONE',  ( 9.488025208946959665, -6.683951901172175525, -0.1062647697984070022 ) ) ;
#166279=EDGE_CURVE ( 'NONE', #128654, #130349, #39400, .T. ) ;
#166292=CARTESIAN_POINT ( 'NONE',  ( 11.00038526257060667, -5.601932402265105360, -0.008494835128417067838 ) ) ;
#166303=DIRECTION ( 'NONE',  ( 0.6691306063588511321, 0.000000000000000000, -0.7431448254774005724 ) ) ;
#166305=CARTESIAN_POINT ( 'NONE',  ( 6.725445687907758874, -7.162053774861991684, -6.710127771514625472 ) ) ;
#166319=VERTEX_POINT ( 'NONE', #7451 ) ;
#166398=CARTESIAN_POINT ( 'NONE',  ( 9.500331257164623011, -7.246166700193447774, 1.020301583428166389E-12 ) ) ;
#166437=CARTESIAN_POINT ( 'NONE',  ( -7.777967379493323286, -9.999999999999994671, -7.664830294503433450 ) ) ;
#166501=EDGE_LOOP ( 'NONE', ( #6833, #179317, #111766, #30788 ) ) ;
#166507=EDGE_CURVE ( 'NONE', #58157, #119756, #104733, .T. ) ;
#166582=CARTESIAN_POINT ( 'NONE',  ( 0.09999999999999592548, -9.999999999999994671, 10.91954211494236660 ) ) ;
#166708=DIRECTION ( 'NONE',  ( 0.2079116908177593703, 0.000000000000000000, -0.9781476007338056888 ) ) ;
#166734=ORIENTED_EDGE ( 'NONE', *, *, #77763, .T. ) ;
#166740=SURFACE_STYLE_FILL_AREA ( #99602 ) ;
#166752=EDGE_CURVE ( 'NONE', #12663, #209328, #116949, .T. ) ;
#166781=CARTESIAN_POINT ( 'NONE',  ( -6.778728372092626131, -7.783114986501003862, 6.734029298721179835 ) ) ;
#166799=EDGE_CURVE ( 'NONE', #142721, #189233, #59377, .T. ) ;
#166808=VERTEX_POINT ( 'NONE', #123205 ) ;
#166817=EDGE_CURVE ( 'NONE', #173465, #87461, #42111, .T. ) ;
#166824=CARTESIAN_POINT ( 'NONE',  ( 10.98997987423603995, -6.700000000000007283, -0.4694063952341755996 ) ) ;
#166825=CARTESIAN_POINT ( 'NONE',  ( -0.4373349612950744869, -5.212340523078053955, -10.97895254167817569 ) ) ;
#166843=ORIENTED_EDGE ( 'NONE', *, *, #32207, .T. ) ;
#166919=CARTESIAN_POINT ( 'NONE',  ( -8.654705636516467323E-15, -6.148216694138043614, -10.67870335800435733 ) ) ;
#166933=ORIENTED_EDGE ( 'NONE', *, *, #187696, .F. ) ;
#166960=CARTESIAN_POINT ( 'NONE',  ( -2.093037498677872144, 1.000000000000000888, 11.70868840297834446 ) ) ;
#166971=ORIENTED_EDGE ( 'NONE', *, *, #175161, .F. ) ;
#166977=CARTESIAN_POINT ( 'NONE',  ( 9.617648866954041864, -9.063431457505050304, -0.6035590660245153671 ) ) ;
#167008=ORIENTED_EDGE ( 'NONE', *, *, #175161, .T. ) ;
#167030=DIRECTION ( 'NONE',  ( 0.000000000000000000, 0.000000000000000000, 1.000000000000000000 ) ) ;
#167040=ORIENTED_EDGE ( 'NONE', *, *, #18222, .F. ) ;
#167045=LINE ( 'NONE', #151866, #174242 ) ;
#167123=CARTESIAN_POINT ( 'NONE',  ( -10.94245301910280865, 3.162178953954597471, 3.962121973755150073 ) ) ;
#167127=COLOUR_RGB ( '', 0.08235294, 0.09019608, 0.10196078) ;
#167205=CARTESIAN_POINT ( 'NONE',  ( -7.173763318588748383, -6.681223591462298828, -7.173763318588716409 ) ) ;
#167216=VERTEX_POINT ( 'NONE', #94047 ) ;
#167233=CARTESIAN_POINT ( 'NONE',  ( -10.91970695577496997, -5.907420853759282053, 5.204170427930421283E-15 ) ) ;
#167253=CARTESIAN_POINT ( 'NONE',  ( 0.000000000000000000, 0.03624871340549007392, 0.000000000000000000 ) ) ;
#167259=AXIS2_PLACEMENT_3D ( 'NONE', #41257, #40175, #105191 ) ;
#167313=CARTESIAN_POINT ( 'NONE',  ( 9.500587730663498931, -7.019129742886753398, -0.03636482241200242327 ) ) ;
#167319=CARTESIAN_POINT ( 'NONE',  ( 6.743487189264861570, -7.020359948792185278, -6.692370362267389794 ) ) ;
#167329=TOROIDAL_SURFACE ( 'NONE', #11627, 10.92000000000000171, 0.08000000000000000167 ) ;
#167331=CARTESIAN_POINT ( 'NONE',  ( 6.764898216730270697, -7.628386336122854772, -6.764898216727333491 ) ) ;
#167358=ORIENTED_EDGE ( 'NONE', *, *, #156758, .T. ) ;
#167388=CARTESIAN_POINT ( 'NONE',  ( -0.08000000000000714873, -9.999999999999994671, 10.91970695577494865 ) ) ;
#167467=EDGE_LOOP ( 'NONE', ( #42343, #68509, #64639, #37726 ) ) ;
#167487=CARTESIAN_POINT ( 'NONE',  ( 10.98677171181892476, -7.666863022245585135, -0.5458515184425005717 ) ) ;
#167505=CARTESIAN_POINT ( 'NONE',  ( -9.590330253158105833, -9.597646708343960498, 0.1673998372498867182 ) ) ;
#167509=EDGE_CURVE ( 'NONE', #82895, #66830, #42087, .T. ) ;
#167511=EDGE_LOOP ( 'NONE', ( #210330, #12062, #209539, #153430 ) ) ;
#167520=CARTESIAN_POINT ( 'NONE',  ( -1.084202172485504434E-15, -6.705807707623162806, -10.34804402329775108 ) ) ;
#167539=TOROIDAL_SURFACE ( 'NONE', #50049, 9.580000000000003624, 0.08000000000000000167 ) ;
#167540=CARTESIAN_POINT ( 'NONE',  ( -10.91812205866965257, -9.932868363016991609, 0.1856806763506273772 ) ) ;
#167630=CARTESIAN_POINT ( 'NONE',  ( 0.000000000000000000, -8.233137084989836652, 0.000000000000000000 ) ) ;
#167635=VERTEX_POINT ( 'NONE', #134814 ) ;
#167713=SURFACE_STYLE_USAGE ( .BOTH. , #101646 ) ;
#167722=CARTESIAN_POINT ( 'NONE',  ( -9.499668754385638181, -7.473374494045003757, -0.07933194154487506478 ) ) ;
#167841=CARTESIAN_POINT ( 'NONE',  ( -6.396834479292370368, -8.176568542494905500, -7.055228938194266775 ) ) ;
#167847=TOROIDAL_SURFACE ( 'NONE', #199040, 10.92000000000000171, 0.08000000000000000167 ) ;
#167848=CARTESIAN_POINT ( 'NONE',  ( 10.93020303578476238, -8.258458176070773149, -0.1907874036681889707 ) ) ;
#167866=FILL_AREA_STYLE_COLOUR ( '', #9742 ) ;
#167875=FACE_OUTER_BOUND ( 'NONE', #65020, .T. ) ;
#167891=EDGE_CURVE ( 'NONE', #90575, #115124, #98878, .T. ) ;
#167897=ADVANCED_FACE ( 'NONE', ( #156151 ), #155688, .T. ) ;
#167909=LINE ( 'NONE', #19507, #57813 ) ;
#167948=CARTESIAN_POINT ( 'NONE',  ( -11.39849338755883323, 1.813773193624679925, 3.751625886033604917 ) ) ;
#167974=CARTESIAN_POINT ( 'NONE',  ( -6.895452369244193136, -6.747656629766889402, 6.524021554744679818 ) ) ;
#167976=CARTESIAN_POINT ( 'NONE',  ( 11.39849338755880659, 1.813773193624685032, -3.751625886033683077 ) ) ;
#167977=CARTESIAN_POINT ( 'NONE',  ( -7.553974597844363537, -6.709380320845435008, -7.821934338880122795 ) ) ;
#168033=CARTESIAN_POINT ( 'NONE',  ( 9.623574082427451160, -9.090902906714891429, -0.4644248560400533465 ) ) ;
#168040=DIRECTION ( 'NONE',  ( 0.000000000000000000, 0.000000000000000000, -1.000000000000000000 ) ) ;
#168062=CARTESIAN_POINT ( 'NONE',  ( -9.007749180432204739, 1.970899860167778073, -7.589917856500828286 ) ) ;
#168066=CARTESIAN_POINT ( 'NONE',  ( -7.439168848973790382, -6.700000000000001066, -8.103009739378192577 ) ) ;
#168094=CARTESIAN_POINT ( 'NONE',  ( 6.773376349083131132, 7.849261790823902629, 6.661184041420955992 ) ) ;
#168116=CARTESIAN_POINT ( 'NONE',  ( -6.439526774797413644, -8.199734048662943309, -6.984891963203985199 ) ) ;
#168118=CARTESIAN_POINT ( 'NONE',  ( 9.499766273075866962, -9.919999999999998153, -0.06663900456893058488 ) ) ;
#168134=CARTESIAN_POINT ( 'NONE',  ( 0.000000000000000000, -11.15905291171102931, 0.000000000000000000 ) ) ;
#168147=CARTESIAN_POINT ( 'NONE',  ( 6.935047222998001359, -6.682123388834269484, -6.658747417466178931 ) ) ;
#168223=CARTESIAN_POINT ( 'NONE',  ( 0.04582610853910489696, -10.00039265882532646, 11.00004154231811526 ) ) ;
#168282=AXIS2_PLACEMENT_3D ( 'NONE', #90306, #172626, #22055 ) ;
#168326=CARTESIAN_POINT ( 'NONE',  ( 0.000000000000000000, -0.9200000000000041478, 0.000000000000000000 ) ) ;
#168335=CARTESIAN_POINT ( 'NONE',  ( 2.554955805669727020, 1.016282880930317933, -12.02012201174058603 ) ) ;
#168390=CARTESIAN_POINT ( 'NONE',  ( 10.99931692196006949, -8.074346042903146170, -0.1488091642035823670 ) ) ;
#168391=CARTESIAN_POINT ( 'NONE',  ( -6.684387857553246270, -6.724344753046691103, -6.908358566921309674 ) ) ;
#168437=CARTESIAN_POINT ( 'NONE',  ( 6.781144757626056396, -7.161464053357567749, -6.776370306708062508 ) ) ;
#168456=CARTESIAN_POINT ( 'NONE',  ( 10.79920600060117586, -6.027819618361855092, 9.269928574751062911E-15 ) ) ;
#168532=CARTESIAN_POINT ( 'NONE',  ( -10.10343170205533880, 2.974000657017113802, 5.833219012925197511 ) ) ;
#168540=CARTESIAN_POINT ( 'NONE',  ( -10.30245174296178057, 3.603753425775780617, -5.948123287112075275 ) ) ;
#168565=CARTESIAN_POINT ( 'NONE',  ( -9.616417370072172233, -9.251786168353179463, 0.2979722244324810032 ) ) ;
#168576=CARTESIAN_POINT ( 'NONE',  ( -7.927630635717298979, -6.615717645446903994, 7.626802973668175056 ) ) ;
#168580=CARTESIAN_POINT ( 'NONE',  ( -10.95855051086948606, -7.723431457505092190, 0.6286713519884027379 ) ) ;
#168600=ORIENTED_EDGE ( 'NONE', *, *, #200299, .T. ) ;
#168602=CARTESIAN_POINT ( 'NONE',  ( -10.41509302999113018, 1.813436143228244424, 5.960384690635835092 ) ) ;
#168605=CIRCLE ( 'NONE', #130657, 0.08000000000000020983 ) ;
#168636=VERTEX_POINT ( 'NONE', #165729 ) ;
#168717=EDGE_CURVE ( 'NONE', #114731, #183021, #199748, .T. ) ;
#168774=ORIENTED_EDGE ( 'NONE', *, *, #186635, .T. ) ;
#168784=CARTESIAN_POINT ( 'NONE',  ( -9.500479199177402023, -7.792108994755980511, 0.01138762994425606724 ) ) ;
#168831=PLANE ( 'NONE',  #121515 ) ;
#168883=CARTESIAN_POINT ( 'NONE',  ( 6.513344551206667887E-14, -9.900000000000005684, -9.500331257164612353 ) ) ;
#168888=VERTEX_POINT ( 'NONE', #156688 ) ;
#168923=DIRECTION ( 'NONE',  ( -5.551115123125783935E-17, 0.7071067811865536790, 0.7071067811865413555 ) ) ;
#168925=PRESENTATION_STYLE_ASSIGNMENT (( #69266 ) ) ;
#168936=CARTESIAN_POINT ( 'NONE',  ( -10.98765602437504185, -5.221050908132831125, 1.680513367352532070E-15 ) ) ;
#168943=CARTESIAN_POINT ( 'NONE',  ( 11.29517787156874498, -8.030538574678857344, -0.1971580631239572556 ) ) ;
#168944=CARTESIAN_POINT ( 'NONE',  ( -1.138412281109779656E-15, -6.105866302528341727, -10.72111444838821193 ) ) ;
#168959=SURFACE_STYLE_USAGE ( .BOTH. , #105056 ) ;
#168971=CARTESIAN_POINT ( 'NONE',  ( -0.2663167167779803557, -9.037303891206464712, 9.496500708127756596 ) ) ;
#168972=EDGE_CURVE ( 'NONE', #144836, #199252, #35229, .T. ) ;
#168977=( BOUNDED_SURFACE ( )  B_SPLINE_SURFACE ( 3, 2, ( 
 ( #151894, #119447, #154025 ),
 ( #18666, #54391, #55450 ),
 ( #3469, #38139, #155092 ),
 ( #186508, #56524, #121602 ),
 ( #22922, #170258, #187574 ),
 ( #53315, #70601, #37055 ),
 ( #72755, #169196, #136715 ),
 ( #184366, #20789, #39199 ) ),
 .UNSPECIFIED., .F., .F., .T. ) 
 B_SPLINE_SURFACE_WITH_KNOTS ( ( 4, 2, 2, 4 ),
 ( 3, 3 ),
 ( 5.421010862427522170E-20, 0.0004401918256853566084, 0.0006602877385280349126, 0.0008803836513707132168 ),
 ( 0.000000000000000000, 1.000000000000000000 ),
 .UNSPECIFIED. ) 
 GEOMETRIC_REPRESENTATION_ITEM ( )  RATIONAL_B_SPLINE_SURFACE ( (
 ( 1.000000000000000000, 0.6787756258918292707, 1.000000000000000000),
 ( 1.000000000000000000, 0.6284487096097822745, 1.000000000000000000),
 ( 1.000000000000000000, 0.5704014816686249212, 1.000000000000000000),
 ( 1.000000000000000000, 0.4882303283128048288, 1.000000000000000000),
 ( 1.000000000000000000, 0.4617370933884766271, 1.000000000000000000),
 ( 1.000000000000000000, 0.4222438920366224369, 1.000000000000000000),
 ( 1.000000000000000000, 0.4105126989450484376, 1.000000000000000000),
 ( 1.000000000000000000, 0.4127341956165116454, 1.000000000000000000) ) ) 
 REPRESENTATION_ITEM ( '' )  SURFACE ( )  );
#168991=CARTESIAN_POINT ( 'NONE',  ( 9.499668754385636404, -7.473374494045003757, 0.07933194154488391880 ) ) ;
#169005=AXIS2_PLACEMENT_3D ( 'NONE', #60677, #7649, #44456 ) ;
#169035=CARTESIAN_POINT ( 'NONE',  ( -6.785280070212318826, -6.896483513897296191, 6.645879322773594389 ) ) ;
#169045=ORIENTED_EDGE ( 'NONE', *, *, #102286, .T. ) ;
#169059=CARTESIAN_POINT ( 'NONE',  ( 1.255262969126037044E-15, -2.000000000000001776, -10.24999999999999822 ) ) ;
#169067=CARTESIAN_POINT ( 'NONE',  ( -0.001123102408844807139, -7.189630408304394926, -9.584291988782274174 ) ) ;
#169072=DIRECTION ( 'NONE',  ( -0.9983585005135561241, 0.000000000000000000, 0.05727394217551147471 ) ) ;
#169078=CARTESIAN_POINT ( 'NONE',  ( -8.064677165291199046, -5.223431457505083308, 7.446209719563363194 ) ) ;
#169098=CARTESIAN_POINT ( 'NONE',  ( -10.89523958697326833, -6.437359833193948333, 0.04208621775142193377 ) ) ;
#169110=CARTESIAN_POINT ( 'NONE',  ( 0.007601003541776819861, -8.259585062615352413, -10.93184718803891187 ) ) ;
#169158=CARTESIAN_POINT ( 'NONE',  ( 0.07933194154487524519, -9.746166700180788567, 9.499668754385634628 ) ) ;
#169160=CARTESIAN_POINT ( 'NONE',  ( -2.331034670843834533E-15, -6.681160345272283863, 10.14529669463342998 ) ) ;
#169169=DIRECTION ( 'NONE',  ( 0.000000000000000000, 0.000000000000000000, 1.000000000000000000 ) ) ;
#169174=DIRECTION ( 'NONE',  ( 0.000000000000000000, 0.000000000000000000, 1.000000000000000000 ) ) ;
#169196=CARTESIAN_POINT ( 'NONE',  ( 6.429544252029160134, -6.709867743870938206, 6.981856502303465106 ) ) ;
#169199=CARTESIAN_POINT ( 'NONE',  ( -10.99126615174920651, -5.166862915010145052, 0.4382560683119391398 ) ) ;
#169221=CARTESIAN_POINT ( 'NONE',  ( -6.661184041420952440, 7.849261790823902629, 6.773376349083140013 ) ) ;
#169230=CARTESIAN_POINT ( 'NONE',  ( -0.01492019832703625482, -9.953727901176275594, -9.579640682430666132 ) ) ;
#169231=EDGE_CURVE ( 'NONE', #176800, #137099, #166203, .T. ) ;
#169234=ORIENTED_EDGE ( 'NONE', *, *, #40097, .T. ) ;
#169348=DIRECTION ( 'NONE',  ( 0.000000000000000000, 0.000000000000000000, 1.000000000000000000 ) ) ;
#169386=( NAMED_UNIT ( * ) PLANE_ANGLE_UNIT ( ) SI_UNIT ( $, .RADIAN. ) );
#169387=EDGE_CURVE ( 'NONE', #148587, #18521, #3669, .T. ) ;
#169395=CARTESIAN_POINT ( 'NONE',  ( -10.91970695577495576, -5.907420853759283830, 8.456776945386934585E-15 ) ) ;
#169405=CARTESIAN_POINT ( 'NONE',  ( 0.04225267894259320672, -6.625438066542582938, 11.00000000000012257 ) ) ;
#169411=FACE_OUTER_BOUND ( 'NONE', #117025, .T. ) ;
#169438=CARTESIAN_POINT ( 'NONE',  ( 9.497255425109827343, -6.896119493545203483, -0.09872732973945687329 ) ) ;
#169447=EDGE_LOOP ( 'NONE', ( #199509, #9353, #20459, #39414 ) ) ;
#169452=CARTESIAN_POINT ( 'NONE',  ( 10.99943592164172657, -8.407420853759269619, -0.1113975120798811613 ) ) ;
#169453=CARTESIAN_POINT ( 'NONE',  ( 6.778728372092623466, -7.783114986501003862, -6.734029298721178947 ) ) ;
#169461=CARTESIAN_POINT ( 'NONE',  ( 7.986233326679963440, -6.863455982311493564, -7.564733433744406987 ) ) ;
#169462=CIRCLE ( 'NONE', #38061, 0.08000000000000020983 ) ;
#169523=CARTESIAN_POINT ( 'NONE',  ( 10.55819884875827697, -6.268611901546719878, -1.734723475976807094E-15 ) ) ;
#169582=VERTEX_POINT ( 'NONE', #213074 ) ;
#169588=ORIENTED_EDGE ( 'NONE', *, *, #186726, .F. ) ;
#169614=CARTESIAN_POINT ( 'NONE',  ( 10.99856159529785060, -8.101932402265175526, -0.2004767358929940846 ) ) ;
#169627=FACE_OUTER_BOUND ( 'NONE', #25069, .T. ) ;
#169671=CARTESIAN_POINT ( 'NONE',  ( -10.91819195543077470, -9.943514287384804362, 0.1813054759508214986 ) ) ;
#169683=CARTESIAN_POINT ( 'NONE',  ( 2.480760062148268386, 4.021557182957057996, -11.67105848277438973 ) ) ;
#169714=VERTEX_POINT ( 'NONE', #33270 ) ;
#169723=B_SPLINE_CURVE_WITH_KNOTS ( 'NONE', 3,
 ( #42200, #90946, #73604, #38981, #25913, #159125, #55231 ),
 .UNSPECIFIED., .F., .F.,
 ( 4, 3, 4 ),
 ( 0.0001126021369344370733, 0.001503110988946918273, 0.002006790696425522769 ),
 .UNSPECIFIED. ) ;
#169747=EDGE_CURVE ( 'NONE', #15455, #29554, #57429, .T. ) ;
#169760=DIRECTION ( 'NONE',  ( 0.000000000000000000, -1.000000000000000000, 0.000000000000000000 ) ) ;
#169775=CARTESIAN_POINT ( 'NONE',  ( -10.99916818177030287, -10.00038292658551420, 0.1458870414460790577 ) ) ;
#169810=B_SPLINE_CURVE_WITH_KNOTS ( 'NONE', 3,
 ( #186223, #89829, #138568, #187296, #87671, #155877, #103934, #36775 ),
 .UNSPECIFIED., .F., .F.,
 ( 4, 2, 2, 4 ),
 ( 1.301042606982573158E-18, 0.0002224730689913829963, 0.0004449461379827646915, 0.0008898922759655280819 ),
 .UNSPECIFIED. ) ;
#169850=CARTESIAN_POINT ( 'NONE',  ( -9.520891725235959058, -8.148349307653482754, 0.3199376857464493740 ) ) ;
#169868=EDGE_CURVE ( 'NONE', #39263, #145242, #149155, .T. ) ;
#169881=CARTESIAN_POINT ( 'NONE',  ( -0.2633404184769205236, -6.747343053191835693, -9.488968570712991379 ) ) ;
#169921=( GEOMETRIC_REPRESENTATION_CONTEXT ( 3 ) GLOBAL_UNCERTAINTY_ASSIGNED_CONTEXT ( ( #20396 ) ) GLOBAL_UNIT_ASSIGNED_CONTEXT ( ( #111707, #25043, #61823 ) ) REPRESENTATION_CONTEXT ( 'NONE', 'WORKASPACE' ) );
#169925=CARTESIAN_POINT ( 'NONE',  ( 10.64229060209986599, 1.016282880930355681, 6.144329343916449027 ) ) ;
#169953=DIRECTION ( 'NONE',  ( -1.544526636936600361E-14, -1.000000000000000000, -1.522060196430166414E-14 ) ) ;
#169963=CARTESIAN_POINT ( 'NONE',  ( 0.3891817118475826009, -6.836286050428183714, 10.85699613887008042 ) ) ;
#169977=CARTESIAN_POINT ( 'NONE',  ( -9.481348452320373710, -9.006862915010128035, 0.5950054837411764552 ) ) ;
#169996=EDGE_CURVE ( 'NONE', #174410, #208229, #62396, .T. ) ;
#170000=ORIENTED_EDGE ( 'NONE', *, *, #118916, .T. ) ;
#170002=CARTESIAN_POINT ( 'NONE',  ( -0.4350533241460393108, -6.938200158402035633, -9.251576347356897045 ) ) ;
#170030=FACE_OUTER_BOUND ( 'NONE', #121058, .T. ) ;
#170031=CARTESIAN_POINT ( 'NONE',  ( -0.2959466228873294247, -9.091099919222520143, 9.630212118911225971 ) ) ;
#170046=AXIS2_PLACEMENT_3D ( 'NONE', #63574, #162155, #193571 ) ;
#170060=( LENGTH_UNIT ( ) NAMED_UNIT ( * ) SI_UNIT ( .MILLI., .METRE. ) );
#170072=FACE_OUTER_BOUND ( 'NONE', #74228, .T. ) ;
#170078=ORIENTED_EDGE ( 'NONE', *, *, #26823, .T. ) ;
#170096=CARTESIAN_POINT ( 'NONE',  ( 7.752014238602739730E-16, 3.000000000000000888, 6.329999999999995630 ) ) ;
#170100=VERTEX_POINT ( 'NONE', #184838 ) ;
#170125=EDGE_CURVE ( 'NONE', #96623, #58812, #183788, .T. ) ;
#170143=CARTESIAN_POINT ( 'NONE',  ( -7.747753938335002921, -5.575271019047995047, 7.808923410443626700 ) ) ;
#170153=DIRECTION ( 'NONE',  ( 0.000000000000000000, 1.000000000000000000, 0.000000000000000000 ) ) ;
#170207=CARTESIAN_POINT ( 'NONE',  ( 10.15205317230714144, 3.956598013261176217, -5.494609294606112471 ) ) ;
#170213=ORIENTED_EDGE ( 'NONE', *, *, #128877, .F. ) ;
#170232=CARTESIAN_POINT ( 'NONE',  ( 0.3046331935817621073, -6.606549254264995064, 9.611339018008543178 ) ) ;
#170243=CARTESIAN_POINT ( 'NONE',  ( 6.662120174140254925, -7.184999792969698262, -6.772456105771881951 ) ) ;
#170258=CARTESIAN_POINT ( 'NONE',  ( 6.524021554744638074, -6.747656629766706438, 6.895452369244322810 ) ) ;
#170268=TOROIDAL_SURFACE ( 'NONE', #80452, 11.70000000000000107, 0.2000000000000000111 ) ;
#170293=ORIENTED_EDGE ( 'NONE', *, *, #59579, .T. ) ;
#170299=DIRECTION ( 'NONE',  ( 0.9990890794760040050, 5.454924750823445190E-15, -0.04267330865764876885 ) ) ;
#170381=CARTESIAN_POINT ( 'NONE',  ( -9.499679989893815346, -7.184999792974224420, -0.07801928546529064701 ) ) ;
#170398=FACE_BOUND ( 'NONE', #145758, .T. ) ;
#170400=EDGE_LOOP ( 'NONE', ( #93788, #22335, #5546, #130358 ) ) ;
#170422=( GEOMETRIC_REPRESENTATION_CONTEXT ( 3 ) GLOBAL_UNCERTAINTY_ASSIGNED_CONTEXT ( ( #105648 ) ) GLOBAL_UNIT_ASSIGNED_CONTEXT ( ( #70788, #169386, #54572 ) ) REPRESENTATION_CONTEXT ( 'NONE', 'WORKASPACE' ) );
#170445=B_SPLINE_CURVE_WITH_KNOTS ( 'NONE', 3,
 ( #52251, #6678, #138852, #102069, #137785, #150834, #118378, #40278, #171327, #106388 ),
 .UNSPECIFIED., .F., .F.,
 ( 4, 2, 2, 2, 4 ),
 ( 0.000000000000000000, 0.0002334048330869039766, 0.0004668096661738078447, 0.0007002144992607117670, 0.0009336193323476156894 ),
 .UNSPECIFIED. ) ;
#170466=CARTESIAN_POINT ( 'NONE',  ( 10.99962150373186986, -9.999999999999879208, -0.09125116240082961627 ) ) ;
#170471=CARTESIAN_POINT ( 'NONE',  ( -2.361527856944989345E-15, -9.448428148670510396, -9.261795338153651969 ) ) ;
#170487=VERTEX_POINT ( 'NONE', #161985 ) ;
#170499=CARTESIAN_POINT ( 'NONE',  ( 0.000000000000000000, 15.50000000000019362, 0.000000000000000000 ) ) ;
#170516=FACE_OUTER_BOUND ( 'NONE', #167511, .T. ) ;
#170524=CARTESIAN_POINT ( 'NONE',  ( 7.720982897393565914, -6.307829212974243482, -7.834948825496931057 ) ) ;
#170549=CARTESIAN_POINT ( 'NONE',  ( 0.000000000000000000, -9.999999999999994671, 0.000000000000000000 ) ) ;
#170581=CARTESIAN_POINT ( 'NONE',  ( -10.99374989157288240, -6.893136995915043919, 0.3811408430856400575 ) ) ;
#170619=DIRECTION ( 'NONE',  ( 0.000000000000000000, 1.000000000000000000, 0.000000000000000000 ) ) ;
#170675=( BOUNDED_SURFACE ( )  B_SPLINE_SURFACE ( 3, 2, ( 
 ( #23870, #89977, #156027 ),
 ( #7617, #140878, #73701 ),
 ( #189582, #41229, #165613 ),
 ( #61721, #131053, #64904 ) ),
 .UNSPECIFIED., .F., .F., .T. ) 
 B_SPLINE_SURFACE_WITH_KNOTS ( ( 4, 4 ),
 ( 3, 3 ),
 ( 0.000000000000000000, 9.170893477921754312E-05 ),
 ( 0.000000000000000000, 1.000000000000000000 ),
 .UNSPECIFIED. ) 
 GEOMETRIC_REPRESENTATION_ITEM ( )  RATIONAL_B_SPLINE_SURFACE ( (
 ( 1.000000000000000000, 0.6787756258918323793, 1.000000000000000000),
 ( 1.000000000000000000, 0.6894756946172844181, 1.000000000000000000),
 ( 1.000000000000000000, 0.6998898451712581847, 1.000000000000000000),
 ( 1.000000000000000000, 0.7100530722070644840, 1.000000000000000000) ) ) 
 REPRESENTATION_ITEM ( '' )  SURFACE ( )  );
#170676=LINE ( 'NONE', #138199, #28730 ) ;
#170677=FACE_OUTER_BOUND ( 'NONE', #35761, .T. ) ;
#170704=ORIENTED_EDGE ( 'NONE', *, *, #7456, .F. ) ;
#170708=CARTESIAN_POINT ( 'NONE',  ( -2.020417662918760016, 3.956598013261175772, 11.36521191596583336 ) ) ;
#170721=B_SPLINE_CURVE_WITH_KNOTS ( 'NONE', 3,
 ( #72358, #204480, #156849, #188249, #39890, #106000, #157919, #108154 ),
 .UNSPECIFIED., .F., .F.,
 ( 4, 2, 2, 4 ),
 ( 1.734723475976789761E-18, 0.0004365159022975801891, 0.0006547738534463698771, 0.0008730318045951596193 ),
 .UNSPECIFIED. ) ;
#170749=ORIENTED_EDGE ( 'NONE', *, *, #135163, .T. ) ;
#170785=DIRECTION ( 'NONE',  ( -0.000000000000000000, -1.000000000000000000, -0.000000000000000000 ) ) ;
#170833=DIRECTION ( 'NONE',  ( -8.881784197001252323E-16, 0.000000000000000000, 1.000000000000000000 ) ) ;
#170841=EDGE_CURVE ( 'NONE', #193389, #94238, #47095, .T. ) ;
#170846=CARTESIAN_POINT ( 'NONE',  ( -10.91877484692252942, -9.999999999999991118, 0.1449562030364423548 ) ) ;
#170909=CARTESIAN_POINT ( 'NONE',  ( 1.409462824231155764E-15, 1.016282880930358123, -12.28865868783309878 ) ) ;
#170924=SURFACE_STYLE_USAGE ( .BOTH. , #188235 ) ;
#170931=( NAMED_UNIT ( * ) PLANE_ANGLE_UNIT ( ) SI_UNIT ( $, .RADIAN. ) );
#170938=CARTESIAN_POINT ( 'NONE',  ( 0.07999999999999327094, 7.849261790823902629, 9.579665964948873125 ) ) ;
#170946=DIRECTION ( 'NONE',  ( -1.224646799147343346E-16, 0.000000000000000000, -1.000000000000000000 ) ) ;
#170949=AXIS2_PLACEMENT_3D ( 'NONE', #55902, #203194, #3916 ) ;
#171017=CARTESIAN_POINT ( 'NONE',  ( -0.07933543236768950124, -9.910877263631634904, -9.499668725233682665 ) ) ;
#171032=CARTESIAN_POINT ( 'NONE',  ( -9.469892045836674654, -6.532648833121171172, 0.4294077647110563500 ) ) ;
#171035=EDGE_LOOP ( 'NONE', ( #136964, #100848 ) ) ;
#171064=CARTESIAN_POINT ( 'NONE',  ( -10.72111444838896155, -6.105866302529358691, 1.138412281109779656E-15 ) ) ;
#171065=CARTESIAN_POINT ( 'NONE',  ( 10.10176665042273392, 1.000000000000000888, 6.279211784079129721 ) ) ;
#171092=( NAMED_UNIT ( * ) PLANE_ANGLE_UNIT ( ) SI_UNIT ( $, .RADIAN. ) );
#171103=CARTESIAN_POINT ( 'NONE',  ( -10.91005274787796786, -6.893137084989842123, 0.4659925305415812957 ) ) ;
#171111=CIRCLE ( 'NONE', #22345, 10.24999999999998934 ) ;
#171132=ORIENTED_EDGE ( 'NONE', *, *, #15624, .F. ) ;
#171134=CARTESIAN_POINT ( 'NONE',  ( -7.451274665340259951, -7.616254850791390751, 6.794158526849257029 ) ) ;
#171142=FACE_OUTER_BOUND ( 'NONE', #203656, .T. ) ;
#171160=CIRCLE ( 'NONE', #95110, 10.91999999999999105 ) ;
#171169=CARTESIAN_POINT ( 'NONE',  ( 7.882977371601994854, -5.341768514962173420, -7.624693973552353121 ) ) ;
#171211=CARTESIAN_POINT ( 'NONE',  ( -7.873959529867724072, -5.295524846228480520, 7.681496476274701557 ) ) ;
#171226=CARTESIAN_POINT ( 'NONE',  ( 9.567202289542830584, -7.627132808484214266, -0.008219159353554262443 ) ) ;
#171237=DIRECTION ( 'NONE',  ( -0.000000000000000000, -1.000000000000000000, -0.000000000000000000 ) ) ;
#171243=ORIENTED_EDGE ( 'NONE', *, *, #156087, .F. ) ;
#171253=CARTESIAN_POINT ( 'NONE',  ( -7.768428355091604232, -6.306978362809940286, -7.788485247870016615 ) ) ;
#171311=CARTESIAN_POINT ( 'NONE',  ( -9.499700864329913230, -7.154544010627095219, -0.07538891330674860058 ) ) ;
#171327=CARTESIAN_POINT ( 'NONE',  ( -2.722740351562989813E-16, -7.550885189219943783, 9.573337995800487832 ) ) ;
#171331=ORIENTED_EDGE ( 'NONE', *, *, #113687, .F. ) ;
#171360=CARTESIAN_POINT ( 'NONE',  ( 7.462104991928526054, -5.166862915010159263, 8.081892667527535323 ) ) ;
#171362=CARTESIAN_POINT ( 'NONE',  ( 10.91944002402979130, -9.900000000000005684, -0.1105873483556608222 ) ) ;
#171365=EDGE_LOOP ( 'NONE', ( #136158, #135527, #52491, #62872 ) ) ;
#171368=ORIENTED_EDGE ( 'NONE', *, *, #56480, .T. ) ;
#171376=CARTESIAN_POINT ( 'NONE',  ( -0.4294077647110545737, -6.532648833121157850, -9.469892045836658667 ) ) ;
#171458=CARTESIAN_POINT ( 'NONE',  ( 11.00006988736402036, -9.999999999999994671, -0.09199170129443705324 ) ) ;
#171485=FILL_AREA_STYLE_COLOUR ( '', #13601 ) ;
#171486=FACE_OUTER_BOUND ( 'NONE', #152359, .T. ) ;
#171493=ORIENTED_EDGE ( 'NONE', *, *, #110609, .F. ) ;
#171516=SURFACE_SIDE_STYLE ('',( #7938 ) ) ;
#171517=EDGE_CURVE ( 'NONE', #51191, #72609, #28136, .T. ) ;
#171556=ORIENTED_EDGE ( 'NONE', *, *, #132492, .F. ) ;
#171572=CARTESIAN_POINT ( 'NONE',  ( 6.663994888585881959, -7.154544010627095219, -6.770610912236887380 ) ) ;
#171580=CARTESIAN_POINT ( 'NONE',  ( 7.446209719563361418, -5.223431457505083308, 8.064677165291199046 ) ) ;
#171584=CARTESIAN_POINT ( 'NONE',  ( -6.524021554744627416, -6.747656629766783709, -6.895452369244214452 ) ) ;
#171603=CARTESIAN_POINT ( 'NONE',  ( 0.09924927195300653482, -9.920000000000094076, 10.99955234463956089 ) ) ;
#171706=CARTESIAN_POINT ( 'NONE',  ( -0.09196683552162310260, -9.918146503183461249, -10.99961570984661563 ) ) ;
#171744=CARTESIAN_POINT ( 'NONE',  ( -9.499610831742323569, -9.904389604292740401, 0.08598863555141569859 ) ) ;
#171751=B_SPLINE_CURVE_WITH_KNOTS ( 'NONE', 3,
 ( #106099, #101779, #172121, #205662, #23715, #155869, #167848, #19447 ),
 .UNSPECIFIED., .F., .F.,
 ( 4, 2, 2, 4 ),
 ( 6.505213034912872530E-19, 0.0002224730689913817223, 0.0004449461379827644204, 0.0008898922759655299251 ),
 .UNSPECIFIED. ) ;
#171755=AXIS2_PLACEMENT_3D ( 'NONE', #49694, #181810, #148277 ) ;
#171768=CARTESIAN_POINT ( 'NONE',  ( 0.000000000000000000, -6.893137084989842123, 0.000000000000000000 ) ) ;
#171799=FILL_AREA_STYLE_COLOUR ( '', #36692 ) ;
#171819=SURFACE_STYLE_FILL_AREA ( #122091 ) ;
#171834=ORIENTED_EDGE ( 'NONE', *, *, #110968, .F. ) ;
#171844=FACE_OUTER_BOUND ( 'NONE', #111930, .T. ) ;
#171851=DIRECTION ( 'NONE',  ( 0.000000000000000000, 1.000000000000000000, 0.000000000000000000 ) ) ;
#171878=ORIENTED_EDGE ( 'NONE', *, *, #132056, .T. ) ;
#171933=COLOUR_RGB ( '', 0.72549020, 0.75294118, 0.79215686) ;
#171998=CARTESIAN_POINT ( 'NONE',  ( -9.492545994383801755, -8.199730735665985648, 0.3846410972798168237 ) ) ;
#172000=CARTESIAN_POINT ( 'NONE',  ( -0.4330588727801884530, -9.006862915010128035, 9.570206894979145673 ) ) ;
#172003=VERTEX_POINT ( 'NONE', #123340 ) ;
#172015=FACE_OUTER_BOUND ( 'NONE', #40243, .T. ) ;
#172023=CARTESIAN_POINT ( 'NONE',  ( -0.08000000000000714873, -5.907420853759270507, 10.99970695577494872 ) ) ;
#172036=CARTESIAN_POINT ( 'NONE',  ( -0.2834499523633308704, -6.554910290221268809, -9.477100695693451371 ) ) ;
#172045=FILL_AREA_STYLE ('',( #22562 ) ) ;
#172048=CARTESIAN_POINT ( 'NONE',  ( -0.4382560683119281486, -7.700000000000008171, 10.99126615174920474 ) ) ;
#172061=CIRCLE ( 'NONE', #185789, 0.07999999999999948819 ) ;
#172075=ORIENTED_EDGE ( 'NONE', *, *, #33910, .T. ) ;
#172104=ORIENTED_EDGE ( 'NONE', *, *, #63903, .F. ) ;
#172114=CARTESIAN_POINT ( 'NONE',  ( -7.346809171966454777, -6.836568542494980250, -8.002408263930250953 ) ) ;
#172121=CARTESIAN_POINT ( 'NONE',  ( 10.96384327792182134, -7.754568858751050620, -0.4817895937885937618 ) ) ;
#172130=CARTESIAN_POINT ( 'NONE',  ( 0.000000000000000000, -6.836568542494925182, 0.000000000000000000 ) ) ;
#172149=CARTESIAN_POINT ( 'NONE',  ( 0.000000000000000000, -2.000000000000001776, 0.000000000000000000 ) ) ;
#172156=DIRECTION ( 'NONE',  ( -0.000000000000000000, -1.000000000000000000, -0.000000000000000000 ) ) ;
#172181=VERTEX_POINT ( 'NONE', #211939 ) ;
#172189=CARTESIAN_POINT ( 'NONE',  ( -10.96499746917716500, -5.350147675656139690, 0.1749484593404612431 ) ) ;
#172200=EDGE_CURVE ( 'NONE', #201551, #49868, #152739, .T. ) ;
#172234=ORIENTED_EDGE ( 'NONE', *, *, #186461, .F. ) ;
#172259=DIRECTION ( 'NONE',  ( 0.7366372490351829061, 1.218064704987765655E-12, -0.6762880771785629852 ) ) ;
#172262=EDGE_LOOP ( 'NONE', ( #65898, #26800, #132855, #208871 ) ) ;
#172334=CARTESIAN_POINT ( 'NONE',  ( -7.362820735711497200, -5.796536394785085200, 7.362820735712229059 ) ) ;
#172373=AXIS2_PLACEMENT_3D ( 'NONE', #131920, #135105, #117833 ) ;
#172374=DIRECTION ( 'NONE',  ( 0.000000000000000000, 0.000000000000000000, 1.000000000000000000 ) ) ;
#172393=DIRECTION ( 'NONE',  ( 0.000000000000000000, 1.000000000000000000, 0.000000000000000000 ) ) ;
#172411=CARTESIAN_POINT ( 'NONE',  ( 0.007565906569757733027, -9.598697202504085979, -9.591786056756832934 ) ) ;
#172415=EDGE_LOOP ( 'NONE', ( #154933, #118875, #75218, #83523 ) ) ;
#172428=COLOUR_RGB ( '', 0.72549020, 0.75294118, 0.79215686) ;
#172445=CARTESIAN_POINT ( 'NONE',  ( 7.004500933659043582, -6.920331743269733771, -7.004500933659070228 ) ) ;
#172478=ORIENTED_EDGE ( 'NONE', *, *, #44939, .F. ) ;
#172492=ADVANCED_FACE ( 'NONE', ( #51596 ), #96645, .T. ) ;
#172604=ADVANCED_FACE ( 'NONE', ( #133942 ), #183499, .F. ) ;
#172624=DIRECTION ( 'NONE',  ( 0.000000000000000000, 1.000000000000000000, 0.000000000000000000 ) ) ;
#172626=DIRECTION ( 'NONE',  ( 0.000000000000000000, 1.000000000000000000, 0.000000000000000000 ) ) ;
#172710=AXIS2_PLACEMENT_3D ( 'NONE', #146998, #98234, #15877 ) ;
#172730=MECHANICAL_DESIGN_GEOMETRIC_PRESENTATION_REPRESENTATION('',(#186480),#200371);
#172731=SURFACE_STYLE_FILL_AREA ( #86132 ) ;
#172739=CARTESIAN_POINT ( 'NONE',  ( -0.07933194154489606187, -9.900000000000005684, -9.499668754385620417 ) ) ;
#172742=SURFACE_SIDE_STYLE ('',( #175946 ) ) ;
#172766=B_SPLINE_CURVE_WITH_KNOTS ( 'NONE', 3,
 ( #148777, #208174, #89130, #5685, #121698, #137878, #156260 ),
 .UNSPECIFIED., .F., .F.,
 ( 4, 3, 4 ),
 ( 0.0001135037246156244756, 0.0006171834326598004457, 0.002007692286214975488 ),
 .UNSPECIFIED. ) ;
#172778=SURFACE_STYLE_FILL_AREA ( #108902 ) ;
#172845=VECTOR ( 'NONE', #13021, 1000.000000000000227 ) ;
#172856=DIRECTION ( 'NONE',  ( -0.9998476951563912696, -0.000000000000000000, 0.01745240643728004568 ) ) ;
#172885=CARTESIAN_POINT ( 'NONE',  ( 9.096228393767193054, 0.9691415390508323346, 7.669416753559205269 ) ) ;
#172906=EDGE_CURVE ( 'NONE', #206352, #40383, #20857, .T. ) ;
#172940=ORIENTED_EDGE ( 'NONE', *, *, #148514, .T. ) ;
#172942=CARTESIAN_POINT ( 'NONE',  ( -0.3175553531547188890, 3.956598013261175772, 11.53924059509144051 ) ) ;
#172945=( NAMED_UNIT ( * ) SI_UNIT ( $, .STERADIAN. ) SOLID_ANGLE_UNIT ( ) );
#172976=VERTEX_POINT ( 'NONE', #85889 ) ;
#172990=DIRECTION ( 'NONE',  ( 0.000000000000000000, 0.000000000000000000, 1.000000000000000000 ) ) ;
#173038=ORIENTED_EDGE ( 'NONE', *, *, #29437, .F. ) ;
#173047=EDGE_CURVE ( 'NONE', #168888, #71781, #134549, .T. ) ;
#173050=VECTOR ( 'NONE', #164147, 1000.000000000000000 ) ;
#173063=EDGE_LOOP ( 'NONE', ( #64630, #27020, #23134, #141943 ) ) ;
#173066=CARTESIAN_POINT ( 'NONE',  ( -1.668847547942637130E-13, 1.972237431424126441, -11.78526707783712624 ) ) ;
#173067=ORIENTED_EDGE ( 'NONE', *, *, #110609, .T. ) ;
#173077=CARTESIAN_POINT ( 'NONE',  ( -10.99526901688165381, -7.794005300192725194, 0.3296348669024621314 ) ) ;
#173083=CARTESIAN_POINT ( 'NONE',  ( 10.91819195543074450, -9.943514287384804362, -0.1813054759508098968 ) ) ;
#173085=B_SPLINE_CURVE_WITH_KNOTS ( 'NONE', 3,
 ( #141652, #175196, #156808, #8395, #190340, #25711 ),
 .UNSPECIFIED., .F., .F.,
 ( 4, 2, 4 ),
 ( 0.000000000000000000, 0.0002955107118804045814, 0.0005910214237608091628 ),
 .UNSPECIFIED. ) ;
#173103=B_SPLINE_CURVE_WITH_KNOTS ( 'NONE', 3,
 ( #44093, #124349, #159960, #93920 ),
 .UNSPECIFIED., .F., .F.,
 ( 4, 4 ),
 ( 8.674676106452419934E-19, 9.170750103568725835E-05 ),
 .UNSPECIFIED. ) ;
#173131=CARTESIAN_POINT ( 'NONE',  ( -0.4373225248172924462, -7.723431457505077979, 10.96785329849814161 ) ) ;
#173146=CARTESIAN_POINT ( 'NONE',  ( 8.917737905728806425, 3.447199233515649386, 8.029567276306217138 ) ) ;
#173163=EDGE_CURVE ( 'NONE', #165149, #149524, #132076, .T. ) ;
#173197=AXIS2_PLACEMENT_3D ( 'NONE', #30733, #95747, #181223 ) ;
#173200=CARTESIAN_POINT ( 'NONE',  ( 0.01315889736931378021, -9.583523248314012477, -9.500441148488286913 ) ) ;
#173210=SURFACE_SIDE_STYLE ('',( #44269 ) ) ;
#173232=ORIENTED_EDGE ( 'NONE', *, *, #46509, .F. ) ;
#173287=DIRECTION ( 'NONE',  ( 0.000000000000000000, -1.000000000000000000, 0.000000000000000000 ) ) ;
#173344=ORIENTED_EDGE ( 'NONE', *, *, #157926, .F. ) ;
#173348=ORIENTED_EDGE ( 'NONE', *, *, #35731, .F. ) ;
#173359=CARTESIAN_POINT ( 'NONE',  ( -9.030096778091493803, 1.000000000000000888, -7.742171412064445590 ) ) ;
#173415=FACE_OUTER_BOUND ( 'NONE', #126622, .T. ) ;
#173425=DIRECTION ( 'NONE',  ( -0.9989735196462991018, -4.834648123959315881E-16, 0.04529798058948755063 ) ) ;
#173433=CARTESIAN_POINT ( 'NONE',  ( 9.499606442108964544, -9.746166700193986898, -0.08647222121513538362 ) ) ;
#173440=CARTESIAN_POINT ( 'NONE',  ( 0.07999999999999327094, -9.900000000000005684, 9.579665964948873125 ) ) ;
#173455=DIRECTION ( 'NONE',  ( 0.000000000000000000, 0.000000000000000000, 1.000000000000000000 ) ) ;
#173463=CARTESIAN_POINT ( 'NONE',  ( -10.99861980075107759, -8.407420853759271395, 0.1919816227428516597 ) ) ;
#173465=VERTEX_POINT ( 'NONE', #143223 ) ;
#173466=EDGE_CURVE ( 'NONE', #1301, #107467, #204663, .T. ) ;
#173477=CARTESIAN_POINT ( 'NONE',  ( -8.917737905728749581, 4.000000000000003553, -8.029567276306266876 ) ) ;
#173499=CARTESIAN_POINT ( 'NONE',  ( -7.828177403543865154, -5.742104877864245616, -7.727873494160012235 ) ) ;
#173525=ORIENTED_EDGE ( 'NONE', *, *, #82593, .F. ) ;
#173599=CARTESIAN_POINT ( 'NONE',  ( -10.95855051086948606, -7.723431457505092190, 0.6286713519884027379 ) ) ;
#173602=ORIENTED_EDGE ( 'NONE', *, *, #100462, .T. ) ;
#173604=CARTESIAN_POINT ( 'NONE',  ( 0.07933191752141914577, -7.643695121331862019, -9.499668754586256370 ) ) ;
#173661=CARTESIAN_POINT ( 'NONE',  ( 0.000000000000000000, 4.000000000000003553, 0.000000000000000000 ) ) ;
#173715=ORIENTED_EDGE ( 'NONE', *, *, #130897, .T. ) ;
#173740=DIRECTION ( 'NONE',  ( -0.6724985119639490527, 0.7071067811865536790, 0.2185080122244163481 ) ) ;
#173753=CARTESIAN_POINT ( 'NONE',  ( 7.583532603600732003, -5.197284395437371529, 7.968353659517134702 ) ) ;
#173755=DIRECTION ( 'NONE',  ( 0.000000000000000000, -1.000000000000000000, 0.000000000000000000 ) ) ;
#173765=DIRECTION ( 'NONE',  ( 0.000000000000000000, 0.000000000000000000, 1.000000000000000000 ) ) ;
#173791=CYLINDRICAL_SURFACE ( 'NONE', #147454, 0.08000000000000020983 ) ;
#173802=CARTESIAN_POINT ( 'NONE',  ( -2.494940289813118994, 4.000000000000003553, 11.73777120880565583 ) ) ;
#173876=EDGE_LOOP ( 'NONE', ( #9978, #119296, #46908, #137110 ) ) ;
#173932=AXIS2_PLACEMENT_3D ( 'NONE', #188320, #104969, #153707 ) ;
#173938=LINE ( 'NONE', #106826, #191130 ) ;
#173956=ADVANCED_FACE ( 'NONE', ( #5240 ), #119092, .F. ) ;
#173969=ORIENTED_EDGE ( 'NONE', *, *, #6898, .T. ) ;
#173986=CARTESIAN_POINT ( 'NONE',  ( 2.157015650737173384, 3.934209603697786495, -11.36298392073394226 ) ) ;
#174008=ORIENTED_EDGE ( 'NONE', *, *, #94862, .T. ) ;
#174047=CARTESIAN_POINT ( 'NONE',  ( -7.100579091573050228, -6.583980363594990948, 6.484567079770452658 ) ) ;
#174059=CARTESIAN_POINT ( 'NONE',  ( -6.979380938965681125, -8.233137084989706977, 6.445605026751805688 ) ) ;
#174069=EDGE_CURVE ( 'NONE', #205917, #127875, #71316, .T. ) ;
#174078=VECTOR ( 'NONE', #20937, 1000.000000000000000 ) ;
#174105=CARTESIAN_POINT ( 'NONE',  ( 7.769310276573728302, -5.221243112839674794, 7.769310276573704321 ) ) ;
#174125=UNCERTAINTY_MEASURE_WITH_UNIT (LENGTH_MEASURE( 1.000000000000000082E-05 ), #67169, 'distance_accuracy_value', 'NONE');
#174157=ORIENTED_EDGE ( 'NONE', *, *, #154365, .T. ) ;
#174173=ORIENTED_EDGE ( 'NONE', *, *, #75043, .T. ) ;
#174181=CYLINDRICAL_SURFACE ( 'NONE', #135866, 0.08000000000000020983 ) ;
#174200=DIRECTION ( 'NONE',  ( -0.04888523518676889112, 8.339466111204228823E-16, -0.9988044021632737079 ) ) ;
#174224=ORIENTED_EDGE ( 'NONE', *, *, #207104, .T. ) ;
#174236=CIRCLE ( 'NONE', #115508, 11.29999999999998828 ) ;
#174242=VECTOR ( 'NONE', #34882, 1000.000000000000000 ) ;
#174249=DIRECTION ( 'NONE',  ( 0.000000000000000000, 0.000000000000000000, 1.000000000000000000 ) ) ;
#174267=ORIENTED_EDGE ( 'NONE', *, *, #100809, .T. ) ;
#174271=DIRECTION ( 'NONE',  ( 0.7071067811865462405, 0.000000000000000000, -0.7071067811865489050 ) ) ;
#174288=CARTESIAN_POINT ( 'NONE',  ( -6.984891963202824350, -8.199734048663005481, 6.439526774796434871 ) ) ;
#174311=DIRECTION ( 'NONE',  ( 0.000000000000000000, 1.000000000000000000, 0.000000000000000000 ) ) ;
#174320=CARTESIAN_POINT ( 'NONE',  ( 1.637338291174485510E-15, -6.530144695498204754, 11.00000000000000178 ) ) ;
#174324=CARTESIAN_POINT ( 'NONE',  ( -11.07693626658230990, 1.970899860167826700, 4.005980692924094200 ) ) ;
#174334=CARTESIAN_POINT ( 'NONE',  ( -10.97113184882213766, -5.223163831703878657, 0.3618152180564682685 ) ) ;
#174366=CARTESIAN_POINT ( 'NONE',  ( 7.735357998705605809, -5.759585062615364848, -7.724608556409205740 ) ) ;
#174369=DIRECTION ( 'NONE',  ( -0.6783731810844091381, 3.929830605827845711E-15, -0.7347175152297782397 ) ) ;
#174410=VERTEX_POINT ( 'NONE', #1771 ) ;
#174496=DIRECTION ( 'NONE',  ( -0.01745240643728004568, 0.000000000000000000, -0.9998476951563912696 ) ) ;
#174524=( BOUNDED_SURFACE ( )  B_SPLINE_SURFACE ( 3, 2, ( 
 ( #188818, #22012, #122857 ),
 ( #74003, #205047, #3629 ),
 ( #70766, #186673, #137948 ),
 ( #38300, #154192, #121771 ) ),
 .UNSPECIFIED., .F., .F., .F. ) 
 B_SPLINE_SURFACE_WITH_KNOTS ( ( 4, 4 ),
 ( 3, 3 ),
 ( 0.000000000000000000, 9.170893476616523974E-05 ),
 ( 0.000000000000000000, 1.000000000000000000 ),
 .UNSPECIFIED. ) 
 GEOMETRIC_REPRESENTATION_ITEM ( )  RATIONAL_B_SPLINE_SURFACE ( (
 ( 1.000000000000000000, 0.7100530722026879848, 1.000000000000000000),
 ( 1.000000000000000000, 0.6998898451682321609, 1.000000000000000000),
 ( 1.000000000000000000, 0.6894756946157196698, 1.000000000000000000),
 ( 1.000000000000000000, 0.6787756258917869712, 1.000000000000000000) ) ) 
 REPRESENTATION_ITEM ( '' )  SURFACE ( )  );
#174555=CARTESIAN_POINT ( 'NONE',  ( -0.4382560683119304801, -7.666862915010147717, 10.99126615174920119 ) ) ;
#174588=CARTESIAN_POINT ( 'NONE',  ( -2.093037498677872144, 1.000000000000000888, 11.70868840297834446 ) ) ;
#174595=CARTESIAN_POINT ( 'NONE',  ( -7.518896314322850216, -5.199789852011974745, -8.029456579251602832 ) ) ;
#174717=( NAMED_UNIT ( * ) PLANE_ANGLE_UNIT ( ) SI_UNIT ( $, .RADIAN. ) );
#174810=ORIENTED_EDGE ( 'NONE', *, *, #64219, .T. ) ;
#174819=CARTESIAN_POINT ( 'NONE',  ( 7.573156686838095730, -5.230039540835552891, 7.978162878861390084 ) ) ;
#174846=CARTESIAN_POINT ( 'NONE',  ( -10.91944002402978775, -9.900000000000005684, 0.1905873483556694836 ) ) ;
#174907=ADVANCED_FACE ( 'NONE', ( #31561 ), #132222, .T. ) ;
#174913=ADVANCED_FACE ( 'NONE', ( #165813 ), #84554, .F. ) ;
#174925=FACE_OUTER_BOUND ( 'NONE', #68, .T. ) ;
#175021=FACE_OUTER_BOUND ( 'NONE', #41161, .T. ) ;
#175035=CARTESIAN_POINT ( 'NONE',  ( -10.67870335800436798, -6.148216694138041838, 1.725267604293023217E-15 ) ) ;
#175057=ORIENTED_EDGE ( 'NONE', *, *, #78925, .F. ) ;
#175072=CARTESIAN_POINT ( 'NONE',  ( 9.590330253158084517, -9.597646708343965827, -0.1673998372498815279 ) ) ;
#175105=CARTESIAN_POINT ( 'NONE',  ( 9.183873789516525221, -7.868711957286002701, 9.269928574751062911E-15 ) ) ;
#175139=VERTEX_POINT ( 'NONE', #117117 ) ;
#175161=EDGE_CURVE ( 'NONE', #190182, #164527, #184117, .T. ) ;
#175188=FACE_OUTER_BOUND ( 'NONE', #194233, .T. ) ;
#175196=CARTESIAN_POINT ( 'NONE',  ( -0.3388969742604198143, -7.666862915010146828, 10.99522790877599654 ) ) ;
#175200=CARTESIAN_POINT ( 'NONE',  ( -6.901817412891860570, -6.554751173179683477, 6.500815856195042208 ) ) ;
#175220=CYLINDRICAL_SURFACE ( 'NONE', #75711, 11.49999999999998934 ) ;
#175231=CARTESIAN_POINT ( 'NONE',  ( -9.765991159989196646, -7.287292132423887736, 1.138412281109779656E-15 ) ) ;
#175257=PRESENTATION_STYLE_ASSIGNMENT (( #125505 ) ) ;
#175281=EDGE_CURVE ( 'NONE', #108269, #86684, #139737, .T. ) ;
#175339=CARTESIAN_POINT ( 'NONE',  ( 0.000000000000000000, 4.000000000000003553, 0.000000000000000000 ) ) ;
#175348=CARTESIAN_POINT ( 'NONE',  ( 0.09916492693110359746, -9.919999999999998153, 9.499482423651659957 ) ) ;
#175381=CARTESIAN_POINT ( 'NONE',  ( -11.57407876878716557, 2.018041202054113636, 3.760646157730112016 ) ) ;
#175401=AXIS2_PLACEMENT_3D ( 'NONE', #17936, #84022, #185776 ) ;
#175472=ORIENTED_EDGE ( 'NONE', *, *, #93956, .F. ) ;
#175475=CIRCLE ( 'NONE', #12936, 0.08000000000000020983 ) ;
#175527=CARTESIAN_POINT ( 'NONE',  ( 0.07302493934787820939, 1.405922845961229184, -11.99988463978223407 ) ) ;
#175540=CARTESIAN_POINT ( 'NONE',  ( 10.25773349932952350, -6.796015482748906322, 1.760695953681369627E-15 ) ) ;
#175543=CARTESIAN_POINT ( 'NONE',  ( 7.728718841140392648, -6.124285369217659536, 7.728718841140364226 ) ) ;
#175575=CARTESIAN_POINT ( 'NONE',  ( 7.037870247915987143, -8.199999999999986855, -6.381095703207948944 ) ) ;
#175580=ORIENTED_EDGE ( 'NONE', *, *, #115776, .T. ) ;
#175582=VERTEX_POINT ( 'NONE', #85620 ) ;
#175586=CARTESIAN_POINT ( 'NONE',  ( -10.99943592145024240, -8.241816521215563185, 0.1113975309873064257 ) ) ;
#175594=CIRCLE ( 'NONE', #182503, 0.08000000000000001554 ) ;
#175600=EDGE_CURVE ( 'NONE', #65129, #201530, #69344, .T. ) ;
#175621=CARTESIAN_POINT ( 'NONE',  ( -7.462104991928524278, -5.166862915010159263, -8.081892667527526442 ) ) ;
#175718=EDGE_CURVE ( 'NONE', #57699, #200355, #23464, .T. ) ;
#175780=AXIS2_PLACEMENT_3D ( 'NONE', #150543, #211396, #66042 ) ;
#175802=ORIENTED_EDGE ( 'NONE', *, *, #180630, .T. ) ;
#175828=DIRECTION ( 'NONE',  ( 0.000000000000000000, 1.000000000000000000, 0.000000000000000000 ) ) ;
#175864=CARTESIAN_POINT ( 'NONE',  ( 10.38819714233671121, 3.487142912321096855, 5.997628416522882588 ) ) ;
#175874=CARTESIAN_POINT ( 'NONE',  ( 0.000000000000000000, -2.079999999999998295, 0.000000000000000000 ) ) ;
#175946=SURFACE_STYLE_FILL_AREA ( #209470 ) ;
#176034=VECTOR ( 'NONE', #185724, 1000.000000000000000 ) ;
#176113=EDGE_LOOP ( 'NONE', ( #161460, #38991, #150283, #75158 ) ) ;
#176128=CARTESIAN_POINT ( 'NONE',  ( -0.01400375819625959001, -6.304807775344903220, -11.00039779441144461 ) ) ;
#176145=ADVANCED_FACE ( 'NONE', ( #187024 ), #14591, .T. ) ;
#176161=ORIENTED_EDGE ( 'NONE', *, *, #124205, .T. ) ;
#176191=CARTESIAN_POINT ( 'NONE',  ( -7.834948825496938163, -5.907420853759296264, -7.720982897393569466 ) ) ;
#176274=EDGE_LOOP ( 'NONE', ( #26247, #138709, #28934, #29290 ) ) ;
#176296=VECTOR ( 'NONE', #137509, 1000.000000000000000 ) ;
#176315=CARTESIAN_POINT ( 'NONE',  ( -9.499606441938682977, -9.580980486002397711, 0.08647223992180037844 ) ) ;
#176359=EDGE_CURVE ( 'NONE', #43490, #114100, #156627, .T. ) ;
#176369=CIRCLE ( 'NONE', #20645, 0.08000000000000009881 ) ;
#176381=DIRECTION ( 'NONE',  ( -0.000000000000000000, -1.000000000000000000, -0.000000000000000000 ) ) ;
#176382=DIRECTION ( 'NONE',  ( 1.000000000000000000, -0.000000000000000000, 1.224646799147353207E-16 ) ) ;
#176398=FACE_OUTER_BOUND ( 'NONE', #130425, .T. ) ;
#176419=CARTESIAN_POINT ( 'NONE',  ( -0.01154776750710303362, -8.267087321559111857, -11.00021059652968347 ) ) ;
#176437=CARTESIAN_POINT ( 'NONE',  ( -11.20845505065987346, 1.972237431424385790, 3.641847810297710097 ) ) ;
#176440=ORIENTED_EDGE ( 'NONE', *, *, #102432, .F. ) ;
#176489=CARTESIAN_POINT ( 'NONE',  ( -0.03132844593999471045, -5.600264386820912321, -10.94526678918446727 ) ) ;
#176516=CARTESIAN_POINT ( 'NONE',  ( 0.1288460037565949678, -8.008893676011954454, 9.499262961676864236 ) ) ;
#176569=CARTESIAN_POINT ( 'NONE',  ( 8.917737905728806425, 3.499999999999989342, 8.029567276306217138 ) ) ;
#176600=DIRECTION ( 'NONE',  ( -0.000000000000000000, -1.000000000000000000, -0.000000000000000000 ) ) ;
#176622=EDGE_CURVE ( 'NONE', #133392, #45686, #52856, .T. ) ;
#176630=CARTESIAN_POINT ( 'NONE',  ( 7.721398836998395687, -6.134628647623487474, 7.721398836998373483 ) ) ;
#176643=SURFACE_SIDE_STYLE ('',( #60747 ) ) ;
#176648=CARTESIAN_POINT ( 'NONE',  ( -7.777967379493323286, -5.907420853759296264, -7.664830294503433450 ) ) ;
#176651=SURFACE_STYLE_FILL_AREA ( #129054 ) ;
#176664=CARTESIAN_POINT ( 'NONE',  ( -0.09280742163705632541, -9.178267117872113801, 9.499822780340156925 ) ) ;
#176701=DIRECTION ( 'NONE',  ( 0.000000000000000000, -1.000000000000000000, 0.000000000000000000 ) ) ;
#176702=CARTESIAN_POINT ( 'NONE',  ( -10.96785329849812562, -5.223431457505089526, 0.4373225248172959434 ) ) ;
#176767=UNCERTAINTY_MEASURE_WITH_UNIT (LENGTH_MEASURE( 1.000000000000000082E-05 ), #107834, 'distance_accuracy_value', 'NONE');
#176780=VERTEX_POINT ( 'NONE', #199549 ) ;
#176790=CARTESIAN_POINT ( 'NONE',  ( -10.99126615174920651, -5.166862915010145052, 0.4382560683119391398 ) ) ;
#176800=VERTEX_POINT ( 'NONE', #169199 ) ;
#176820=CARTESIAN_POINT ( 'NONE',  ( 6.776370306708061619, -7.161464053357560644, 6.781144757626056396 ) ) ;
#176827=CARTESIAN_POINT ( 'NONE',  ( -7.548736457559128255, -7.034525084977406806, 7.548736457552015722 ) ) ;
#176833=( NAMED_UNIT ( * ) SI_UNIT ( $, .STERADIAN. ) SOLID_ANGLE_UNIT ( ) );
#176838=CARTESIAN_POINT ( 'NONE',  ( 8.280982047128212287, -6.442483420143131134, -7.626074736120320274 ) ) ;
#176851=FILL_AREA_STYLE_COLOUR ( '', #189023 ) ;
#176853=CIRCLE ( 'NONE', #138830, 0.07999999999999951594 ) ;
#176854=CARTESIAN_POINT ( 'NONE',  ( -1.734723475976807094E-15, -9.900000000000005684, -10.91970695577494332 ) ) ;
#176860=B_SPLINE_CURVE_WITH_KNOTS ( 'NONE', 3,
 ( #48530, #129852, #193690, #32268 ),
 .UNSPECIFIED., .F., .F.,
 ( 4, 4 ),
 ( 0.0005910214237608091628, 0.001001414237305831186 ),
 .UNSPECIFIED. ) ;
#176863=CARTESIAN_POINT ( 'NONE',  ( 7.657759090810039915, -5.412329794880678335, 7.842350841322885735 ) ) ;
#176865=SURFACE_STYLE_USAGE ( .BOTH. , #193102 ) ;
#176887=CARTESIAN_POINT ( 'NONE',  ( 0.4382560683119269829, -5.166862915010145052, 10.99126615174920474 ) ) ;
#176888=ORIENTED_EDGE ( 'NONE', *, *, #2389, .F. ) ;
#176922=CARTESIAN_POINT ( 'NONE',  ( 6.999862025036637014, -6.532648833121176501, -6.392587740394701790 ) ) ;
#176933=AXIS2_PLACEMENT_3D ( 'NONE', #55701, #6925, #8006 ) ;
#176973=LINE ( 'NONE', #212647, #148908 ) ;
#177065=EDGE_CURVE ( 'NONE', #176800, #144861, #177342, .T. ) ;
#177125=( NAMED_UNIT ( * ) PLANE_ANGLE_UNIT ( ) SI_UNIT ( $, .RADIAN. ) );
#177138=EDGE_CURVE ( 'NONE', #73749, #123257, #184269, .T. ) ;
#177165=DIRECTION ( 'NONE',  ( -0.008295560218253903231, 0.000000000000000000, -0.9999655912483516040 ) ) ;
#177184=CARTESIAN_POINT ( 'NONE',  ( -0.4694063952341900881, -6.893137084989856334, -10.98997987423602751 ) ) ;
#177201=CARTESIAN_POINT ( 'NONE',  ( -7.462104991928524278, -5.166862915010159263, -8.081892667527526442 ) ) ;
#177241=AXIS2_PLACEMENT_3D ( 'NONE', #171768, #157670, #191201 ) ;
#177289=VECTOR ( 'NONE', #65012, 1000.000000000000000 ) ;
#177334=ORIENTED_EDGE ( 'NONE', *, *, #80448, .T. ) ;
#177342=CIRCLE ( 'NONE', #194642, 0.07999999999999951594 ) ;
#177350=CARTESIAN_POINT ( 'NONE',  ( -10.08385610902500140, -7.605490242282780144, 0.4645879755154607160 ) ) ;
#177427=ORIENTED_EDGE ( 'NONE', *, *, #207501, .F. ) ;
#177439=CARTESIAN_POINT ( 'NONE',  ( 9.498564853506497485, -8.073984524010468178, -0.1796516426515351594 ) ) ;
#177443=DIRECTION ( 'NONE',  ( 0.000000000000000000, 1.000000000000000000, 0.000000000000000000 ) ) ;
#177445=CARTESIAN_POINT ( 'NONE',  ( 1.337314304668908615E-15, -2.079999999999998295, -10.91999999999999105 ) ) ;
#177447=CARTESIAN_POINT ( 'NONE',  ( -0.3869736770896817224, 1.794419290072776896, 11.79366332131313300 ) ) ;
#177488=DIRECTION ( 'NONE',  ( 0.000000000000000000, 0.000000000000000000, 1.000000000000000000 ) ) ;
#177507=ORIENTED_EDGE ( 'NONE', *, *, #38304, .T. ) ;
#177536=CARTESIAN_POINT ( 'NONE',  ( 0.4642244361878632430, -7.321523296574938833, 10.36809559534897929 ) ) ;
#177551=DIRECTION ( 'NONE',  ( 0.000000000000000000, 1.000000000000000000, 0.000000000000000000 ) ) ;
#177560=CARTESIAN_POINT ( 'NONE',  ( -8.966186108929056431, 2.441452740530747789, -7.552575952455633512 ) ) ;
#177574=CARTESIAN_POINT ( 'NONE',  ( -1.423015351387224570E-15, 0.9706168436483886275, 11.90408086427858336 ) ) ;
#177589=CARTESIAN_POINT ( 'NONE',  ( -3.686287386450715076E-15, -7.473374494045017968, 9.579665964948883783 ) ) ;
#177671=DIRECTION ( 'NONE',  ( 1.224646799147355426E-16, 0.000000000000000000, -1.000000000000000000 ) ) ;
#177703=ORIENTED_EDGE ( 'NONE', *, *, #28884, .F. ) ;
#177723=VECTOR ( 'NONE', #68856, 1000.000000000000000 ) ;
#177744=CARTESIAN_POINT ( 'NONE',  ( -9.606148981167596190, -6.583980363595129504, 0.4355862708379978354 ) ) ;
#177750=CARTESIAN_POINT ( 'NONE',  ( 10.90688615205259104, -6.291672674598550508, 1.452407135538879159E-15 ) ) ;
#177776=CARTESIAN_POINT ( 'NONE',  ( -7.462104991928527831, -5.200000000000006395, -8.081892667527538876 ) ) ;
#177809=CARTESIAN_POINT ( 'NONE',  ( 6.505896022970779846, -8.148356111791681400, 6.958662999125761139 ) ) ;
#177831=CARTESIAN_POINT ( 'NONE',  ( 7.055228938194279209, -8.176568542494891290, -6.396834479292358822 ) ) ;
#177836=CARTESIAN_POINT ( 'NONE',  ( -3.812211943230557213E-13, -7.217909409572238033, 9.581972888692771306 ) ) ;
#177849=CARTESIAN_POINT ( 'NONE',  ( 0.000000000000000000, -7.154544010627095219, 0.000000000000000000 ) ) ;
#177901=CARTESIAN_POINT ( 'NONE',  ( 11.09544190643661210, 2.974000657017507709, -3.605127613804859799 ) ) ;
#177902=CARTESIAN_POINT ( 'NONE',  ( -10.44245235073009326, 1.000000000000000888, 5.695529491621741158 ) ) ;
#177929=DIRECTION ( 'NONE',  ( 0.000000000000000000, -1.000000000000000000, 0.000000000000000000 ) ) ;
#177939=ORIENTED_EDGE ( 'NONE', *, *, #31233, .F. ) ;
#177980=ORIENTED_EDGE ( 'NONE', *, *, #199113, .F. ) ;
#177984=( GEOMETRIC_REPRESENTATION_CONTEXT ( 3 ) GLOBAL_UNCERTAINTY_ASSIGNED_CONTEXT ( ( #63826 ) ) GLOBAL_UNIT_ASSIGNED_CONTEXT ( ( #58068, #123174, #189134 ) ) REPRESENTATION_CONTEXT ( 'NONE', 'WORKASPACE' ) );
#177991=VERTEX_POINT ( 'NONE', #183076 ) ;
#178005=CARTESIAN_POINT ( 'NONE',  ( 0.08506230894391486608, -9.914238990527385553, 9.499619272424267180 ) ) ;
#178012=EDGE_CURVE ( 'NONE', #115982, #60692, #108283, .T. ) ;
#178025=ADVANCED_FACE ( 'NONE', ( #98644 ), #50953, .T. ) ;
#178047=B_SPLINE_CURVE_WITH_KNOTS ( 'NONE', 3,
 ( #29480, #209258, #56899, #60903, #96632, #93430, #130252, #176790 ),
 .UNSPECIFIED., .F., .F.,
 ( 4, 2, 2, 4 ),
 ( 0.000000000000000000, 0.0004970278158210380409, 0.0007455417237315570614, 0.0009940556316420760818 ),
 .UNSPECIFIED. ) ;
#178145=ORIENTED_EDGE ( 'NONE', *, *, #181839, .T. ) ;
#178156=DIRECTION ( 'NONE',  ( 0.000000000000000000, -1.000000000000000000, 0.000000000000000000 ) ) ;
#178265=EDGE_CURVE ( 'NONE', #87461, #35700, #187676, .T. ) ;
#178308=CARTESIAN_POINT ( 'NONE',  ( -9.000007961041697868, 1.000000000000000888, -7.937244906211844864 ) ) ;
#178319=( BOUNDED_SURFACE ( )  B_SPLINE_SURFACE ( 3, 2, ( 
 ( #108075, #174105, #143757 ),
 ( #94983, #25677, #157841 ),
 ( #209752, #142676, #10492 ),
 ( #61393, #71480, #75507 ) ),
 .UNSPECIFIED., .F., .F., .T. ) 
 B_SPLINE_SURFACE_WITH_KNOTS ( ( 4, 4 ),
 ( 3, 3 ),
 ( 0.04893088146668654603, 0.05137248493452926945 ),
 ( 0.000000000000000000, 1.000000000000000000 ),
 .UNSPECIFIED. ) 
 GEOMETRIC_REPRESENTATION_ITEM ( )  RATIONAL_B_SPLINE_SURFACE ( (
 ( 1.000000000000000000, 0.7169884966214681299, 1.000000000000000000),
 ( 1.000000000000000000, 0.7174883642158058628, 1.000000000000000000),
 ( 1.000000000000000000, 0.7180610417773378717, 1.000000000000000000),
 ( 1.000000000000000000, 0.7187540717311196037, 1.000000000000000000) ) ) 
 REPRESENTATION_ITEM ( '' )  SURFACE ( )  );
#178409=( NAMED_UNIT ( * ) SI_UNIT ( $, .STERADIAN. ) SOLID_ANGLE_UNIT ( ) );
#178419=CARTESIAN_POINT ( 'NONE',  ( 9.029845422049886494, 1.720726420432415082, 7.609771484012845200 ) ) ;
#178421=CARTESIAN_POINT ( 'NONE',  ( -9.513083153069262110, -8.198316282515559550, 1.138412281109779656E-15 ) ) ;
#178422=AXIS2_PLACEMENT_3D ( 'NONE', #195270, #145498, #11157 ) ;
#178433=FACE_OUTER_BOUND ( 'NONE', #180276, .T. ) ;
#178473=( LENGTH_UNIT ( ) NAMED_UNIT ( * ) SI_UNIT ( .MILLI., .METRE. ) );
#178497=CARTESIAN_POINT ( 'NONE',  ( 7.721398836998361936, -6.134628647623488362, -7.721398836998387694 ) ) ;
#178501=ADVANCED_FACE ( 'NONE', ( #31005 ), #191720, .T. ) ;
#178506=CARTESIAN_POINT ( 'NONE',  ( 9.495223711095174934, -8.169755926620892339, -0.3080734816350358951 ) ) ;
#178508=VERTEX_POINT ( 'NONE', #51497 ) ;
#178509=DIRECTION ( 'NONE',  ( 0.000000000000000000, 0.000000000000000000, 1.000000000000000000 ) ) ;
#178517=AXIS2_PLACEMENT_3D ( 'NONE', #78677, #198800, #182560 ) ;
#178527=( NAMED_UNIT ( * ) SI_UNIT ( $, .STERADIAN. ) SOLID_ANGLE_UNIT ( ) );
#178576=ORIENTED_EDGE ( 'NONE', *, *, #59332, .F. ) ;
#178601=ADVANCED_FACE ( 'NONE', ( #207338 ), #118785, .F. ) ;
#178607=CARTESIAN_POINT ( 'NONE',  ( -0.08000000000000367928, 7.849261790823902629, -9.579665964948867796 ) ) ;
#178619=SURFACE_STYLE_FILL_AREA ( #96313 ) ;
#178630=CARTESIAN_POINT ( 'NONE',  ( -0.3540227772641141302, -5.166863022244726267, -10.99462479582585672 ) ) ;
#178668=CARTESIAN_POINT ( 'NONE',  ( 0.000000000000000000, 3.499999999999989342, 0.000000000000000000 ) ) ;
#178691=CARTESIAN_POINT ( 'NONE',  ( -0.3689019803513007845, -6.583711573986997578, -9.609441814500801371 ) ) ;
#178716=CARTESIAN_POINT ( 'NONE',  ( -6.396834479292370368, -8.176568542494905500, -7.055228938194266775 ) ) ;
#178786=DIRECTION ( 'NONE',  ( 0.000000000000000000, 0.000000000000000000, 1.000000000000000000 ) ) ;
#178812=AXIS2_PLACEMENT_3D ( 'NONE', #148502, #117115, #19541 ) ;
#178839=TOROIDAL_SURFACE ( 'NONE', #9360, 9.559451093910105612, 0.08000000000000000167 ) ;
#178873=CARTESIAN_POINT ( 'NONE',  ( 7.654042494670958593E-16, 0.03624871340549007392, -6.250000000000000000 ) ) ;
#178881=CARTESIAN_POINT ( 'NONE',  ( 6.381095703207996017, -8.233137084989849086, 7.037870247915945399 ) ) ;
#178886=MECHANICAL_DESIGN_GEOMETRIC_PRESENTATION_REPRESENTATION('',(#64742),#37072);
#178968=CARTESIAN_POINT ( 'NONE',  ( 6.658747417465789908, -6.682123388833677069, 6.935047222998400152 ) ) ;
#178972=FACE_OUTER_BOUND ( 'NONE', #116819, .T. ) ;
#178985=CARTESIAN_POINT ( 'NONE',  ( 6.905598479220742547, -7.287292266636080207, -6.905598479220769192 ) ) ;
#178999=( NAMED_UNIT ( * ) PLANE_ANGLE_UNIT ( ) SI_UNIT ( $, .RADIAN. ) );
#179045=CARTESIAN_POINT ( 'NONE',  ( 0.000000000000000000, -9.999999999999994671, 0.000000000000000000 ) ) ;
#179062=ORIENTED_EDGE ( 'NONE', *, *, #152080, .F. ) ;
#179111=FACE_OUTER_BOUND ( 'NONE', #72148, .T. ) ;
#179134=AXIS2_PLACEMENT_3D ( 'NONE', #131926, #181680, #165445 ) ;
#179210=VERTEX_POINT ( 'NONE', #138951 ) ;
#179300=CARTESIAN_POINT ( 'NONE',  ( 9.586610838029415049, -7.161464053357574855, -0.003376046620562692113 ) ) ;
#179303=CARTESIAN_POINT ( 'NONE',  ( -4.218316008240990271E-13, -9.350066838357692589, -9.500000000000001776 ) ) ;
#179317=ORIENTED_EDGE ( 'NONE', *, *, #54983, .F. ) ;
#179324=ADVANCED_FACE ( 'NONE', ( #38231 ), #107564, .T. ) ;
#179385=VERTEX_POINT ( 'NONE', #173599 ) ;
#179401=DIRECTION ( 'NONE',  ( 0.000000000000000000, -0.08676576675288254215, 0.9962287396576070542 ) ) ;
#179421=UNCERTAINTY_MEASURE_WITH_UNIT (LENGTH_MEASURE( 1.000000000000000082E-05 ), #83581, 'distance_accuracy_value', 'NONE');
#179427=DIRECTION ( 'NONE',  ( 0.000000000000000000, 0.000000000000000000, 1.000000000000000000 ) ) ;
#179455=ORIENTED_EDGE ( 'NONE', *, *, #134540, .T. ) ;
#179480=TOROIDAL_SURFACE ( 'NONE', #41101, 10.92000000000000171, 0.08000000000000000167 ) ;
#179485=FILL_AREA_STYLE ('',( #112408 ) ) ;
#179497=FACE_OUTER_BOUND ( 'NONE', #4771, .T. ) ;
#179514=LINE ( 'NONE', #97209, #62263 ) ;
#179526=AXIS2_PLACEMENT_3D ( 'NONE', #99005, #134722, #184490 ) ;
#179530=( BOUNDED_SURFACE ( )  B_SPLINE_SURFACE ( 3, 2, ( 
 ( #72714, #175575, #27166 ),
 ( #93271, #159304, #105248 ),
 ( #10902, #60733, #138810 ),
 ( #204829, #188604, #40236 ),
 ( #126897, #78053, #11979 ),
 ( #14093, #211237, #179829 ),
 ( #97527, #110630, #47715 ),
 ( #16221, #129029, #112760 ) ),
 .UNSPECIFIED., .F., .F., .F. ) 
 B_SPLINE_SURFACE_WITH_KNOTS ( ( 4, 2, 2, 4 ),
 ( 3, 3 ),
 ( 0.000000000000000000, 0.0002575597274893397974, 0.0005151194549786795949, 0.001030238909957359190 ),
 ( 0.000000000000000000, 1.000000000000000000 ),
 .UNSPECIFIED. ) 
 GEOMETRIC_REPRESENTATION_ITEM ( )  RATIONAL_B_SPLINE_SURFACE ( (
 ( 1.000000000000000000, 0.9238795325112797441, 1.000000000000000000),
 ( 1.000000000000000000, 0.9228594682462623044, 1.000000000000000000),
 ( 1.000000000000000000, 0.9150875845229113903, 1.000000000000000000),
 ( 1.000000000000000000, 0.8905471774190711898, 1.000000000000000000),
 ( 1.000000000000000000, 0.8740340839248519345, 1.000000000000000000),
 ( 1.000000000000000000, 0.8160099319846257915, 1.000000000000000000),
 ( 1.000000000000000000, 0.7673743911479106172, 1.000000000000000000),
 ( 1.000000000000000000, 0.7100530722070661493, 1.000000000000000000) ) ) 
 REPRESENTATION_ITEM ( '' )  SURFACE ( )  );
#179580=CARTESIAN_POINT ( 'NONE',  ( -0.08058608058608471292, -5.770897281092843834, 10.99970480893081870 ) ) ;
#179598=ORIENTED_EDGE ( 'NONE', *, *, #188352, .T. ) ;
#179686=FACE_OUTER_BOUND ( 'NONE', #90243, .T. ) ;
#179689=CIRCLE ( 'NONE', #37896, 0.07999999999999934941 ) ;
#179719=CARTESIAN_POINT ( 'NONE',  ( -10.96964784646768365, -7.712340523144905369, 0.6288774950739232095 ) ) ;
#179733=DIRECTION ( 'NONE',  ( -0.000000000000000000, -1.000000000000000000, -0.000000000000000000 ) ) ;
#179794=CIRCLE ( 'NONE', #207452, 0.08000000000000020983 ) ;
#179796=CARTESIAN_POINT ( 'NONE',  ( -8.773304256324728101, 3.742896273583257383, -7.826845210040933587 ) ) ;
#179797=CARTESIAN_POINT ( 'NONE',  ( 6.818239719371234742, -6.631671897294228124, -6.594971851908891125 ) ) ;
#179828=CARTESIAN_POINT ( 'NONE',  ( 0.000000000000000000, -9.900000000000005684, 9.579665964948883783 ) ) ;
#179829=CARTESIAN_POINT ( 'NONE',  ( 6.689804758640306659, -7.818797203689485720, -6.745710774231028495 ) ) ;
#179832=ORIENTED_EDGE ( 'NONE', *, *, #139632, .F. ) ;
#179907=ORIENTED_EDGE ( 'NONE', *, *, #72198, .T. ) ;
#179953=B_SPLINE_CURVE_WITH_KNOTS ( 'NONE', 3,
 ( #168580, #152338, #39652, #102517, #202113, #117772, #22301 ),
 .UNSPECIFIED., .F., .F.,
 ( 4, 3, 4 ),
 ( 3.314949680323801069E-05, 0.0009000000012044577329, 0.001928999666871128449 ),
 .UNSPECIFIED. ) ;
#179959=CARTESIAN_POINT ( 'NONE',  ( -0.3870735955438814879, 1.000000000000000888, 11.88799243440809050 ) ) ;
#179964=CARTESIAN_POINT ( 'NONE',  ( 10.39230484541318589, 3.499999999999989342, -6.000000000000107470 ) ) ;
#179984=ORIENTED_EDGE ( 'NONE', *, *, #161695, .T. ) ;
#180028=PLANE ( 'NONE',  #118601 ) ;
#180030=ADVANCED_FACE ( 'NONE', ( #59720 ), #36734, .T. ) ;
#180041=CARTESIAN_POINT ( 'NONE',  ( 7.834948825496934610, -6.307829212974246147, 7.720982897393585453 ) ) ;
#180049=ORIENTED_EDGE ( 'NONE', *, *, #168717, .T. ) ;
#180128=CARTESIAN_POINT ( 'NONE',  ( -9.496663239506002441, -6.863887327018314721, -0.01979922387980589255 ) ) ;
#180176=CARTESIAN_POINT ( 'NONE',  ( -7.100579091573050228, -6.583980363594990948, 6.484567079770452658 ) ) ;
#180178=B_SPLINE_CURVE_WITH_KNOTS ( 'NONE', 3,
 ( #126111, #31480, #131164, #16248, #17318, #198209 ),
 .UNSPECIFIED., .F., .F.,
 ( 4, 2, 4 ),
 ( 0.000000000000000000, 0.0002835903134653046712, 0.0005671806269306093424 ),
 .UNSPECIFIED. ) ;
#180179=( BOUNDED_SURFACE ( )  B_SPLINE_SURFACE ( 3, 2, ( 
 ( #206659, #87592, #107103 ),
 ( #6313, #187212, #153664 ),
 ( #7382, #72387, #90809 ),
 ( #188277, #104924, #203439 ),
 ( #207729, #59352, #190407 ),
 ( #156873, #74547, #125508 ),
 ( #38841, #157943, #139563 ),
 ( #8459, #172048, #103846 ) ),
 .UNSPECIFIED., .F., .F., .T. ) 
 B_SPLINE_SURFACE_WITH_KNOTS ( ( 4, 2, 2, 4 ),
 ( 3, 3 ),
 ( 0.000000000000000000, 0.0004924884914732687849, 0.0007387327372099031231, 0.0009849769829465375697 ),
 ( 0.000000000000000000, 1.000000000000000000 ),
 .UNSPECIFIED. ) 
 GEOMETRIC_REPRESENTATION_ITEM ( )  RATIONAL_B_SPLINE_SURFACE ( (
 ( 1.000000000000000000, 0.7045118851637611757, 1.000000000000000000),
 ( 1.000000000000000000, 0.7593505504064838041, 1.000000000000000000),
 ( 1.000000000000000000, 0.8104906253032566621, 1.000000000000000000),
 ( 1.000000000000000000, 0.8722646935501406906, 1.000000000000000000),
 ( 1.000000000000000000, 0.8905178607896868659, 1.000000000000000000),
 ( 1.000000000000000000, 0.9170530604351515569, 1.000000000000000000),
 ( 1.000000000000000000, 0.9248184710078943827, 1.000000000000000000),
 ( 1.000000000000000000, 0.9238795325112871826, 1.000000000000000000) ) ) 
 REPRESENTATION_ITEM ( '' )  SURFACE ( )  );
#180271=EDGE_LOOP ( 'NONE', ( #117048, #59121, #81699, #99375 ) ) ;
#180276=EDGE_LOOP ( 'NONE', ( #77573, #17393, #167040, #28411 ) ) ;
#180369=DIRECTION ( 'NONE',  ( 0.000000000000000000, 0.000000000000000000, 1.000000000000000000 ) ) ;
#180380=CARTESIAN_POINT ( 'NONE',  ( -0.04225267894259204793, -6.625438066542577609, -11.00000000000012434 ) ) ;
#180418=CARTESIAN_POINT ( 'NONE',  ( -10.43625799253213060, 3.019799309333130566, -6.025376361320772034 ) ) ;
#180435=EDGE_CURVE ( 'NONE', #156791, #93013, #196133, .T. ) ;
#180455=CARTESIAN_POINT ( 'NONE',  ( -9.612263720970512182, -6.681311647492908179, 0.1963700886236081633 ) ) ;
#180500=CARTESIAN_POINT ( 'NONE',  ( -1.874318606243677236E-12, -8.296536394940149606, 10.41260094160982064 ) ) ;
#180510=VERTEX_POINT ( 'NONE', #50937 ) ;
#180534=CARTESIAN_POINT ( 'NONE',  ( -11.35993080936265187, 3.555461883994699868, 3.691065267805003103 ) ) ;
#180581=ORIENTED_EDGE ( 'NONE', *, *, #169868, .F. ) ;
#180584=ORIENTED_EDGE ( 'NONE', *, *, #171517, .F. ) ;
#180589=FILL_AREA_STYLE_COLOUR ( '', #202339 ) ;
#180624=CARTESIAN_POINT ( 'NONE',  ( 10.98997987423604172, -6.893137084989842123, -0.4694063952341842594 ) ) ;
#180630=EDGE_CURVE ( 'NONE', #10241, #21185, #53057, .T. ) ;
#180634=CARTESIAN_POINT ( 'NONE',  ( -0.08058608058608696112, -5.907420853759267843, 10.99970480893081870 ) ) ;
#180641=CARTESIAN_POINT ( 'NONE',  ( 6.770610912236884715, -7.154544010627095219, 6.663994888585883736 ) ) ;
#180650=CARTESIAN_POINT ( 'NONE',  ( 6.396834479292349052, -8.176568542494905500, 7.055228938194280985 ) ) ;
#180674=CARTESIAN_POINT ( 'NONE',  ( 9.579417154662843714, -9.998067499250630874, -0.08973735058632786865 ) ) ;
#180684=CARTESIAN_POINT ( 'NONE',  ( 2.290347054751562528, 1.000000000000000888, -11.71088463649530453 ) ) ;
#180697=ADVANCED_FACE ( 'NONE', ( #204617 ), #117148, .F. ) ;
#180784=EDGE_LOOP ( 'NONE', ( #119896, #98278, #33559, #73945 ) ) ;
#180815=( LENGTH_UNIT ( ) NAMED_UNIT ( * ) SI_UNIT ( .MILLI., .METRE. ) );
#180824=AXIS2_PLACEMENT_3D ( 'NONE', #103679, #53854, #102605 ) ;
#180843=DIRECTION ( 'NONE',  ( 0.000000000000000000, 0.000000000000000000, 1.000000000000000000 ) ) ;
#180847=( LENGTH_UNIT ( ) NAMED_UNIT ( * ) SI_UNIT ( .MILLI., .METRE. ) );
#180917=CARTESIAN_POINT ( 'NONE',  ( -7.721398836998378812, -6.134628647623499909, 7.721398836998403681 ) ) ;
#180938=AXIS2_PLACEMENT_3D ( 'NONE', #41295, #173425, #45555 ) ;
#180947=CARTESIAN_POINT ( 'NONE',  ( -3.239364772909965661E-16, -5.511313137147274333, -11.00000000000000178 ) ) ;
#180980=B_SPLINE_CURVE_WITH_KNOTS ( 'NONE', 3,
 ( #30020, #98226, #45219, #64642, #144874, #95035, #47354 ),
 .UNSPECIFIED., .F., .F.,
 ( 4, 3, 4 ),
 ( 0.0001932293135873452484, 0.0009000000018422023643, 0.002089330742406755349 ),
 .UNSPECIFIED. ) ;
#180985=ORIENTED_EDGE ( 'NONE', *, *, #81885, .F. ) ;
#181001=ORIENTED_EDGE ( 'NONE', *, *, #118553, .T. ) ;
#181016=AXIS2_PLACEMENT_3D ( 'NONE', #206347, #56910, #123083 ) ;
#181082=DIRECTION ( 'NONE',  ( 0.000000000000000000, 0.000000000000000000, 1.000000000000000000 ) ) ;
#181123=CARTESIAN_POINT ( 'NONE',  ( 0.1653080603930551784, -5.324706741106330909, 10.99896775280371308 ) ) ;
#181147=ORIENTED_EDGE ( 'NONE', *, *, #85714, .T. ) ;
#181182=DIRECTION ( 'NONE',  ( 0.000000000000000000, 1.000000000000000000, 0.000000000000000000 ) ) ;
#181190=DIRECTION ( 'NONE',  ( 0.000000000000000000, 0.000000000000000000, 1.000000000000000000 ) ) ;
#181212=ORIENTED_EDGE ( 'NONE', *, *, #99318, .F. ) ;
#181223=DIRECTION ( 'NONE',  ( 0.000000000000000000, 0.000000000000000000, 1.000000000000000000 ) ) ;
#181246=CIRCLE ( 'NONE', #115604, 0.08000000000000001554 ) ;
#181263=SHAPE_REPRESENTATION_RELATIONSHIP ( 'NONE' , 'NONE' ,  #63688, #112039 ) ;
#181306=CIRCLE ( 'NONE', #105271, 0.08000000000000040412 ) ;
#181314=CARTESIAN_POINT ( 'NONE',  ( -1.040834085586084257E-14, -7.246166700194011767, -9.579665964935651701 ) ) ;
#181317=EDGE_CURVE ( 'NONE', #107434, #90309, #171111, .T. ) ;
#181376=CARTESIAN_POINT ( 'NONE',  ( -10.99431798667095883, -5.199791778945004772, 0.3617173305618339163 ) ) ;
#181408=CARTESIAN_POINT ( 'NONE',  ( 0.000000000000000000, 0.000000000000000000, 0.000000000000000000 ) ) ;
#181416=VERTEX_POINT ( 'NONE', #29702 ) ;
#181422=CARTESIAN_POINT ( 'NONE',  ( 0.4630894006623479942, -6.442483420144672124, 11.24798772015295789 ) ) ;
#181431=CARTESIAN_POINT ( 'NONE',  ( 1.270994156678442596E-16, -6.530144695498194096, -11.00000000000000178 ) ) ;
#181483=CARTESIAN_POINT ( 'NONE',  ( 6.661184042391356641, -7.215568602681155852, -6.773376348128788749 ) ) ;
#181492=CYLINDRICAL_SURFACE ( 'NONE', #66626, 0.08000000000000020983 ) ;
#181549=CARTESIAN_POINT ( 'NONE',  ( -1.192622389734054877E-15, -8.030730635398791506, 11.29670623088188464 ) ) ;
#181584=CARTESIAN_POINT ( 'NONE',  ( 0.000000000000000000, 4.006659545634088992, 0.000000000000000000 ) ) ;
#181585=DIRECTION ( 'NONE',  ( 0.000000000000000000, 0.000000000000000000, -1.000000000000000000 ) ) ;
#181616=CARTESIAN_POINT ( 'NONE',  ( -8.074422843256325422, -6.701288531901958834, 7.470306724221552841 ) ) ;
#181629=STYLED_ITEM ( 'NONE', ( #213072 ), #91529 ) ;
#181641=( GEOMETRIC_REPRESENTATION_CONTEXT ( 3 ) GLOBAL_UNCERTAINTY_ASSIGNED_CONTEXT ( ( #47548 ) ) GLOBAL_UNIT_ASSIGNED_CONTEXT ( ( #4115, #204449, #124390 ) ) REPRESENTATION_CONTEXT ( 'NONE', 'WORKASPACE' ) );
#181652=CARTESIAN_POINT ( 'NONE',  ( 10.97113184882213943, -5.223163831703878657, -0.3618152180564628284 ) ) ;
#181680=DIRECTION ( 'NONE',  ( 0.000000000000000000, 1.000000000000000000, 0.000000000000000000 ) ) ;
#181682=CARTESIAN_POINT ( 'NONE',  ( -6.770610912236888268, -7.154544010627095219, -6.663994888585867749 ) ) ;
#181684=CIRCLE ( 'NONE', #119469, 0.08000000000000020983 ) ;
#181695=CARTESIAN_POINT ( 'NONE',  ( 10.46159335054553807, 1.264806443676224967, -5.593087811558966393 ) ) ;
#181723=PRESENTATION_STYLE_ASSIGNMENT (( #115731 ) ) ;
#181724=FACE_OUTER_BOUND ( 'NONE', #197415, .T. ) ;
#181775=VECTOR ( 'NONE', #109366, 1000.000000000000000 ) ;
#181792=EDGE_CURVE ( 'NONE', #93109, #182484, #61424, .T. ) ;
#181795=AXIS2_PLACEMENT_3D ( 'NONE', #126917, #44530, #94354 ) ;
#181808=AXIS2_PLACEMENT_3D ( 'NONE', #205168, #122979, #54672 ) ;
#181810=DIRECTION ( 'NONE',  ( 0.000000000000000000, -1.000000000000000000, 0.000000000000000000 ) ) ;
#181818=CARTESIAN_POINT ( 'NONE',  ( -9.500338091956020747, -7.818966704647505317, -0.03919461954075445509 ) ) ;
#181839=EDGE_CURVE ( 'NONE', #66830, #212186, #120974, .T. ) ;
#181893=CARTESIAN_POINT ( 'NONE',  ( 10.85277107007934205, 3.956598013261175772, -3.932872935640606915 ) ) ;
#181895=DIRECTION ( 'NONE',  ( 0.000000000000000000, 0.000000000000000000, 1.000000000000000000 ) ) ;
#181897=COLOUR_RGB ( '', 0.08235294, 0.09019608, 0.10196078) ;
#181907=ADVANCED_FACE ( 'NONE', ( #184456 ), #103175, .T. ) ;
#181931=CARTESIAN_POINT ( 'NONE',  ( -0.08506230894392234620, -9.914238990527385553, -9.499619272424258298 ) ) ;
#181943=DIRECTION ( 'NONE',  ( -0.000000000000000000, 1.000000000000000000, -0.000000000000000000 ) ) ;
#181997=DIRECTION ( 'NONE',  ( 0.000000000000000000, 0.000000000000000000, 1.000000000000000000 ) ) ;
#182006=( LENGTH_UNIT ( ) NAMED_UNIT ( * ) SI_UNIT ( .MILLI., .METRE. ) );
#182008=CARTESIAN_POINT ( 'NONE',  ( -2.331034670843834533E-15, -6.920331743278509862, 9.905860218026841579 ) ) ;
#182026=DIRECTION ( 'NONE',  ( 8.659560562354853972E-17, -0.7071067811865540120, 0.7071067811865410224 ) ) ;
#182098=ADVANCED_FACE ( 'NONE', ( #201757 ), #185522, .T. ) ;
#182116=AXIS2_PLACEMENT_3D ( 'NONE', #29865, #130629, #180369 ) ;
#182131=CARTESIAN_POINT ( 'NONE',  ( 9.491602870538727643, -9.241975548351300418, -0.4178506376739458683 ) ) ;
#182153=CARTESIAN_POINT ( 'NONE',  ( 9.797921721691059460, 3.956598013261175772, 6.103348209225848642 ) ) ;
#182158=CARTESIAN_POINT ( 'NONE',  ( -8.867053104062382118, 4.021557182957048227, -7.983930475901429347 ) ) ;
#182169=ORIENTED_EDGE ( 'NONE', *, *, #97288, .F. ) ;
#182178=AXIS2_PLACEMENT_3D ( 'NONE', #199122, #165585, #83253 ) ;
#182214=CARTESIAN_POINT ( 'NONE',  ( -6.637758778446696262, -7.996947095390848581, -6.849430810391457847 ) ) ;
#182233=CARTESIAN_POINT ( 'NONE',  ( 0.01083140255523393387, -7.162053774861991684, 9.500385102287575378 ) ) ;
#182250=AXIS2_PLACEMENT_3D ( 'NONE', #8665, #111576, #62745 ) ;
#182267=CARTESIAN_POINT ( 'NONE',  ( -9.499668754385634628, -7.559700871049417792, -0.07933194154487524519 ) ) ;
#182320=( NAMED_UNIT ( * ) SI_UNIT ( $, .STERADIAN. ) SOLID_ANGLE_UNIT ( ) );
#182418=EDGE_CURVE ( 'NONE', #104249, #105884, #73863, .T. ) ;
#182421=EDGE_CURVE ( 'NONE', #143658, #29860, #147467, .T. ) ;
#182484=VERTEX_POINT ( 'NONE', #179959 ) ;
#182503=AXIS2_PLACEMENT_3D ( 'NONE', #131892, #52727, #20213 ) ;
#182546=AXIS2_PLACEMENT_3D ( 'NONE', #43451, #41321, #142032 ) ;
#182554=VERTEX_POINT ( 'NONE', #160504 ) ;
#182560=DIRECTION ( 'NONE',  ( 0.000000000000000000, 0.000000000000000000, 1.000000000000000000 ) ) ;
#182623=VERTEX_POINT ( 'NONE', #177831 ) ;
#182637=CARTESIAN_POINT ( 'NONE',  ( 9.500350659417458488, -7.217450603046484225, -0.002323312720761049489 ) ) ;
#182654=CARTESIAN_POINT ( 'NONE',  ( -0.08000000000000194456, -8.407420853759283830, -10.91970695577494865 ) ) ;
#182664=CARTESIAN_POINT ( 'NONE',  ( 0.09999999999985714760, -10.00000000000009592, 9.579478065114059859 ) ) ;
#182674=EDGE_CURVE ( 'NONE', #86477, #6643, #63976, .T. ) ;
#182680=DIRECTION ( 'NONE',  ( 1.000000000000000000, 1.084202172485501594E-14, 0.000000000000000000 ) ) ;
#182694=DIRECTION ( 'NONE',  ( 0.000000000000000000, 1.000000000000000000, 0.000000000000000000 ) ) ;
#182758=CARTESIAN_POINT ( 'NONE',  ( 6.764690511086886823E-16, -5.511313137147262786, 11.00000000000000178 ) ) ;
#182762=B_SPLINE_CURVE_WITH_KNOTS ( 'NONE', 3,
 ( #145316, #211320, #148477, #62944 ),
 .UNSPECIFIED., .F., .F.,
 ( 4, 4 ),
 ( 0.000000000000000000, 0.0002908967400263822562 ),
 .UNSPECIFIED. ) ;
#182766=CARTESIAN_POINT ( 'NONE',  ( 6.772457744868908947, -7.185026885899450377, 6.662118508819615315 ) ) ;
#182811=EDGE_CURVE ( 'NONE', #129023, #82463, #194920, .T. ) ;
#182816=( GEOMETRIC_REPRESENTATION_CONTEXT ( 3 ) GLOBAL_UNCERTAINTY_ASSIGNED_CONTEXT ( ( #148250 ) ) GLOBAL_UNIT_ASSIGNED_CONTEXT ( ( #121366, #171092, #58419 ) ) REPRESENTATION_CONTEXT ( 'NONE', 'WORKASPACE' ) );
#182858=ORIENTED_EDGE ( 'NONE', *, *, #82593, .T. ) ;
#182888=DIRECTION ( 'NONE',  ( 0.000000000000000000, 0.000000000000000000, -1.000000000000000000 ) ) ;
#183006=CARTESIAN_POINT ( 'NONE',  ( -8.064677165291197269, -5.223431457505076203, 7.446209719563364082 ) ) ;
#183010=CARTESIAN_POINT ( 'NONE',  ( 8.917737905728806425, 3.447199233515649386, 8.029567276306217138 ) ) ;
#183021=VERTEX_POINT ( 'NONE', #103041 ) ;
#183043=ORIENTED_EDGE ( 'NONE', *, *, #27140, .T. ) ;
#183060=DIRECTION ( 'NONE',  ( 0.000000000000000000, -1.000000000000000000, 0.000000000000000000 ) ) ;
#183076=CARTESIAN_POINT ( 'NONE',  ( -6.484567079770452658, -6.583980363594976737, -7.100579091573040458 ) ) ;
#183078=DIRECTION ( 'NONE',  ( 0.000000000000000000, -1.000000000000000000, 0.000000000000000000 ) ) ;
#183107=CARTESIAN_POINT ( 'NONE',  ( 1.408343819019454993E-15, 4.000000000000003553, 11.49999999999998934 ) ) ;
#183121=DIRECTION ( 'NONE',  ( -0.9999753971658824625, 0.000000000000000000, 0.007014632059889242682 ) ) ;
#183133=VERTEX_POINT ( 'NONE', #161397 ) ;
#183157=DIRECTION ( 'NONE',  ( 0.6743504407188151140, 0.000000000000000000, 0.7384114592165670343 ) ) ;
#183172=CARTESIAN_POINT ( 'NONE',  ( 9.871989323747737188, 3.235871879154604169, 6.146221223954385415 ) ) ;
#183209=CARTESIAN_POINT ( 'NONE',  ( 9.481348452320355946, -9.199999999999983302, -0.5950054837414361364 ) ) ;
#183226=CARTESIAN_POINT ( 'NONE',  ( 0.1747071867222109443, -7.850481869465713913, -10.96497182194659281 ) ) ;
#183231=CARTESIAN_POINT ( 'NONE',  ( 9.994890815243271831, 3.870538056096196833, 5.945519334325363836 ) ) ;
#183232=AXIS2_PLACEMENT_3D ( 'NONE', #50321, #116439, #132670 ) ;
#183241=ORIENTED_EDGE ( 'NONE', *, *, #45284, .T. ) ;
#183248=ORIENTED_EDGE ( 'NONE', *, *, #119616, .T. ) ;
#183306=CARTESIAN_POINT ( 'NONE',  ( -9.911098634504678095E-13, -7.246166700193024113, 9.500331257164617682 ) ) ;
#183422=VERTEX_POINT ( 'NONE', #43386 ) ;
#183451=CARTESIAN_POINT ( 'NONE',  ( -5.204170427930421283E-15, -1.000000000000000888, -12.26547674076639716 ) ) ;
#183495=EDGE_CURVE ( 'NONE', #183546, #113976, #174236, .T. ) ;
#183499=( BOUNDED_SURFACE ( )  B_SPLINE_SURFACE ( 3, 2, ( 
 ( #40684, #138182, #153353 ),
 ( #69934, #168532, #120931 ),
 ( #204192, #202058, #53718 ),
 ( #41759, #139247, #119851 ) ),
 .UNSPECIFIED., .F., .F., .T. ) 
 B_SPLINE_SURFACE_WITH_KNOTS ( ( 4, 4 ),
 ( 3, 3 ),
 ( 0.005239860189960142932, 0.008266248133684681726 ),
 ( 0.000000000000000000, 1.000000000000000000 ),
 .UNSPECIFIED. ) 
 GEOMETRIC_REPRESENTATION_ITEM ( )  RATIONAL_B_SPLINE_SURFACE ( (
 ( 1.000000000000000000, 0.7187737999613679207, 1.000000000000000000),
 ( 1.000000000000000000, 0.7186585579881036301, 1.000000000000000000),
 ( 1.000000000000000000, 0.7185467277397536989, 1.000000000000000000),
 ( 1.000000000000000000, 0.7184380228464066764, 1.000000000000000000) ) ) 
 REPRESENTATION_ITEM ( '' )  SURFACE ( )  );
#183546=VERTEX_POINT ( 'NONE', #50825 ) ;
#183547=CARTESIAN_POINT ( 'NONE',  ( 9.611175950047698535, -6.604184692106344734, -0.3106162252735243934 ) ) ;
#183550=VERTEX_POINT ( 'NONE', #212244 ) ;
#183561=EDGE_CURVE ( 'NONE', #7171, #205917, #22028, .T. ) ;
#183565=CARTESIAN_POINT ( 'NONE',  ( -6.447678837262236229, -6.532648880268781433, -6.949550370341204264 ) ) ;
#183572=MECHANICAL_DESIGN_GEOMETRIC_PRESENTATION_REPRESENTATION('',(#17652),#190523);
#183636=EDGE_CURVE ( 'NONE', #51191, #183133, #108562, .T. ) ;
#183643=EDGE_CURVE ( 'NONE', #143658, #187130, #163866, .T. ) ;
#183707=VERTEX_POINT ( 'NONE', #149394 ) ;
#183727=AXIS2_PLACEMENT_3D ( 'NONE', #178668, #179733, #81153 ) ;
#183752=VERTEX_POINT ( 'NONE', #133179 ) ;
#183788=LINE ( 'NONE', #101473, #3815 ) ;
#183812=ORIENTED_EDGE ( 'NONE', *, *, #18617, .T. ) ;
#183829=CARTESIAN_POINT ( 'NONE',  ( 0.000000000000000000, 7.849261790823902629, 0.000000000000000000 ) ) ;
#183871=FACE_OUTER_BOUND ( 'NONE', #48326, .T. ) ;
#183887=CARTESIAN_POINT ( 'NONE',  ( -10.91962425643211532, -9.999999999999998224, 0.09058751758334862569 ) ) ;
#183938=DIRECTION ( 'NONE',  ( 0.6743504407188133376, -1.091556109765015220E-14, 0.7384114592165688107 ) ) ;
#183955=FILL_AREA_STYLE ('',( #19316 ) ) ;
#183967=ORIENTED_EDGE ( 'NONE', *, *, #100257, .F. ) ;
#184019=AXIS2_PLACEMENT_3D ( 'NONE', #132282, #200418, #119254 ) ;
#184032=EDGE_CURVE ( 'NONE', #114840, #21185, #4845, .T. ) ;
#184050=EDGE_CURVE ( 'NONE', #157333, #166319, #185315, .T. ) ;
#184067=CARTESIAN_POINT ( 'NONE',  ( -0.08228926980218694009, -9.910743320677065427, -9.499643698783447832 ) ) ;
#184102=ORIENTED_EDGE ( 'NONE', *, *, #168972, .F. ) ;
#184110=DIRECTION ( 'NONE',  ( -0.01745240643728004568, 0.000000000000000000, -0.9998476951563913806 ) ) ;
#184117=CIRCLE ( 'NONE', #90773, 0.08000000000000044575 ) ;
#184143=FACE_OUTER_BOUND ( 'NONE', #15712, .T. ) ;
#184174=( NAMED_UNIT ( * ) SI_UNIT ( $, .STERADIAN. ) SOLID_ANGLE_UNIT ( ) );
#184208=CARTESIAN_POINT ( 'NONE',  ( -7.057683771862373945, -6.583723166013941253, 6.531918710723850552 ) ) ;
#184211=CARTESIAN_POINT ( 'NONE',  ( -7.460470246983022413, -6.805008568744149500, -7.900729602272508423 ) ) ;
#184212=VERTEX_POINT ( 'NONE', #149131 ) ;
#184243=VECTOR ( 'NONE', #101966, 1000.000000000000000 ) ;
#184269=CIRCLE ( 'NONE', #101243, 11.99999999999999112 ) ;
#184293=CARTESIAN_POINT ( 'NONE',  ( -9.043854491631282855, 2.018041202053908023, -8.143123160305936636 ) ) ;
#184338=EDGE_CURVE ( 'NONE', #179385, #16492, #179953, .T. ) ;
#184366=CARTESIAN_POINT ( 'NONE',  ( 6.484567079770445552, -6.583980363594983842, 7.100579091573057333 ) ) ;
#184376=CARTESIAN_POINT ( 'NONE',  ( 0.1132184859782718600, 3.829867255648774726, -11.66962136008044304 ) ) ;
#184379=CARTESIAN_POINT ( 'NONE',  ( 7.100579091573050228, -6.583980363594990948, -6.484567079770450881 ) ) ;
#184431=VERTEX_POINT ( 'NONE', #53773 ) ;
#184456=FACE_OUTER_BOUND ( 'NONE', #145304, .T. ) ;
#184467=SURFACE_STYLE_USAGE ( .BOTH. , #149866 ) ;
#184490=DIRECTION ( 'NONE',  ( 0.000000000000000000, 0.000000000000000000, -1.000000000000000000 ) ) ;
#184502=ORIENTED_EDGE ( 'NONE', *, *, #81818, .T. ) ;
#184507=CARTESIAN_POINT ( 'NONE',  ( 6.500815859342971237, -6.554751161430536932, 6.901817408925775332 ) ) ;
#184562=CARTESIAN_POINT ( 'NONE',  ( -10.99462479582586738, -5.166863022246599435, 0.3540227772641256210 ) ) ;
#184573=CARTESIAN_POINT ( 'NONE',  ( 10.99943592164172657, -9.900000000000005684, -0.1113975120798811613 ) ) ;
#184591=EDGE_CURVE ( 'NONE', #94238, #69637, #143329, .T. ) ;
#184656=EDGE_CURVE ( 'NONE', #82080, #50087, #181306, .T. ) ;
#184678=( NAMED_UNIT ( * ) PLANE_ANGLE_UNIT ( ) SI_UNIT ( $, .RADIAN. ) );
#184735=EDGE_CURVE ( 'NONE', #41100, #15288, #164016, .T. ) ;
#184758=VERTEX_POINT ( 'NONE', #85196 ) ;
#184761=FILL_AREA_STYLE_COLOUR ( '', #114781 ) ;
#184771=EDGE_CURVE ( 'NONE', #77260, #60029, #35373, .T. ) ;
#184803=ADVANCED_FACE ( 'NONE', ( #155547 ), #35457, .F. ) ;
#184826=VERTEX_POINT ( 'NONE', #137170 ) ;
#184838=CARTESIAN_POINT ( 'NONE',  ( -7.037870247915956945, -8.233137084989836652, 6.381095703207982694 ) ) ;
#184880=CARTESIAN_POINT ( 'NONE',  ( 10.99970480893080627, -6.221252899067775566, 0.08058608058608524027 ) ) ;
#184918=CARTESIAN_POINT ( 'NONE',  ( -6.381095703207996905, -8.233137084989849086, -7.037870247915946287 ) ) ;
#184986=UNCERTAINTY_MEASURE_WITH_UNIT (LENGTH_MEASURE( 1.000000000000000082E-05 ), #182006, 'distance_accuracy_value', 'NONE');
#184989=CARTESIAN_POINT ( 'NONE',  ( 0.000000000000000000, -9.919999999999998153, 0.000000000000000000 ) ) ;
#184995=CIRCLE ( 'NONE', #119372, 0.08000000000000040412 ) ;
#185021=EDGE_LOOP ( 'NONE', ( #109677, #174157, #19703, #34835, #116629, #62322 ) ) ;
#185033=FILL_AREA_STYLE ('',( #103816 ) ) ;
#185040=DIRECTION ( 'NONE',  ( 0.000000000000000000, -1.000000000000000000, 0.000000000000000000 ) ) ;
#185041=CARTESIAN_POINT ( 'NONE',  ( -0.4373225248172993851, -5.223431457505089526, -10.96785329849811497 ) ) ;
#185061=CARTESIAN_POINT ( 'NONE',  ( 8.832353407160718817, 3.956598013261175772, 7.432338980325266853 ) ) ;
#185072=DIRECTION ( 'NONE',  ( -1.000000000000000000, 0.000000000000000000, 0.000000000000000000 ) ) ;
#185125=CARTESIAN_POINT ( 'NONE',  ( -0.07971467182326515133, -9.904506264776385294, -9.499665578938831345 ) ) ;
#185133=CARTESIAN_POINT ( 'NONE',  ( -6.875062624577635617, -8.049367966558001797, 6.605500049835224097 ) ) ;
#185142=CARTESIAN_POINT ( 'NONE',  ( 7.550983558724436051, -6.148216694138042726, 7.550983558724430722 ) ) ;
#185151=CARTESIAN_POINT ( 'NONE',  ( -9.499562802171206854, -9.415754203682764611, 0.1226201807150902046 ) ) ;
#185158=FACE_OUTER_BOUND ( 'NONE', #204272, .T. ) ;
#185161=( BOUNDED_SURFACE ( )  B_SPLINE_SURFACE ( 3, 2, ( 
 ( #166977, #183209, #103036 ),
 ( #36956, #18568, #200508 ),
 ( #168033, #66228, #48966 ),
 ( #133437, #182131, #67298 ),
 ( #83574, #149655, #199444 ),
 ( #70497, #69438, #201569 ),
 ( #84644, #150735, #115084 ),
 ( #51087, #53215, #148592 ) ),
 .UNSPECIFIED., .F., .F., .F. ) 
 B_SPLINE_SURFACE_WITH_KNOTS ( ( 4, 2, 2, 4 ),
 ( 3, 3 ),
 ( 0.000000000000000000, 0.0002469787127373868161, 0.0004939574254747736322, 0.0009879148509495472644 ),
 ( 0.000000000000000000, 1.000000000000000000 ),
 .UNSPECIFIED. ) 
 GEOMETRIC_REPRESENTATION_ITEM ( )  RATIONAL_B_SPLINE_SURFACE ( (
 ( 1.000000000000000000, 0.3826834323650769032, 1.000000000000000000),
 ( 1.000000000000000000, 0.3798541548344007701, 1.000000000000000000),
 ( 1.000000000000000000, 0.3995981355978897587, 1.000000000000000000),
 ( 1.000000000000000000, 0.4556299950042955182, 1.000000000000000000),
 ( 1.000000000000000000, 0.4903550589607370558, 1.000000000000000000),
 ( 1.000000000000000000, 0.5915489574622737612, 1.000000000000000000),
 ( 1.000000000000000000, 0.6554239218402749811, 1.000000000000000000),
 ( 1.000000000000000000, 0.7100530722070640399, 1.000000000000000000) ) ) 
 REPRESENTATION_ITEM ( '' )  SURFACE ( )  );
#185177=FACE_OUTER_BOUND ( 'NONE', #84888, .T. ) ;
#185182=CARTESIAN_POINT ( 'NONE',  ( -10.35569247086017697, 1.405922845961228962, -6.063183772476178568 ) ) ;
#185194=CARTESIAN_POINT ( 'NONE',  ( 0.000000000000000000, 1.000000000000000888, 0.000000000000000000 ) ) ;
#185204=CIRCLE ( 'NONE', #133315, 0.07999999999999951594 ) ;
#185234=DIRECTION ( 'NONE',  ( -1.084202172485362439E-14, -1.000000000000000000, -3.260636891504970529E-14 ) ) ;
#185245=CARTESIAN_POINT ( 'NONE',  ( 10.72111444838738059, -6.105866302527761746, 9.269928574751062911E-15 ) ) ;
#185272=CARTESIAN_POINT ( 'NONE',  ( -6.864213375409984330, -6.776276029125434697, 6.558483974469869082 ) ) ;
#185279=CARTESIAN_POINT ( 'NONE',  ( -3.239364772909965661E-16, -5.511313137147274333, -11.00000000000000178 ) ) ;
#185287=EDGE_LOOP ( 'NONE', ( #82319, #154170, #195925, #192073 ) ) ;
#185315=B_SPLINE_CURVE_WITH_KNOTS ( 'NONE', 3,
 ( #209853, #141726, #127656, #144917, #90814, #189357, #40997, #156878, #107108, #173131 ),
 .UNSPECIFIED., .F., .F.,
 ( 4, 2, 2, 2, 4 ),
 ( 0.000000000000000000, 0.0002216178067634634239, 0.0004432356135269268477, 0.0006648534202903903529, 0.0008864712270538519607 ),
 .UNSPECIFIED. ) ;
#185319=CARTESIAN_POINT ( 'NONE',  ( -7.978162878861394525, -5.230039540835476508, 7.573156686838125928 ) ) ;
#185339=CARTESIAN_POINT ( 'NONE',  ( -10.91339599544322780, -6.211932585243250315, -0.000000000000000000 ) ) ;
#185379=EDGE_CURVE ( 'NONE', #90864, #135683, #19960, .T. ) ;
#185392=LINE ( 'NONE', #168094, #140241 ) ;
#185395=CARTESIAN_POINT ( 'NONE',  ( -1.734723475976807094E-15, -8.407420853759283830, -10.91970695577494332 ) ) ;
#185413=CARTESIAN_POINT ( 'NONE',  ( -10.91944002402979130, -8.407420853759269619, 0.1105873483556677611 ) ) ;
#185427=DIRECTION ( 'NONE',  ( 0.000000000000000000, 1.000000000000000000, 0.000000000000000000 ) ) ;
#185439=ORIENTED_EDGE ( 'NONE', *, *, #28829, .T. ) ;
#185443=CARTESIAN_POINT ( 'NONE',  ( 10.99956415888072492, -9.918872522958837479, -0.09791994008662846527 ) ) ;
#185446=B_SPLINE_CURVE_WITH_KNOTS ( 'NONE', 3,
 ( #180947, #32569, #164703, #16291, #82376, #35 ),
 .UNSPECIFIED., .F., .F.,
 ( 4, 2, 4 ),
 ( 0.0004065497138311778428, 0.0007003026727366230050, 0.0009940556316420680587 ),
 .UNSPECIFIED. ) ;
#185459=CIRCLE ( 'NONE', #99062, 10.97656854249491509 ) ;
#185469=CARTESIAN_POINT ( 'NONE',  ( -1.040834085586084257E-14, -9.911192057434348612, -9.579665964948867796 ) ) ;
#185480=CARTESIAN_POINT ( 'NONE',  ( -0.1062647551456016304, -6.683951888245086792, -9.488025208486867257 ) ) ;
#185505=EDGE_CURVE ( 'NONE', #120494, #189233, #48399, .T. ) ;
#185522=PLANE ( 'NONE',  #49736 ) ;
#185570=ORIENTED_EDGE ( 'NONE', *, *, #99318, .T. ) ;
#185576=CARTESIAN_POINT ( 'NONE',  ( 6.594971851908695726, -6.631671897293982987, 6.818239719371404384 ) ) ;
#185589=ORIENTED_EDGE ( 'NONE', *, *, #166279, .T. ) ;
#185594=CARTESIAN_POINT ( 'NONE',  ( -0.07933194154489606187, -9.609467486116969326, -9.499668754385620417 ) ) ;
#185595=ORIENTED_EDGE ( 'NONE', *, *, #157678, .F. ) ;
#185601=FACE_OUTER_BOUND ( 'NONE', #91306, .T. ) ;
#185647=EDGE_LOOP ( 'NONE', ( #144933, #205658, #69011, #68145, #90627, #42391, #137513, #160413, #210279, #14865, #22398, #125204, #202708 ) ) ;
#185652=AXIS2_PLACEMENT_3D ( 'NONE', #26786, #162145, #47339 ) ;
#185657=DIRECTION ( 'NONE',  ( 0.000000000000000000, 0.000000000000000000, 1.000000000000000000 ) ) ;
#185676=ORIENTED_EDGE ( 'NONE', *, *, #44682, .T. ) ;
#185688=CARTESIAN_POINT ( 'NONE',  ( -6.776593369756422902, -7.026643280347922627, -6.796618584848064692 ) ) ;
#185715=AXIS2_PLACEMENT_3D ( 'NONE', #41114, #29109, #93064 ) ;
#185724=DIRECTION ( 'NONE',  ( 0.000000000000000000, 1.000000000000000000, 0.000000000000000000 ) ) ;
#185746=AXIS2_PLACEMENT_3D ( 'NONE', #112543, #212086, #177488 ) ;
#185776=DIRECTION ( 'NONE',  ( 0.000000000000000000, 0.000000000000000000, 1.000000000000000000 ) ) ;
#185789=AXIS2_PLACEMENT_3D ( 'NONE', #133128, #161334, #47601 ) ;
#185797=CARTESIAN_POINT ( 'NONE',  ( -1.020505294851981049E-14, -5.907420853759271395, -10.91970695577494332 ) ) ;
#185836=DIRECTION ( 'NONE',  ( -1.000000000000000000, 0.000000000000000000, 0.000000000000000000 ) ) ;
#185845=CARTESIAN_POINT ( 'NONE',  ( 10.18461545817735470, 3.956598013261175772, -5.433575010662928584 ) ) ;
#185846=B_SPLINE_CURVE_WITH_KNOTS ( 'NONE', 3,
 ( #188030, #190168, #124204, #58040 ),
 .UNSPECIFIED., .F., .F.,
 ( 4, 4 ),
 ( 0.000000000000000000, 9.170750102251527260E-05 ),
 .UNSPECIFIED. ) ;
#185866=CARTESIAN_POINT ( 'NONE',  ( 0.000000000000000000, 0.000000000000000000, 0.000000000000000000 ) ) ;
#185941=B_SPLINE_CURVE_WITH_KNOTS ( 'NONE', 3,
 ( #57185, #187172, #108135, #91845, #25734, #173083, #158953, #9496, #39875, #92907, #122277, #24664, #75568, #207690, #59309, #38800 ),
 .UNSPECIFIED., .F., .F.,
 ( 4, 3, 3, 3, 3, 4 ),
 ( 5.421010862428817358E-20, 2.208392919728564190E-05, 5.593630375490294554E-05, 8.978950068604114713E-05, 0.0001236430975991122182, 0.0001574962648025070408 ),
 .UNSPECIFIED. ) ;
#186070=AXIS2_PLACEMENT_3D ( 'NONE', #104469, #39454, #154282 ) ;
#186088=ORIENTED_EDGE ( 'NONE', *, *, #130618, .F. ) ;
#186092=CARTESIAN_POINT ( 'NONE',  ( -9.498564853506350047, -8.073984524010683117, 0.1796516426514711273 ) ) ;
#186101=SURFACE_STYLE_FILL_AREA ( #37731 ) ;
#186146=AXIS2_PLACEMENT_3D ( 'NONE', #185866, #37501, #52682 ) ;
#186169=CARTESIAN_POINT ( 'NONE',  ( 2.373851744317274193, 1.000000000000000888, -11.76285798163019969 ) ) ;
#186196=CARTESIAN_POINT ( 'NONE',  ( 7.905503641038563956, -6.808400134080580202, -7.455003611050280199 ) ) ;
#186215=CIRCLE ( 'NONE', #16752, 0.08000000000000020983 ) ;
#186223=CARTESIAN_POINT ( 'NONE',  ( -10.95855051086948606, -7.723431457505092190, 0.6286713519884027379 ) ) ;
#186225=DIRECTION ( 'NONE',  ( 0.000000000000000000, -1.000000000000000000, 0.000000000000000000 ) ) ;
#186228=CARTESIAN_POINT ( 'NONE',  ( 0.000000000000000000, 15.50000000000019362, 0.000000000000000000 ) ) ;
#186230=FILL_AREA_STYLE ('',( #167866 ) ) ;
#186247=CARTESIAN_POINT ( 'NONE',  ( -0.4359508081057549833, -6.362962251423736504, -9.827407719474871683 ) ) ;
#186266=FACE_OUTER_BOUND ( 'NONE', #47447, .T. ) ;
#186269=ORIENTED_EDGE ( 'NONE', *, *, #137160, .T. ) ;
#186274=CARTESIAN_POINT ( 'NONE',  ( 0.000000000000000000, 0.000000000000000000, 0.000000000000000000 ) ) ;
#186295=CARTESIAN_POINT ( 'NONE',  ( 9.500102690074733403, -7.891095720666440272, -0.004933703209193082348 ) ) ;
#186317=CARTESIAN_POINT ( 'NONE',  ( -11.38999389752409819, 1.405705671057795092, 3.777644806142836487 ) ) ;
#186328=EDGE_CURVE ( 'NONE', #21185, #6643, #146616, .T. ) ;
#186342=CARTESIAN_POINT ( 'NONE',  ( 7.847520364415523808, -5.402328468025352493, -7.653681110113485175 ) ) ;
#186353=ORIENTED_EDGE ( 'NONE', *, *, #187477, .T. ) ;
#186386=CARTESIAN_POINT ( 'NONE',  ( -7.761717428875326341, -5.600320323339592399, 7.717216217110903109 ) ) ;
#186393=VERTEX_POINT ( 'NONE', #134585 ) ;
#186402=CARTESIAN_POINT ( 'NONE',  ( -2.391594655221676469, 3.742896273583256050, 11.51132696612781814 ) ) ;
#186430=CARTESIAN_POINT ( 'NONE',  ( -7.439168848974001769, -6.893137084989842123, -8.103009739377998955 ) ) ;
#186431=EDGE_LOOP ( 'NONE', ( #100812, #148553, #66790, #54830 ) ) ;
#186461=EDGE_CURVE ( 'NONE', #82463, #207870, #79451, .T. ) ;
#186468=CARTESIAN_POINT ( 'NONE',  ( 0.4373349612950711007, -5.212340523078045962, 10.97895254167818280 ) ) ;
#186475=CARTESIAN_POINT ( 'NONE',  ( 0.04765083308771843329, -6.900199406649612399, 9.605391220871890567 ) ) ;
#186479=EDGE_CURVE ( 'NONE', #115124, #110438, #115814, .T. ) ;
#186480=STYLED_ITEM ( 'NONE', ( #101563 ), #158480 ) ;
#186483=EDGE_CURVE ( 'NONE', #100589, #58795, #107450, .T. ) ;
#186487=CARTESIAN_POINT ( 'NONE',  ( 9.499750697158754420, -9.920000000031521381, -0.06885943948997400033 ) ) ;
#186499=CARTESIAN_POINT ( 'NONE',  ( 10.91804383151479740, -8.407420853759283830, -0.1905751639681655396 ) ) ;
#186508=CARTESIAN_POINT ( 'NONE',  ( 6.684387857553273804, -6.724344753046613832, 6.908358566921364741 ) ) ;
#186516=CARTESIAN_POINT ( 'NONE',  ( 10.99944088594791580, -9.904389777384739801, -0.1109062511178756510 ) ) ;
#186521=DIRECTION ( 'NONE',  ( 0.7347175152297782397, 3.929830605827906454E-15, -0.6783731810844091381 ) ) ;
#186540=CARTESIAN_POINT ( 'NONE',  ( -6.773376349083141790, -7.246166700180801001, -6.661184041420938229 ) ) ;
#186542=CARTESIAN_POINT ( 'NONE',  ( -1.040834085586084257E-14, -9.900000000000005684, -9.579665964948867796 ) ) ;
#186547=EDGE_CURVE ( 'NONE', #49868, #75305, #190746, .T. ) ;
#186606=EDGE_CURVE ( 'NONE', #29173, #139878, #109591, .T. ) ;
#186607=ORIENTED_EDGE ( 'NONE', *, *, #101175, .T. ) ;
#186619=ORIENTED_EDGE ( 'NONE', *, *, #184050, .F. ) ;
#186635=EDGE_CURVE ( 'NONE', #18108, #184431, #160605, .T. ) ;
#186641=CARTESIAN_POINT ( 'NONE',  ( -7.580882385731773532, -6.105993949506148155, -7.580882385731739781 ) ) ;
#186652=ORIENTED_EDGE ( 'NONE', *, *, #195653, .T. ) ;
#186657=CARTESIAN_POINT ( 'NONE',  ( 0.000000000000000000, -6.893137084989842123, 0.000000000000000000 ) ) ;
#186666=CARTESIAN_POINT ( 'NONE',  ( -0.05436647835300534304, -9.474608021433725824, -9.500000000000147438 ) ) ;
#186673=CARTESIAN_POINT ( 'NONE',  ( -6.722000117219788073, -7.189371949512781690, 6.713552092916484249 ) ) ;
#186704=CARTESIAN_POINT ( 'NONE',  ( 6.992767129439140028, -7.336076765398686028, 7.649321060469624456 ) ) ;
#186726=EDGE_CURVE ( 'NONE', #60692, #166808, #93292, .T. ) ;
#186771=CARTESIAN_POINT ( 'NONE',  ( 0.1062647697984270417, -6.683951901172196841, 9.488025208946959665 ) ) ;
#186808=DIRECTION ( 'NONE',  ( -1.000000000000000000, -0.000000000000000000, -0.000000000000000000 ) ) ;
#186828=CARTESIAN_POINT ( 'NONE',  ( -10.99968117833243220, -6.698521824825906634, 0.09510031644099410653 ) ) ;
#186853=EDGE_CURVE ( 'NONE', #170487, #98224, #207002, .T. ) ;
#186858=FACE_OUTER_BOUND ( 'NONE', #70444, .T. ) ;
#186874=DIRECTION ( 'NONE',  ( -0.000000000000000000, -1.000000000000000000, -0.000000000000000000 ) ) ;
#186889=ORIENTED_EDGE ( 'NONE', *, *, #133466, .T. ) ;
#186922=CARTESIAN_POINT ( 'NONE',  ( 10.99873804690151147, -8.265528217051443249, -0.1803058380980962216 ) ) ;
#186954=CARTESIAN_POINT ( 'NONE',  ( -0.4294425147611594107, -9.006862915010128035, 9.490288674561789151 ) ) ;
#186972=VERTEX_POINT ( 'NONE', #159328 ) ;
#186986=CARTESIAN_POINT ( 'NONE',  ( -7.721398836998370818, -5.907420853759296264, 7.721398836998400128 ) ) ;
#186990=EDGE_LOOP ( 'NONE', ( #139891, #2559, #173525, #194225, #124473 ) ) ;
#187012=ORIENTED_EDGE ( 'NONE', *, *, #12707, .T. ) ;
#187014=DIRECTION ( 'NONE',  ( -0.2079116908177593703, 0.000000000000000000, 0.9781476007338056888 ) ) ;
#187024=FACE_OUTER_BOUND ( 'NONE', #41314, .T. ) ;
#187026=CARTESIAN_POINT ( 'NONE',  ( 9.498884310698274547, -9.900000000000076739, -0.1658036423890195676 ) ) ;
#187047=ORIENTED_EDGE ( 'NONE', *, *, #4172, .F. ) ;
#187065=AXIS2_PLACEMENT_3D ( 'NONE', #94046, #59385, #9567 ) ;
#187077=ORIENTED_EDGE ( 'NONE', *, *, #180630, .F. ) ;
#187130=VERTEX_POINT ( 'NONE', #163323 ) ;
#187172=CARTESIAN_POINT ( 'NONE',  ( 10.91804383151480806, -9.907361309732431565, -0.1905751639681794174 ) ) ;
#187176=CARTESIAN_POINT ( 'NONE',  ( -8.002408263930261612, -6.836568542494980250, 7.346809171966449448 ) ) ;
#187200=CARTESIAN_POINT ( 'NONE',  ( 0.01979922387977678389, -6.863887327018420415, -9.496663239506007770 ) ) ;
#187212=CARTESIAN_POINT ( 'NONE',  ( 0.01154776750823807881, -8.267087321559200674, 11.00021059652653754 ) ) ;
#187272=DIRECTION ( 'NONE',  ( 1.000000000000000000, -1.084202172485501594E-14, 0.000000000000000000 ) ) ;
#187278=TOROIDAL_SURFACE ( 'NONE', #80129, 10.92000000000000171, 0.08000000000000000167 ) ;
#187280=CIRCLE ( 'NONE', #45532, 0.08000000000000020983 ) ;
#187284=VERTEX_POINT ( 'NONE', #122125 ) ;
#187296=CARTESIAN_POINT ( 'NONE',  ( -10.96027417533446346, -7.850147675656140578, 0.3662874062585462220 ) ) ;
#187303=DIRECTION ( 'NONE',  ( 0.000000000000000000, -1.000000000000000000, 0.000000000000000000 ) ) ;
#187327=CARTESIAN_POINT ( 'NONE',  ( -10.38813158755799471, 2.629643693813620065, -6.007251501586706510 ) ) ;
#187378=EDGE_LOOP ( 'NONE', ( #162917, #91034, #3175, #71258, #121910 ) ) ;
#187379=DIRECTION ( 'NONE',  ( 0.000000000000000000, 0.000000000000000000, 1.000000000000000000 ) ) ;
#187477=EDGE_CURVE ( 'NONE', #107724, #184758, #120563, .T. ) ;
#187503=CARTESIAN_POINT ( 'NONE',  ( -7.806953216197586087, -6.479141885268315804, -7.749822179018686974 ) ) ;
#187539=EDGE_LOOP ( 'NONE', ( #186652, #33466, #83141, #174267 ) ) ;
#187569=DIRECTION ( 'NONE',  ( -0.7408284471490506062, -1.804614770759877281E-12, 0.6716942845482062330 ) ) ;
#187574=CARTESIAN_POINT ( 'NONE',  ( 6.594971855056625643, -6.631671885544809797, 6.818239715405312040 ) ) ;
#187619=CARTESIAN_POINT ( 'NONE',  ( -0.1588445005388229581, -6.630981418884854151, -9.484513308955760280 ) ) ;
#187671=CARTESIAN_POINT ( 'NONE',  ( 0.01181297548617449289, -7.619382996155831478, -9.500232605409566489 ) ) ;
#187676=CIRCLE ( 'NONE', #869, 10.86343145750506878 ) ;
#187677=EDGE_CURVE ( 'NONE', #179385, #51705, #153789, .T. ) ;
#187696=EDGE_CURVE ( 'NONE', #195818, #10241, #99761, .T. ) ;
#187698=DIRECTION ( 'NONE',  ( 0.9998476951563912696, -0.000000000000000000, -0.01745240643728004568 ) ) ;
#187798=CARTESIAN_POINT ( 'NONE',  ( -10.98997987423604172, -6.893137084989842123, 0.4694063952341877011 ) ) ;
#187815=ORIENTED_EDGE ( 'NONE', *, *, #102432, .T. ) ;
#187821=ORIENTED_EDGE ( 'NONE', *, *, #75342, .T. ) ;
#187836=FACE_OUTER_BOUND ( 'NONE', #73946, .T. ) ;
#187846=CARTESIAN_POINT ( 'NONE',  ( 0.000000000000000000, 1.000000000000000888, -12.00000000000000178 ) ) ;
#187872=CARTESIAN_POINT ( 'NONE',  ( 0.000000000000000000, 0.000000000000000000, 0.000000000000000000 ) ) ;
#187916=CARTESIAN_POINT ( 'NONE',  ( 9.586610838029415049, -7.161464053357574855, -0.003376046620562692113 ) ) ;
#187963=EDGE_CURVE ( 'NONE', #187284, #168636, #204595, .T. ) ;
#187970=PRESENTATION_STYLE_ASSIGNMENT (( #8158 ) ) ;
#187987=CARTESIAN_POINT ( 'NONE',  ( -9.499701791763566661, -9.918130724412307586, 0.07530116296179305280 ) ) ;
#188023=CARTESIAN_POINT ( 'NONE',  ( -2.937463097380563013E-12, -7.034525084947490292, -10.67552547708197608 ) ) ;
#188030=CARTESIAN_POINT ( 'NONE',  ( -6.661184041420952440, -7.246166700180828535, 6.773376349083140013 ) ) ;
#188046=CARTESIAN_POINT ( 'NONE',  ( -10.91877977293360047, -9.985078020775008056, 0.1443118549625500291 ) ) ;
#188053=LINE ( 'NONE', #26628, #205626 ) ;
#188060=CARTESIAN_POINT ( 'NONE',  ( 2.044581833100483692, 2.972657967446784788, -11.47952151275210930 ) ) ;
#188079=CARTESIAN_POINT ( 'NONE',  ( 9.499562802171208631, -9.415754203682769941, -0.1226201807150868461 ) ) ;
#188096=AXIS2_PLACEMENT_3D ( 'NONE', #164963, #196406, #62142 ) ;
#188097=EDGE_CURVE ( 'NONE', #94442, #205391, #133156, .T. ) ;
#188122=CARTESIAN_POINT ( 'NONE',  ( 11.24798771954521293, -6.442483420751878853, -0.4630894006630673077 ) ) ;
#188156=ORIENTED_EDGE ( 'NONE', *, *, #208257, .T. ) ;
#188171=CARTESIAN_POINT ( 'NONE',  ( 0.02903434592765696126, -5.609732095436333665, 10.94445979172680516 ) ) ;
#188203=CARTESIAN_POINT ( 'NONE',  ( 0.000000000000000000, 15.50000000000019362, 0.000000000000000000 ) ) ;
#188204=EDGE_CURVE ( 'NONE', #115124, #142909, #67329, .T. ) ;
#188231=ORIENTED_EDGE ( 'NONE', *, *, #133268, .F. ) ;
#188235=SURFACE_SIDE_STYLE ('',( #26805 ) ) ;
#188236=FILL_AREA_STYLE_COLOUR ( '', #189227 ) ;
#188249=CARTESIAN_POINT ( 'NONE',  ( -6.783773228136968036, -6.684699857435323800, 6.634380643896202301 ) ) ;
#188274=CARTESIAN_POINT ( 'NONE',  ( -9.496893780459334522, -9.200036371099116650, 0.2463816395386524416 ) ) ;
#188277=CARTESIAN_POINT ( 'NONE',  ( -0.08202876420372198774, -7.861065518611666469, 10.99977341864973468 ) ) ;
#188320=CARTESIAN_POINT ( 'NONE',  ( 0.000000000000000000, 3.499999999999989342, 0.000000000000000000 ) ) ;
#188344=CARTESIAN_POINT ( 'NONE',  ( -6.953912913643675253, -8.144978210217285408, 6.511381374296902891 ) ) ;
#188352=EDGE_CURVE ( 'NONE', #193389, #72609, #160908, .T. ) ;
#188385=CARTESIAN_POINT ( 'NONE',  ( 0.09999999999999592548, -9.919999999999998153, 10.91954211494236660 ) ) ;
#188393=CARTESIAN_POINT ( 'NONE',  ( 6.773846765307952822, -7.473374494058216300, -6.773846765307982132 ) ) ;
#188403=CARTESIAN_POINT ( 'NONE',  ( 0.4366703603831034175, -8.283751815806033036, -10.40709768291843673 ) ) ;
#188418=DIRECTION ( 'NONE',  ( 0.000000000000000000, 0.000000000000000000, -1.000000000000000000 ) ) ;
#188428=EDGE_LOOP ( 'NONE', ( #93075, #7195, #42192, #127072 ) ) ;
#188471=B_SPLINE_CURVE_WITH_KNOTS ( 'NONE', 3,
 ( #57378, #39000, #123542, #7539, #204666, #73623, #43284 ),
 .UNSPECIFIED., .F., .F.,
 ( 4, 3, 4 ),
 ( 3.315837474970997266E-05, 0.0009000000035470257127, 0.001929259801299054245 ),
 .UNSPECIFIED. ) ;
#188500=ORIENTED_EDGE ( 'NONE', *, *, #89525, .F. ) ;
#188521=EDGE_CURVE ( 'NONE', #146898, #109724, #83999, .T. ) ;
#188527=CARTESIAN_POINT ( 'NONE',  ( -7.720982915750198572, -5.743759731405759794, 7.834948807407328353 ) ) ;
#188542=AXIS2_PLACEMENT_3D ( 'NONE', #111928, #177929, #80418 ) ;
#188568=( GEOMETRIC_REPRESENTATION_CONTEXT ( 3 ) GLOBAL_UNCERTAINTY_ASSIGNED_CONTEXT ( ( #116084 ) ) GLOBAL_UNIT_ASSIGNED_CONTEXT ( ( #11767, #51759, #66887 ) ) REPRESENTATION_CONTEXT ( 'NONE', 'WORKASPACE' ) );
#188569=CARTESIAN_POINT ( 'NONE',  ( -7.664865541497347223, -5.787795860784272328, 7.047292192038678849 ) ) ;
#188592=DIRECTION ( 'NONE',  ( 0.000000000000000000, -1.000000000000000000, 0.000000000000000000 ) ) ;
#188604=CARTESIAN_POINT ( 'NONE',  ( 6.844216539294127877, -8.074889850123396329, -6.588752024304540988 ) ) ;
#188606=CYLINDRICAL_SURFACE ( 'NONE', #113158, 0.07999999999999993228 ) ;
#188627=DIRECTION ( 'NONE',  ( 0.000000000000000000, 1.000000000000000000, 0.000000000000000000 ) ) ;
#188647=CARTESIAN_POINT ( 'NONE',  ( 0.1738264060025629942, -9.190401220100138602, -9.624818503329224839 ) ) ;
#188739=( NAMED_UNIT ( * ) PLANE_ANGLE_UNIT ( ) SI_UNIT ( $, .RADIAN. ) );
#188759=CIRCLE ( 'NONE', #36602, 0.08000000000000020983 ) ;
#188803=B_SPLINE_CURVE_WITH_KNOTS ( 'NONE', 3,
 ( #137628, #20634, #37979, #69381, #166919, #135489, #86723 ),
 .UNSPECIFIED., .F., .F.,
 ( 4, 3, 4 ),
 ( 0.0001126021369358736141, 0.001495765174703651314, 0.002006790696433096571 ),
 .UNSPECIFIED. ) ;
#188804=CARTESIAN_POINT ( 'NONE',  ( -8.280982047128215839, -6.442483420143127582, 7.626074736120322051 ) ) ;
#188810=DIRECTION ( 'NONE',  ( -0.8660254037844433705, 0.000000000000000000, -0.4999999999999917843 ) ) ;
#188812=EDGE_CURVE ( 'NONE', #74995, #50845, #95065, .T. ) ;
#188818=CARTESIAN_POINT ( 'NONE',  ( -6.773846765317315999, -7.246166700180828535, 6.773846765317339091 ) ) ;
#188837=DIRECTION ( 'NONE',  ( 0.000000000000000000, 0.000000000000000000, -1.000000000000000000 ) ) ;
#188865=LINE ( 'NONE', #6890, #66137 ) ;
#188895=CARTESIAN_POINT ( 'NONE',  ( 7.720011280421983813, -5.361065518611646041, 7.836017471263537537 ) ) ;
#188935=DIRECTION ( 'NONE',  ( 0.000000000000000000, 0.000000000000000000, 1.000000000000000000 ) ) ;
#188944=CARTESIAN_POINT ( 'NONE',  ( 9.488641820551102057, -8.233137084989836652, -0.4644097342743017665 ) ) ;
#188975=EDGE_CURVE ( 'NONE', #60692, #162811, #91667, .T. ) ;
#189023=COLOUR_RGB ( '', 0.72549020, 0.75294118, 0.79215686) ;
#189032=EDGE_CURVE ( 'NONE', #54631, #93709, #119379, .T. ) ;
#189045=EDGE_LOOP ( 'NONE', ( #39239, #208806, #136578, #93812 ) ) ;
#189083=CARTESIAN_POINT ( 'NONE',  ( 6.455298931196946199, -8.176227052203557832, 7.002681350352347067 ) ) ;
#189092=( GEOMETRIC_REPRESENTATION_CONTEXT ( 3 ) GLOBAL_UNCERTAINTY_ASSIGNED_CONTEXT ( ( #24913 ) ) GLOBAL_UNIT_ASSIGNED_CONTEXT ( ( #170060, #39010, #184174 ) ) REPRESENTATION_CONTEXT ( 'NONE', 'WORKASPACE' ) );
#189110=DIRECTION ( 'NONE',  ( 0.000000000000000000, -1.000000000000000000, 0.000000000000000000 ) ) ;
#189116=CARTESIAN_POINT ( 'NONE',  ( 8.867053104062428304, 4.021557182957047338, 7.983930475901377832 ) ) ;
#189119=ORIENTED_EDGE ( 'NONE', *, *, #115265, .T. ) ;
#189134=( NAMED_UNIT ( * ) SI_UNIT ( $, .STERADIAN. ) SOLID_ANGLE_UNIT ( ) );
#189145=ORIENTED_EDGE ( 'NONE', *, *, #151210, .F. ) ;
#189170=CARTESIAN_POINT ( 'NONE',  ( -0.3866937364864243554, 3.956598013261175772, 11.53692321988874170 ) ) ;
#189174=SURFACE_STYLE_USAGE ( .BOTH. , #155615 ) ;
#189199=CARTESIAN_POINT ( 'NONE',  ( -6.825879202496262899, -6.900108348305959538, 6.758184431511289780 ) ) ;
#189221=DIRECTION ( 'NONE',  ( 0.000000000000000000, 1.000000000000000000, 0.000000000000000000 ) ) ;
#189227=COLOUR_RGB ( '', 0.31764706, 0.68627451, 0.89019608) ;
#189233=VERTEX_POINT ( 'NONE', #53033 ) ;
#189305=CARTESIAN_POINT ( 'NONE',  ( -10.99663476780025206, -7.859187537802515777, 0.2753234695294815570 ) ) ;
#189331=EDGE_CURVE ( 'NONE', #209328, #17507, #5170, .T. ) ;
#189352=FACE_OUTER_BOUND ( 'NONE', #40446, .T. ) ;
#189357=CARTESIAN_POINT ( 'NONE',  ( -0.1305260785387524214, -7.912329794880667677, 10.96023284214815163 ) ) ;
#189408=CARTESIAN_POINT ( 'NONE',  ( 7.827294160508029286, -6.717993526550377403, -7.547439985188189482 ) ) ;
#189426=CARTESIAN_POINT ( 'NONE',  ( -6.855650617048436146, -7.357813805523307771, 6.855650617048461015 ) ) ;
#189438=( LENGTH_UNIT ( ) NAMED_UNIT ( * ) SI_UNIT ( .MILLI., .METRE. ) );
#189465=CARTESIAN_POINT ( 'NONE',  ( 0.1236583036082015280, 1.000000000000000888, -11.99936284241577233 ) ) ;
#189525=DIRECTION ( 'NONE',  ( 0.000000000000000000, 0.000000000000000000, 1.000000000000000000 ) ) ;
#189531=ORIENTED_EDGE ( 'NONE', *, *, #46711, .T. ) ;
#189553=ORIENTED_EDGE ( 'NONE', *, *, #203402, .F. ) ;
#189582=CARTESIAN_POINT ( 'NONE',  ( 3.241898903847886913E-13, -7.217880409008443188, -9.581975256308904676 ) ) ;
#189594=CARTESIAN_POINT ( 'NONE',  ( -0.1523027874135017556, -6.731960136058439126, -9.611344009005488687 ) ) ;
#189629=ORIENTED_EDGE ( 'NONE', *, *, #170125, .F. ) ;
#189635=CARTESIAN_POINT ( 'NONE',  ( 9.926723642588102692, -7.126685749119995528, 1.734723475976807094E-15 ) ) ;
#189647=DIRECTION ( 'NONE',  ( 0.000000000000000000, 0.000000000000000000, 1.000000000000000000 ) ) ;
#189656=DIRECTION ( 'NONE',  ( 0.000000000000000000, 0.000000000000000000, -1.000000000000000000 ) ) ;
#189669=CARTESIAN_POINT ( 'NONE',  ( 2.075332711124678653, 1.720726420432414860, -11.62496126974820143 ) ) ;
#189670=ORIENTED_EDGE ( 'NONE', *, *, #3623, .F. ) ;
#189679=FACE_OUTER_BOUND ( 'NONE', #8924, .T. ) ;
#189681=ADVANCED_FACE ( 'NONE', ( #110390, #93029 ), #6397, .T. ) ;
#189690=CARTESIAN_POINT ( 'NONE',  ( 0.000000000000000000, 4.000000000000003553, 0.000000000000000000 ) ) ;
#189732=EDGE_CURVE ( 'NONE', #144836, #74967, #5306, .T. ) ;
#189743=ORIENTED_EDGE ( 'NONE', *, *, #101693, .T. ) ;
#189788=ORIENTED_EDGE ( 'NONE', *, *, #35599, .T. ) ;
#189811=CARTESIAN_POINT ( 'NONE',  ( 2.032879073410320814E-16, -7.473374494045017968, -9.579665964948882007 ) ) ;
#189846=CARTESIAN_POINT ( 'NONE',  ( 0.4294425147611385940, -9.006862915010128035, -9.490288674561771387 ) ) ;
#189856=VERTEX_POINT ( 'NONE', #155879 ) ;
#189866=CARTESIAN_POINT ( 'NONE',  ( 11.68720892159067937, 1.016282880930320598, -3.797404372613902179 ) ) ;
#189869=AXIS2_PLACEMENT_3D ( 'NONE', #53233, #36973, #197343 ) ;
#189874=SURFACE_SIDE_STYLE ('',( #124965 ) ) ;
#189880=CARTESIAN_POINT ( 'NONE',  ( 7.460470246983015308, -6.805008568744152164, 7.900729602272511976 ) ) ;
#189933=ORIENTED_EDGE ( 'NONE', *, *, #87853, .F. ) ;
#189941=ORIENTED_EDGE ( 'NONE', *, *, #184591, .F. ) ;
#189954=EDGE_LOOP ( 'NONE', ( #207057, #48919, #56750, #66907 ) ) ;
#189975=CARTESIAN_POINT ( 'NONE',  ( -0.07538891330675720481, -7.154544010627095219, 9.499700864329915007 ) ) ;
#190007=VECTOR ( 'NONE', #152513, 1000.000000000000227 ) ;
#190034=CARTESIAN_POINT ( 'NONE',  ( -10.87712779691732834, -6.655928102866995211, 0.1480828224388648917 ) ) ;
#190036=CARTESIAN_POINT ( 'NONE',  ( -2.425588855773942676, 2.974000657016653282, 11.41149836408661322 ) ) ;
#190072=SURFACE_SIDE_STYLE ('',( #172778 ) ) ;
#190097=CARTESIAN_POINT ( 'NONE',  ( 1.347111479062087616E-15, -9.999999999999994671, -10.99999999999999112 ) ) ;
#190098=EDGE_CURVE ( 'NONE', #108269, #207703, #176860, .T. ) ;
#190134=CIRCLE ( 'NONE', #48392, 8.049999999999993605 ) ;
#190141=CARTESIAN_POINT ( 'NONE',  ( 6.764898216727350366, -7.628386336122866318, 6.764898216730284020 ) ) ;
#190145=DIRECTION ( 'NONE',  ( 8.881784197001252323E-16, 0.000000000000000000, -1.000000000000000000 ) ) ;
#190168=CARTESIAN_POINT ( 'NONE',  ( -6.661184041420952440, -7.215597533173327527, 6.773376349083140013 ) ) ;
#190182=VERTEX_POINT ( 'NONE', #15984 ) ;
#190196=CARTESIAN_POINT ( 'NONE',  ( 2.505492374191277349, 3.019799309332890314, -11.78741486268894434 ) ) ;
#190200=ORIENTED_EDGE ( 'NONE', *, *, #75043, .F. ) ;
#190225=CARTESIAN_POINT ( 'NONE',  ( -9.537847510268184337, -7.985988503423656404, 0.1421055763938848249 ) ) ;
#190226=CARTESIAN_POINT ( 'NONE',  ( -0.02500845152586464101, 3.700502905159948508, 11.79962023279682271 ) ) ;
#190229=FILL_AREA_STYLE ('',( #89565 ) ) ;
#190252=CARTESIAN_POINT ( 'NONE',  ( 9.765991159990626613, -7.287292132425312374, 9.269928574751062911E-15 ) ) ;
#190265=CARTESIAN_POINT ( 'NONE',  ( -2.791122189554258290E-19, 3.467171072964057910, 11.99762841690770365 ) ) ;
#190275=ORIENTED_EDGE ( 'NONE', *, *, #58624, .F. ) ;
#190285=CARTESIAN_POINT ( 'NONE',  ( 0.03750003396568112046, -9.978860739388867529, 10.91964959838802507 ) ) ;
#190286=ORIENTED_EDGE ( 'NONE', *, *, #110968, .T. ) ;
#190334=VECTOR ( 'NONE', #62369, 1000.000000000000000 ) ;
#190340=CARTESIAN_POINT ( 'NONE',  ( -0.03969736035582727834, -7.921780080556630743, 11.00000000000013145 ) ) ;
#190358=CARTESIAN_POINT ( 'NONE',  ( -10.98676690055265581, -7.666862915010298707, 0.5459353850038998202 ) ) ;
#190365=CARTESIAN_POINT ( 'NONE',  ( -10.10176665042269839, 1.000000000000000888, -6.279211784079198999 ) ) ;
#190367=EDGE_CURVE ( 'NONE', #118273, #55414, #50251, .T. ) ;
#190376=VERTEX_POINT ( 'NONE', #294 ) ;
#190395=DIRECTION ( 'NONE',  ( 0.000000000000000000, 1.000000000000000000, 0.000000000000000000 ) ) ;
#190403=CARTESIAN_POINT ( 'NONE',  ( 0.000000000000000000, -13.99999999999999822, 0.000000000000000000 ) ) ;
#190407=CARTESIAN_POINT ( 'NONE',  ( -0.1826339422288273118, -7.841768514962170755, 10.96557956857094673 ) ) ;
#190428=ORIENTED_EDGE ( 'NONE', *, *, #107850, .T. ) ;
#190447=SURFACE_SIDE_STYLE ('',( #56201 ) ) ;
#190453=CYLINDRICAL_SURFACE ( 'NONE', #101038, 6.249999999999995559 ) ;
#190461=CARTESIAN_POINT ( 'NONE',  ( 7.966449380362733201, -6.654700410849428316, -7.586197045692575358 ) ) ;
#190490=CARTESIAN_POINT ( 'NONE',  ( -0.05513001983272274725, -8.135652870098727618, -11.00000000000013145 ) ) ;
#190504=EDGE_CURVE ( 'NONE', #119302, #55041, #21826, .T. ) ;
#190519=CARTESIAN_POINT ( 'NONE',  ( 0.05470795666945791474, -5.634700952767746962, -11.00000000000002487 ) ) ;
#190523=( GEOMETRIC_REPRESENTATION_CONTEXT ( 3 ) GLOBAL_UNCERTAINTY_ASSIGNED_CONTEXT ( ( #145373 ) ) GLOBAL_UNIT_ASSIGNED_CONTEXT ( ( #180815, #160577, #26297 ) ) REPRESENTATION_CONTEXT ( 'NONE', 'WORKASPACE' ) );
#190556=UNCERTAINTY_MEASURE_WITH_UNIT (LENGTH_MEASURE( 1.000000000000000082E-05 ), #180847, 'distance_accuracy_value', 'NONE');
#190567=FACE_OUTER_BOUND ( 'NONE', #161600, .T. ) ;
#190585=CARTESIAN_POINT ( 'NONE',  ( -0.3663205537283738544, -5.223179855898254509, -10.97093617010719946 ) ) ;
#190633=EDGE_CURVE ( 'NONE', #57699, #131570, #70925, .T. ) ;
#190634=ORIENTED_EDGE ( 'NONE', *, *, #166214, .T. ) ;
#190635=DIRECTION ( 'NONE',  ( 0.000000000000000000, -1.000000000000000000, 0.000000000000000000 ) ) ;
#190642=CARTESIAN_POINT ( 'NONE',  ( 10.39025099420807052, 3.467171072964058354, -5.998814208453958408 ) ) ;
#190661=CARTESIAN_POINT ( 'NONE',  ( 9.555169238417182243, -7.776896528353608673, -0.04234008746931129663 ) ) ;
#190700=CARTESIAN_POINT ( 'NONE',  ( -9.498256814137544524, -6.950186805636726639, -0.04218801535505443956 ) ) ;
#190705=EDGE_CURVE ( 'NONE', #187130, #80718, #19144, .T. ) ;
#190726=ORIENTED_EDGE ( 'NONE', *, *, #175281, .F. ) ;
#190728=ORIENTED_EDGE ( 'NONE', *, *, #135027, .F. ) ;
#190735=SURFACE_STYLE_USAGE ( .BOTH. , #176643 ) ;
#190743=TOROIDAL_SURFACE ( 'NONE', #3937, 10.92000000000000171, 0.08000000000000000167 ) ;
#190746=LINE ( 'NONE', #42410, #129606 ) ;
#190762=EDGE_LOOP ( 'NONE', ( #137824, #86879, #62565, #115638 ) ) ;
#190776=DIRECTION ( 'NONE',  ( 0.000000000000000000, 0.000000000000000000, -1.000000000000000000 ) ) ;
#190825=AXIS2_PLACEMENT_3D ( 'NONE', #141912, #12915, #78995 ) ;
#190826=B_SPLINE_CURVE_WITH_KNOTS ( 'NONE', 3,
 ( #189170, #172942, #24520, #140466, #58109, #190226, #41885, #107996 ),
 .UNSPECIFIED., .F., .F.,
 ( 4, 2, 2, 4 ),
 ( 7.413913665834773066E-18, 0.0002034531274099240334, 0.0004069062548198406400, 0.0008138125096396705465 ),
 .UNSPECIFIED. ) ;
#190832=TOROIDAL_SURFACE ( 'NONE', #163190, 9.559451093910102060, 0.08000000000000000167 ) ;
#190840=CARTESIAN_POINT ( 'NONE',  ( -11.40816717570230310, 3.487142912321092414, 3.706738213303463425 ) ) ;
#190846=ORIENTED_EDGE ( 'NONE', *, *, #207247, .T. ) ;
#190856=ORIENTED_EDGE ( 'NONE', *, *, #75342, .F. ) ;
#190890=EDGE_CURVE ( 'NONE', #96623, #33092, #84824, .T. ) ;
#190920=FILL_AREA_STYLE ('',( #171485 ) ) ;
#190954=CARTESIAN_POINT ( 'NONE',  ( 7.721398836998391246, -5.907420853759296264, 7.721398836998372595 ) ) ;
#191007=EDGE_LOOP ( 'NONE', ( #118185, #171132, #172104, #89582 ) ) ;
#191019=CARTESIAN_POINT ( 'NONE',  ( 1.432836755002402101E-15, 0.7999999999999951594, -11.69999999999999041 ) ) ;
#191044=CARTESIAN_POINT ( 'NONE',  ( 0.08814328694727366353, -9.915773547069447247, 10.99964701288573465 ) ) ;
#191048=CARTESIAN_POINT ( 'NONE',  ( -0.4635785636673758758, -6.836568542495036205, -10.85353573482950829 ) ) ;
#191077=ORIENTED_EDGE ( 'NONE', *, *, #169747, .F. ) ;
#191089=CARTESIAN_POINT ( 'NONE',  ( -11.00029612940780410, -6.479296433800279864, -0.04006801626462446614 ) ) ;
#191091=CARTESIAN_POINT ( 'NONE',  ( -2.480760062148275491, 4.021557182957056220, 11.67105848277438795 ) ) ;
#191130=VECTOR ( 'NONE', #172856, 1000.000000000000000 ) ;
#191143=EDGE_CURVE ( 'NONE', #113279, #207870, #81433, .T. ) ;
#191153=ADVANCED_FACE ( 'NONE', ( #14167 ), #80150, .T. ) ;
#191167=EDGE_LOOP ( 'NONE', ( #205402, #198446, #62938, #661 ) ) ;
#191178=CARTESIAN_POINT ( 'NONE',  ( -0.1007326007325826528, -9.920000000000095852, -10.99953876047305812 ) ) ;
#191197=CARTESIAN_POINT ( 'NONE',  ( 11.21553972792699128, 3.696394713403117649, -3.679259263401860380 ) ) ;
#191201=DIRECTION ( 'NONE',  ( 0.000000000000000000, 0.000000000000000000, 1.000000000000000000 ) ) ;
#191232=SURFACE_STYLE_FILL_AREA ( #40750 ) ;
#191280=CARTESIAN_POINT ( 'NONE',  ( 9.578206935409037115, -9.746166700193986898, -0.1671882239534273895 ) ) ;
#191287=CARTESIAN_POINT ( 'NONE',  ( 9.499606459999014874, -9.910930816046773728, -0.08647025586254107610 ) ) ;
#191306=ORIENTED_EDGE ( 'NONE', *, *, #92980, .T. ) ;
#191337=DIRECTION ( 'NONE',  ( 0.000000000000000000, 0.000000000000000000, 1.000000000000000000 ) ) ;
#191346=CARTESIAN_POINT ( 'NONE',  ( 0.009341426467586660259, -9.943661027227909344, 10.91969313363970251 ) ) ;
#191373=AXIS2_PLACEMENT_3D ( 'NONE', #25384, #156473, #8062 ) ;
#191409=ORIENTED_EDGE ( 'NONE', *, *, #143030, .T. ) ;
#191414=ORIENTED_EDGE ( 'NONE', *, *, #194669, .F. ) ;
#191440=CARTESIAN_POINT ( 'NONE',  ( -6.580818069394661407, -6.606405293530497325, -7.011678565220725190 ) ) ;
#191451=CARTESIAN_POINT ( 'NONE',  ( -0.4382560683119374190, -5.166862915010145052, -10.99126615174919408 ) ) ;
#191468=CARTESIAN_POINT ( 'NONE',  ( -9.622374086701562135, -9.063146643177661943, 0.5328106107931148694 ) ) ;
#191509=CARTESIAN_POINT ( 'NONE',  ( 7.583016927391839523, -5.196967604326695245, 7.968844136639797959 ) ) ;
#191533=CARTESIAN_POINT ( 'NONE',  ( 9.488641820551087847, -8.200000000000001066, -0.4644097342742986578 ) ) ;
#191535=EDGE_LOOP ( 'NONE', ( #74765, #212002, #213100, #132470 ) ) ;
#191538=FACE_OUTER_BOUND ( 'NONE', #202067, .T. ) ;
#191540=CARTESIAN_POINT ( 'NONE',  ( -7.253312916980312330, -6.796015482748900993, 7.253312916980332758 ) ) ;
#191549=FILL_AREA_STYLE ('',( #109330 ) ) ;
#191557=CARTESIAN_POINT ( 'NONE',  ( -7.005920419302424484, -8.176248043969003731, 6.451695228974702268 ) ) ;
#191589=CARTESIAN_POINT ( 'NONE',  ( -0.08058608058608175695, -6.271284633940164888, 10.99970480893082225 ) ) ;
#191645=VERTEX_POINT ( 'NONE', #176191 ) ;
#191672=UNCERTAINTY_MEASURE_WITH_UNIT (LENGTH_MEASURE( 1.000000000000000082E-05 ), #196303, 'distance_accuracy_value', 'NONE');
#191684=EDGE_LOOP ( 'NONE', ( #137554, #170000, #121004, #130327, #145390, #138185 ) ) ;
#191698=ORIENTED_EDGE ( 'NONE', *, *, #159427, .T. ) ;
#191707=ADVANCED_FACE ( 'NONE', ( #27791 ), #140210, .T. ) ;
#191720=( BOUNDED_SURFACE ( )  B_SPLINE_SURFACE ( 3, 2, ( 
 ( #196685, #48324, #114435 ),
 ( #164189, #83980, #181483 ),
 ( #118685, #65579, #33112 ),
 ( #168437, #166305, #132776 ) ),
 .UNSPECIFIED., .F., .F., .T. ) 
 B_SPLINE_SURFACE_WITH_KNOTS ( ( 4, 4 ),
 ( 3, 3 ),
 ( 0.000000000000000000, 9.170893476604520501E-05 ),
 ( 0.000000000000000000, 1.000000000000000000 ),
 .UNSPECIFIED. ) 
 GEOMETRIC_REPRESENTATION_ITEM ( )  RATIONAL_B_SPLINE_SURFACE ( (
 ( 1.000000000000000000, 0.7100530722026773267, 1.000000000000000000),
 ( 1.000000000000000000, 0.6998898451682598054, 1.000000000000000000),
 ( 1.000000000000000000, 0.6894756946157374333, 1.000000000000000000),
 ( 1.000000000000000000, 0.6787756258918233865, 1.000000000000000000) ) ) 
 REPRESENTATION_ITEM ( '' )  SURFACE ( )  );
#191759=EDGE_LOOP ( 'NONE', ( #25987, #212066, #165678, #189941 ) ) ;
#191792=FACE_OUTER_BOUND ( 'NONE', #171035, .T. ) ;
#191798=CARTESIAN_POINT ( 'NONE',  ( -10.98633066092102872, -7.699791778944246268, 0.5535395452644350511 ) ) ;
#191803=AXIS2_PLACEMENT_3D ( 'NONE', #211546, #96781, #51202 ) ;
#191931=CARTESIAN_POINT ( 'NONE',  ( -10.91944002402978775, -8.407420853759269619, 0.1905873483556677628 ) ) ;
#191954=VERTEX_POINT ( 'NONE', #14720 ) ;
#191962=B_SPLINE_CURVE_WITH_KNOTS ( 'NONE', 3,
 ( #26840, #27916, #11655, #63616 ),
 .UNSPECIFIED., .F., .F.,
 ( 4, 4 ),
 ( 0.000000000000000000, 0.0002908967400263861051 ),
 .UNSPECIFIED. ) ;
#192011=CARTESIAN_POINT ( 'NONE',  ( -0.01492041558615165263, -9.953728265215222137, -10.91968477554607730 ) ) ;
#192050=ORIENTED_EDGE ( 'NONE', *, *, #87853, .T. ) ;
#192073=ORIENTED_EDGE ( 'NONE', *, *, #96073, .F. ) ;
#192082=PLANE ( 'NONE',  #53787 ) ;
#192107=( GEOMETRIC_REPRESENTATION_CONTEXT ( 3 ) GLOBAL_UNCERTAINTY_ASSIGNED_CONTEXT ( ( #100335 ) ) GLOBAL_UNIT_ASSIGNED_CONTEXT ( ( #107185, #125589, #156952 ) ) REPRESENTATION_CONTEXT ( 'NONE', 'WORKASPACE' ) );
#192114=CARTESIAN_POINT ( 'NONE',  ( -0.4652101495396395725, -7.972382850425336009, -9.716492259128731490 ) ) ;
#192159=B_SPLINE_CURVE_WITH_KNOTS ( 'NONE', 3,
 ( #80791, #160977, #129624, #81844, #65564, #94928, #14696, #213943, #131711, #127499 ),
 .UNSPECIFIED., .F., .F.,
 ( 4, 2, 2, 2, 4 ),
 ( 0.000000000000000000, 0.0002216178067634644539, 0.0004432356135269289077, 0.0006648534202903933887, 0.0008864712270538578154 ),
 .UNSPECIFIED. ) ;
#192211=CARTESIAN_POINT ( 'NONE',  ( -0.08359363160203592269, -9.910747646673586431, -10.99968245379460186 ) ) ;
#192281=CARTESIAN_POINT ( 'NONE',  ( 10.49201538390852129, 0.9691415390508777428, -5.610609371109157806 ) ) ;
#192294=PRESENTATION_STYLE_ASSIGNMENT (( #91649 ) ) ;
#192298=ORIENTED_EDGE ( 'NONE', *, *, #54326, .F. ) ;
#192304=ORIENTED_EDGE ( 'NONE', *, *, #27811, .F. ) ;
#192315=CARTESIAN_POINT ( 'NONE',  ( 2.020417662918754687, 3.956598013261175772, -11.36521191596581737 ) ) ;
#192316=AXIS2_PLACEMENT_3D ( 'NONE', #25070, #91172, #74903 ) ;
#192339=CARTESIAN_POINT ( 'NONE',  ( -0.09510031644103759951, -6.698521824825871107, -10.99968117833243042 ) ) ;
#192346=CARTESIAN_POINT ( 'NONE',  ( 9.622669940282555956, -9.063128755109502777, -0.5283818209470574345 ) ) ;
#192381=CARTESIAN_POINT ( 'NONE',  ( 10.66594405399933976, -7.024005795609692626, -0.4637852190794419793 ) ) ;
#192418=CARTESIAN_POINT ( 'NONE',  ( 0.07538891330674882263, -7.154544010627095219, -9.499700864329891914 ) ) ;
#192461=B_SPLINE_CURVE_WITH_KNOTS ( 'NONE', 3,
 ( #148118, #181652, #20217, #136136, #151317, #202152, #67879, #50598 ),
 .UNSPECIFIED., .F., .F.,
 ( 4, 2, 2, 4 ),
 ( 5.963111948670136683E-19, 0.0002224730689913816681, 0.0004449461379827627399, 0.0008898922759655248293 ),
 .UNSPECIFIED. ) ;
#192481=VERTEX_POINT ( 'NONE', #20883 ) ;
#192490=CARTESIAN_POINT ( 'NONE',  ( 0.000000000000000000, 0.7999999999999951594, -11.50000000000000000 ) ) ;
#192497=ADVANCED_FACE ( 'NONE', ( #38236 ), #60858, .T. ) ;
#192533=CARTESIAN_POINT ( 'NONE',  ( -9.603221262331047114, -9.439766061754902182, 0.1988025308400011015 ) ) ;
#192559=AXIS2_PLACEMENT_3D ( 'NONE', #75519, #123302, #23545 ) ;
#192573=FILL_AREA_STYLE_COLOUR ( '', #50250 ) ;
#192579=DIRECTION ( 'NONE',  ( 0.000000000000000000, 1.000000000000000000, 0.000000000000000000 ) ) ;
#192624=CARTESIAN_POINT ( 'NONE',  ( -6.773846765316610785, -7.473374494057217987, 6.773846765316634766 ) ) ;
#192645=CARTESIAN_POINT ( 'NONE',  ( 0.3870735955438693310, 1.000000000000000888, -11.88799243440807274 ) ) ;
#192659=CARTESIAN_POINT ( 'NONE',  ( -11.09544190643409678, 2.974000657017215055, 3.605127613804370412 ) ) ;
#192689=CARTESIAN_POINT ( 'NONE',  ( -0.08000000000000714873, -6.134628647623513231, 10.91970695577494865 ) ) ;
#192695=CARTESIAN_POINT ( 'NONE',  ( 0.000000000000000000, -8.233137084989836652, 0.000000000000000000 ) ) ;
#192701=CARTESIAN_POINT ( 'NONE',  ( 8.064677165291193717, -5.223431457505076203, -7.446209719563348983 ) ) ;
#192703=CARTESIAN_POINT ( 'NONE',  ( 6.776370306708061619, -7.161464053357560644, 6.781144757626056396 ) ) ;
#192726=SURFACE_STYLE_FILL_AREA ( #63810 ) ;
#192750=ORIENTED_EDGE ( 'NONE', *, *, #152940, .T. ) ;
#192753=CIRCLE ( 'NONE', #9398, 0.08000000000000020983 ) ;
#192792=CARTESIAN_POINT ( 'NONE',  ( -0.07933194154488912297, -7.473374494045017968, 9.499668754385634628 ) ) ;
#192794=DIRECTION ( 'NONE',  ( -0.000000000000000000, -1.000000000000000000, -0.000000000000000000 ) ) ;
#192810=ADVANCED_FACE ( 'NONE', ( #111563 ), #20668, .T. ) ;
#192823=CARTESIAN_POINT ( 'NONE',  ( 7.834948825496932834, -5.907420853759296264, 7.720982897393586342 ) ) ;
#192831=PLANE ( 'NONE',  #205182 ) ;
#192837=LINE ( 'NONE', #78035, #172845 ) ;
#192853=CARTESIAN_POINT ( 'NONE',  ( 6.717278222822382183, 7.849261790823902629, -6.750415307812251520 ) ) ;
#192862=VERTEX_POINT ( 'NONE', #138956 ) ;
#192899=CARTESIAN_POINT ( 'NONE',  ( -1.040834085586084257E-14, -9.746166700180788567, -9.579665964948867796 ) ) ;
#192908=ADVANCED_FACE ( 'NONE', ( #4660 ), #35869, .F. ) ;
#192913=DIRECTION ( 'NONE',  ( 0.000000000000000000, 1.000000000000000000, 0.000000000000000000 ) ) ;
#192924=CARTESIAN_POINT ( 'NONE',  ( -2.290347054751606493, 1.000000000000000888, 11.71088463649534717 ) ) ;
#192932=CARTESIAN_POINT ( 'NONE',  ( -7.720011280421934963, -5.361065518611648706, -7.836017471263586387 ) ) ;
#192938=EDGE_CURVE ( 'NONE', #74349, #177991, #133563, .T. ) ;
#192946=CARTESIAN_POINT ( 'NONE',  ( 10.99970480893080627, -5.907420853759282053, 0.08058608058608522640 ) ) ;
#192965=ORIENTED_EDGE ( 'NONE', *, *, #122755, .F. ) ;
#192970=VECTOR ( 'NONE', #181082, 1000.000000000000000 ) ;
#192988=UNCERTAINTY_MEASURE_WITH_UNIT (LENGTH_MEASURE( 1.000000000000000082E-05 ), #110478, 'distance_accuracy_value', 'NONE');
#192990=DIRECTION ( 'NONE',  ( -1.000000000000000000, -1.561251128379122346E-12, 0.000000000000000000 ) ) ;
#193058=B_SPLINE_CURVE_WITH_KNOTS ( 'NONE', 3,
 ( #174320, #141841, #191589, #90931 ),
 .UNSPECIFIED., .F., .F.,
 ( 4, 4 ),
 ( 0.0006294919072214776642, 0.001039439579420692490 ),
 .UNSPECIFIED. ) ;
#193092=( NAMED_UNIT ( * ) PLANE_ANGLE_UNIT ( ) SI_UNIT ( $, .RADIAN. ) );
#193102=SURFACE_SIDE_STYLE ('',( #214365 ) ) ;
#193127=VERTEX_POINT ( 'NONE', #189846 ) ;
#193183=CARTESIAN_POINT ( 'NONE',  ( 7.664865541498710577, -5.787795860784239466, -7.047292192037250658 ) ) ;
#193316=VERTEX_POINT ( 'NONE', #166960 ) ;
#193327=CYLINDRICAL_SURFACE ( 'NONE', #35515, 0.07999999999999993228 ) ;
#193367=CARTESIAN_POINT ( 'NONE',  ( 0.000000000000000000, -2.079999999999998295, 0.000000000000000000 ) ) ;
#193383=ORIENTED_EDGE ( 'NONE', *, *, #84110, .F. ) ;
#193389=VERTEX_POINT ( 'NONE', #52135 ) ;
#193438=EDGE_LOOP ( 'NONE', ( #57294, #155087, #132907, #155019, #206577 ) ) ;
#193505=FACE_OUTER_BOUND ( 'NONE', #194223, .T. ) ;
#193531=AXIS2_PLACEMENT_3D ( 'NONE', #201007, #150173, #117726 ) ;
#193539=ORIENTED_EDGE ( 'NONE', *, *, #164125, .T. ) ;
#193549=CARTESIAN_POINT ( 'NONE',  ( -8.736946208889554263E-14, -8.872104535001076542, 9.837524982414052488 ) ) ;
#193571=DIRECTION ( 'NONE',  ( 0.000000000000000000, -1.084202172485501594E-14, -1.000000000000000000 ) ) ;
#193661=ORIENTED_EDGE ( 'NONE', *, *, #128877, .T. ) ;
#193673=CARTESIAN_POINT ( 'NONE',  ( 9.488641820551089623, -8.233137084989849086, -0.4644097342742991019 ) ) ;
#193690=CARTESIAN_POINT ( 'NONE',  ( 0.08058608058607655278, -8.270571484000479145, 10.99970480893082225 ) ) ;
#193700=ORIENTED_EDGE ( 'NONE', *, *, #186547, .F. ) ;
#193717=CARTESIAN_POINT ( 'NONE',  ( -1.938011383317839176E-15, -8.407420853759283830, -10.91970695577494865 ) ) ;
#193774=EDGE_LOOP ( 'NONE', ( #199763, #46120, #27075, #157153 ) ) ;
#193781=CARTESIAN_POINT ( 'NONE',  ( 6.775478006741583847, -7.217909409563576517, 6.775478006741560755 ) ) ;
#193788=CARTESIAN_POINT ( 'NONE',  ( -8.855744143575682514, 3.691791674785632082, -7.453352967675195728 ) ) ;
#193808=DIRECTION ( 'NONE',  ( 0.000000000000000000, 1.000000000000000000, 0.000000000000000000 ) ) ;
#193825=ORIENTED_EDGE ( 'NONE', *, *, #128394, .F. ) ;
#193930=CARTESIAN_POINT ( 'NONE',  ( 7.834948813061768824, -6.306565840633488129, 7.720982910012296863 ) ) ;
#193933=EDGE_LOOP ( 'NONE', ( #177703, #44482, #163740, #95561 ) ) ;
#193946=ORIENTED_EDGE ( 'NONE', *, *, #109273, .T. ) ;
#193957=CARTESIAN_POINT ( 'NONE',  ( -9.499668754385638181, -7.246166700194470067, -0.07933194154487506478 ) ) ;
#193959=DIRECTION ( 'NONE',  ( 0.000000000000000000, 1.000000000000000000, 0.000000000000000000 ) ) ;
#194003=CARTESIAN_POINT ( 'NONE',  ( -7.573156686838094842, -5.230039540835550227, -7.978162878861462914 ) ) ;
#194036=FACE_OUTER_BOUND ( 'NONE', #85917, .T. ) ;
#194070=ORIENTED_EDGE ( 'NONE', *, *, #67908, .T. ) ;
#194072=DIRECTION ( 'NONE',  ( -0.9992060137953822085, -9.538978360076122062E-16, -0.03984146075563014394 ) ) ;
#194076=EDGE_CURVE ( 'NONE', #24478, #161735, #153438, .T. ) ;
#194102=VERTEX_POINT ( 'NONE', #89984 ) ;
#194126=CARTESIAN_POINT ( 'NONE',  ( 10.91970695577495043, -6.134628647623513231, 5.204170427930421283E-15 ) ) ;
#194158=SURFACE_STYLE_USAGE ( .BOTH. , #13277 ) ;
#194161=FILL_AREA_STYLE_COLOUR ( '', #40925 ) ;
#194189=( GEOMETRIC_REPRESENTATION_CONTEXT ( 3 ) GLOBAL_UNCERTAINTY_ASSIGNED_CONTEXT ( ( #150171 ) ) GLOBAL_UNIT_ASSIGNED_CONTEXT ( ( #7069, #3861, #136046 ) ) REPRESENTATION_CONTEXT ( 'NONE', 'WORKASPACE' ) );
#194223=EDGE_LOOP ( 'NONE', ( #86288, #4241, #69779 ) ) ;
#194225=ORIENTED_EDGE ( 'NONE', *, *, #205728, .F. ) ;
#194233=EDGE_LOOP ( 'NONE', ( #181147, #100153 ) ) ;
#194244=FACE_OUTER_BOUND ( 'NONE', #132143, .T. ) ;
#194276=CYLINDRICAL_SURFACE ( 'NONE', #130205, 0.07999999999999993228 ) ;
#194303=ADVANCED_FACE ( 'NONE', ( #158178 ), #105171, .F. ) ;
#194305=( GEOMETRIC_REPRESENTATION_CONTEXT ( 3 ) GLOBAL_UNCERTAINTY_ASSIGNED_CONTEXT ( ( #190556 ) ) GLOBAL_UNIT_ASSIGNED_CONTEXT ( ( #180847, #107662, #158483 ) ) REPRESENTATION_CONTEXT ( 'NONE', 'WORKASPACE' ) );
#194334=ORIENTED_EDGE ( 'NONE', *, *, #53547, .F. ) ;
#194395=DIRECTION ( 'NONE',  ( -0.000000000000000000, 1.000000000000000000, -0.000000000000000000 ) ) ;
#194459=AXIS2_PLACEMENT_3D ( 'NONE', #24941, #190635, #125737 ) ;
#194464=CARTESIAN_POINT ( 'NONE',  ( 0.3866937364864087567, 3.956598013261175772, -11.53692321988872926 ) ) ;
#194477=ORIENTED_EDGE ( 'NONE', *, *, #163321, .F. ) ;
#194531=CARTESIAN_POINT ( 'NONE',  ( -7.720982897393583677, -5.907420853759296264, 7.834948825496934610 ) ) ;
#194541=CIRCLE ( 'NONE', #156531, 10.99999999999999112 ) ;
#194558=VERTEX_POINT ( 'NONE', #33097 ) ;
#194562=DIRECTION ( 'NONE',  ( 0.000000000000000000, 1.000000000000000000, 0.000000000000000000 ) ) ;
#194608=SURFACE_STYLE_FILL_AREA ( #139489 ) ;
#194642=AXIS2_PLACEMENT_3D ( 'NONE', #103140, #151898, #115187 ) ;
#194659=CARTESIAN_POINT ( 'NONE',  ( 0.000000000000000000, -6.893137084989842123, 0.000000000000000000 ) ) ;
#194669=EDGE_CURVE ( 'NONE', #174410, #36083, #192159, .T. ) ;
#194681=ADVANCED_FACE ( 'NONE', ( #147927 ), #71899, .F. ) ;
#194704=EDGE_CURVE ( 'NONE', #186393, #15455, #185459, .T. ) ;
#194706=SURFACE_STYLE_FILL_AREA ( #33268 ) ;
#194729=CARTESIAN_POINT ( 'NONE',  ( 7.778383330260338013, -6.134628647623489250, -7.778383330260366435 ) ) ;
#194740=CARTESIAN_POINT ( 'NONE',  ( 9.500331257164628340, -7.473374494045002869, -1.537682436621775084E-15 ) ) ;
#194742=EDGE_LOOP ( 'NONE', ( #115686, #159375 ) ) ;
#194768=ORIENTED_EDGE ( 'NONE', *, *, #132492, .T. ) ;
#194785=CARTESIAN_POINT ( 'NONE',  ( -0.08058605481485492383, -8.243759731405749136, -10.99970480911961346 ) ) ;
#194788=CYLINDRICAL_SURFACE ( 'NONE', #185746, 0.07999999999999993228 ) ;
#194790=CARTESIAN_POINT ( 'NONE',  ( 0.000000000000000000, -8.176568542494919711, 0.000000000000000000 ) ) ;
#194852=SURFACE_STYLE_USAGE ( .BOTH. , #63783 ) ;
#194863=CARTESIAN_POINT ( 'NONE',  ( -0.4382560683119315903, -5.166862915010159263, -10.99126615174919408 ) ) ;
#194874=CARTESIAN_POINT ( 'NONE',  ( -0.4655551865852132210, -8.176568542494939251, -9.512045263456258226 ) ) ;
#194920=CIRCLE ( 'NONE', #25457, 10.99999999999999112 ) ;
#194951=CARTESIAN_POINT ( 'NONE',  ( -0.000000000000000000, 3.038454817776199413, 12.00000000000000178 ) ) ;
#194999=VERTEX_POINT ( 'NONE', #70890 ) ;
#195035=DIRECTION ( 'NONE',  ( 0.000000000000000000, 0.000000000000000000, 1.000000000000000000 ) ) ;
#195056=CARTESIAN_POINT ( 'NONE',  ( 11.00029612940780410, -6.479296433800342925, 0.04006801626471419991 ) ) ;
#195073=SURFACE_STYLE_FILL_AREA ( #83442 ) ;
#195084=FACE_OUTER_BOUND ( 'NONE', #154407, .T. ) ;
#195088=CARTESIAN_POINT ( 'NONE',  ( -6.742488139262638275E-15, -9.746166700180788567, 9.500331257164617682 ) ) ;
#195091=LINE ( 'NONE', #30467, #96571 ) ;
#195116=ORIENTED_EDGE ( 'NONE', *, *, #161695, .F. ) ;
#195130=CONICAL_SURFACE ( 'NONE', #126097, 11.53746066217573940, 0.1181278931043537039 ) ;
#195134=ADVANCED_FACE ( 'NONE', ( #5886 ), #173791, .T. ) ;
#195156=CARTESIAN_POINT ( 'NONE',  ( 7.037870247915942734, -8.233137084989836652, -6.381095703207974701 ) ) ;
#195175=ORIENTED_EDGE ( 'NONE', *, *, #204228, .F. ) ;
#195209=CARTESIAN_POINT ( 'NONE',  ( -1.937985808864938540E-15, -9.954378579146972328, -10.91970693179590768 ) ) ;
#195213=CARTESIAN_POINT ( 'NONE',  ( -7.137427359597535492, -7.616807914308467709, 7.137427359599341159 ) ) ;
#195223=CARTESIAN_POINT ( 'NONE',  ( 7.317172100869718143, -6.705807707649934279, -7.317172100869746565 ) ) ;
#195230=EDGE_LOOP ( 'NONE', ( #197644, #136810, #63462, #70761 ) ) ;
#195236=AXIS2_PLACEMENT_3D ( 'NONE', #56535, #21855, #202750 ) ;
#195239=DIRECTION ( 'NONE',  ( 0.000000000000000000, 0.000000000000000000, 1.000000000000000000 ) ) ;
#195240=FILL_AREA_STYLE ('',( #194161 ) ) ;
#195270=CARTESIAN_POINT ( 'NONE',  ( 1.383850883036507884E-15, 0.2000000000000057288, -11.29999999999998828 ) ) ;
#195271=DIRECTION ( 'NONE',  ( 0.000000000000000000, 1.000000000000000000, 0.000000000000000000 ) ) ;
#195289=FACE_BOUND ( 'NONE', #125936, .T. ) ;
#195290=( GEOMETRIC_REPRESENTATION_CONTEXT ( 3 ) GLOBAL_UNCERTAINTY_ASSIGNED_CONTEXT ( ( #212129 ) ) GLOBAL_UNIT_ASSIGNED_CONTEXT ( ( #52892, #134180, #116889 ) ) REPRESENTATION_CONTEXT ( 'NONE', 'WORKASPACE' ) );
#195297=AXIS2_PLACEMENT_3D ( 'NONE', #138266, #24477, #110092 ) ;
#195315=CARTESIAN_POINT ( 'NONE',  ( -9.499801640457404162, -7.008739397177338404, -0.06269018847474143452 ) ) ;
#195316=VERTEX_POINT ( 'NONE', #105584 ) ;
#195317=CARTESIAN_POINT ( 'NONE',  ( 0.000000000000000000, -9.999999999999994671, 0.000000000000000000 ) ) ;
#195331=CARTESIAN_POINT ( 'NONE',  ( 6.549078289569694178, -6.948428148671534466, -6.549078289569718159 ) ) ;
#195353=CARTESIAN_POINT ( 'NONE',  ( -7.629869294364566734, -5.350481869465718354, -7.876942567271131068 ) ) ;
#195361=CARTESIAN_POINT ( 'NONE',  ( 7.341412881700125403, -6.244189044378190445, -6.724721492623487507 ) ) ;
#195512=AXIS2_PLACEMENT_3D ( 'NONE', #70511, #5506, #104123 ) ;
#195534=ADVANCED_FACE ( 'NONE', ( #11248 ), #194276, .T. ) ;
#195545=DIRECTION ( 'NONE',  ( 0.000000000000000000, 0.000000000000000000, 1.000000000000000000 ) ) ;
#195557=CARTESIAN_POINT ( 'NONE',  ( -7.720982897393583677, -6.134628647623485698, 7.834948825496934610 ) ) ;
#195581=DIRECTION ( 'NONE',  ( 0.000000000000000000, 0.000000000000000000, 1.000000000000000000 ) ) ;
#195623=EDGE_CURVE ( 'NONE', #138616, #147438, #132353, .T. ) ;
#195647=CARTESIAN_POINT ( 'NONE',  ( -7.548736465707863275, -7.034525073441514564, -7.548736465707114540 ) ) ;
#195653=EDGE_CURVE ( 'NONE', #175582, #163622, #96812, .T. ) ;
#195687=DIRECTION ( 'NONE',  ( 0.000000000000000000, 0.000000000000000000, -1.000000000000000000 ) ) ;
#195728=CARTESIAN_POINT ( 'NONE',  ( 0.4382560683119269829, -5.166862915010145052, 10.99126615174920474 ) ) ;
#195730=DIRECTION ( 'NONE',  ( 0.000000000000000000, -1.000000000000000000, 0.000000000000000000 ) ) ;
#195732=AXIS2_PLACEMENT_3D ( 'NONE', #143353, #77235, #196335 ) ;
#195792=( NAMED_UNIT ( * ) SI_UNIT ( $, .STERADIAN. ) SOLID_ANGLE_UNIT ( ) );
#195796=AXIS2_PLACEMENT_3D ( 'NONE', #64452, #196586, #96981 ) ;
#195818=VERTEX_POINT ( 'NONE', #86928 ) ;
#195821=DIRECTION ( 'NONE',  ( 1.224646799147343346E-16, 0.000000000000000000, -1.000000000000000000 ) ) ;
#195823=MECHANICAL_DESIGN_GEOMETRIC_PRESENTATION_REPRESENTATION('',(#9054),#119825);
#195864=( NAMED_UNIT ( * ) PLANE_ANGLE_UNIT ( ) SI_UNIT ( $, .RADIAN. ) );
#195874=CARTESIAN_POINT ( 'NONE',  ( 10.85353573482951717, -6.836568542495036205, -0.4635785636673637189 ) ) ;
#195917=DIRECTION ( 'NONE',  ( 0.000000000000000000, 0.000000000000000000, -1.000000000000000000 ) ) ;
#195925=ORIENTED_EDGE ( 'NONE', *, *, #145289, .F. ) ;
#195932=DIRECTION ( 'NONE',  ( 0.000000000000000000, 0.000000000000000000, -1.000000000000000000 ) ) ;
#195939=ADVANCED_FACE ( 'NONE', ( #162086 ), #15976, .T. ) ;
#195943=EDGE_LOOP ( 'NONE', ( #209105, #63165, #39944, #37059 ) ) ;
#195972=UNCERTAINTY_MEASURE_WITH_UNIT (LENGTH_MEASURE( 1.000000000000000082E-05 ), #189438, 'distance_accuracy_value', 'NONE');
#195993=CARTESIAN_POINT ( 'NONE',  ( 6.717278222822382183, -7.246166700180828535, -6.830415307812249814 ) ) ;
#196043=ORIENTED_EDGE ( 'NONE', *, *, #18861, .F. ) ;
#196046=EDGE_CURVE ( 'NONE', #41517, #135108, #85897, .T. ) ;
#196051=CARTESIAN_POINT ( 'NONE',  ( 6.701130199342107296, -6.864242587301194298, -6.729185404178121388 ) ) ;
#196061=VERTEX_POINT ( 'NONE', #213977 ) ;
#196079=ORIENTED_EDGE ( 'NONE', *, *, #158865, .F. ) ;
#196083=CARTESIAN_POINT ( 'NONE',  ( 10.95855051086948251, -7.723431457505092190, -0.6286713519883923018 ) ) ;
#196095=DIRECTION ( 'NONE',  ( -0.000000000000000000, -1.000000000000000000, -0.000000000000000000 ) ) ;
#196111=CARTESIAN_POINT ( 'NONE',  ( 0.07999999999999327094, -9.900000000000005684, 10.91970695577496286 ) ) ;
#196133=LINE ( 'NONE', #197179, #95081 ) ;
#196158=ORIENTED_EDGE ( 'NONE', *, *, #111366, .F. ) ;
#196159=CARTESIAN_POINT ( 'NONE',  ( -0.2514851628625219271, -9.242341987627245459, 9.497468999145645796 ) ) ;
#196185=CARTESIAN_POINT ( 'NONE',  ( 6.764644832398833962, -7.632775601084119010, 6.764644832401402574 ) ) ;
#196198=ADVANCED_FACE ( 'NONE', ( #79747 ), #124520, .F. ) ;
#196210=CARTESIAN_POINT ( 'NONE',  ( -0.07933194154489606187, 7.849261790823902629, -9.499668754385620417 ) ) ;
#196215=DIRECTION ( 'NONE',  ( 0.000000000000000000, 0.000000000000000000, 1.000000000000000000 ) ) ;
#196250=ORIENTED_EDGE ( 'NONE', *, *, #200174, .T. ) ;
#196270=ORIENTED_EDGE ( 'NONE', *, *, #172200, .T. ) ;
#196277=CARTESIAN_POINT ( 'NONE',  ( 10.85075961359305197, 3.974415841077577838, -3.932216895623887432 ) ) ;
#196278=CARTESIAN_POINT ( 'NONE',  ( 6.773846765317333762, -7.246166700180801001, 6.773846765317311558 ) ) ;
#196295=ORIENTED_EDGE ( 'NONE', *, *, #166752, .F. ) ;
#196298=ADVANCED_FACE ( 'NONE', ( #66651 ), #149009, .T. ) ;
#196303=( LENGTH_UNIT ( ) NAMED_UNIT ( * ) SI_UNIT ( .MILLI., .METRE. ) );
#196306=( NAMED_UNIT ( * ) SI_UNIT ( $, .STERADIAN. ) SOLID_ANGLE_UNIT ( ) );
#196319=CARTESIAN_POINT ( 'NONE',  ( -2.791320394097926997E-15, -5.754340240174641963, 10.93220419382255848 ) ) ;
#196335=DIRECTION ( 'NONE',  ( 0.000000000000000000, 0.000000000000000000, -1.000000000000000000 ) ) ;
#196337=VECTOR ( 'NONE', #197018, 1000.000000000000000 ) ;
#196341=B_SPLINE_CURVE_WITH_KNOTS ( 'NONE', 3,
 ( #180176, #78399, #143447, #80539, #13394, #130438, #79470 ),
 .UNSPECIFIED., .F., .F.,
 ( 4, 3, 4 ),
 ( 0.0001788552925466778897, 0.0009000000022260264132, 0.002103779968145178675 ),
 .UNSPECIFIED. ) ;
#196376=CARTESIAN_POINT ( 'NONE',  ( -0.07538891330676925073, -7.154544010627095219, 9.499700864329915007 ) ) ;
#196395=CARTESIAN_POINT ( 'NONE',  ( 7.173763318588945559, -6.681223591462591926, -7.173763318588971316 ) ) ;
#196406=DIRECTION ( 'NONE',  ( -1.000000000000000000, 0.000000000000000000, 0.000000000000000000 ) ) ;
#196410=ORIENTED_EDGE ( 'NONE', *, *, #207563, .T. ) ;
#196420=EDGE_CURVE ( 'NONE', #7171, #89957, #202093, .T. ) ;
#196425=CARTESIAN_POINT ( 'NONE',  ( 7.100579091573050228, -6.583980363594990948, -6.484567079770450881 ) ) ;
#196441=CARTESIAN_POINT ( 'NONE',  ( 10.39230484541318589, 3.447199233515649386, -6.000000000000107470 ) ) ;
#196570=CARTESIAN_POINT ( 'NONE',  ( -10.96785329849814161, -5.223431457505069098, 0.4373225248172953883 ) ) ;
#196586=DIRECTION ( 'NONE',  ( -0.000000000000000000, -1.000000000000000000, -0.000000000000000000 ) ) ;
#196602=CARTESIAN_POINT ( 'NONE',  ( 9.611339018008546731, -6.606549254265010163, -0.3046331935817545578 ) ) ;
#196620=ORIENTED_EDGE ( 'NONE', *, *, #69925, .T. ) ;
#196623=CARTESIAN_POINT ( 'NONE',  ( -2.736367132584055707E-14, -7.616807913964303900, 10.09384657274620523 ) ) ;
#196631=CARTESIAN_POINT ( 'NONE',  ( -0.3636750363432391664, -6.893137084989841235, -10.99449589488467183 ) ) ;
#196637=CARTESIAN_POINT ( 'NONE',  ( 0.06814526087292921419, -6.511064858252400001, 10.88932262995847822 ) ) ;
#196685=CARTESIAN_POINT ( 'NONE',  ( 6.773846765317307117, -7.246166700180829423, -6.773846765317326657 ) ) ;
#196698=EDGE_LOOP ( 'NONE', ( #207502, #188156, #79807, #44667 ) ) ;
#196702=DIRECTION ( 'NONE',  ( -0.3090169943749582759, 0.000000000000000000, -0.9510565162951500895 ) ) ;
#196738=CIRCLE ( 'NONE', #79223, 10.24999999999998934 ) ;
#196749=SURFACE_STYLE_USAGE ( .BOTH. , #12650 ) ;
#196754=AXIS2_PLACEMENT_3D ( 'NONE', #142977, #55292, #106224 ) ;
#196786=DIRECTION ( 'NONE',  ( 0.8660254037844433705, 0.000000000000000000, 0.4999999999999917843 ) ) ;
#196809=ADVANCED_FACE ( 'NONE', ( #74171 ), #66206, .F. ) ;
#196841=( NAMED_UNIT ( * ) PLANE_ANGLE_UNIT ( ) SI_UNIT ( $, .RADIAN. ) );
#196882=CARTESIAN_POINT ( 'NONE',  ( -6.773376349083141790, -7.246166700180801001, -6.661184041420938229 ) ) ;
#196924=CARTESIAN_POINT ( 'NONE',  ( 9.578353140444622937, -9.943513495888055331, -0.1579188828665808730 ) ) ;
#196952=ORIENTED_EDGE ( 'NONE', *, *, #92980, .F. ) ;
#197018=DIRECTION ( 'NONE',  ( -0.000000000000000000, -0.000000000000000000, 1.000000000000000000 ) ) ;
#197126=CARTESIAN_POINT ( 'NONE',  ( 0.08522810233020440551, -9.999176686163549377, 9.579508557966974536 ) ) ;
#197141=COLOUR_RGB ( '', 0.31764706, 0.68627451, 0.89019608) ;
#197163=CARTESIAN_POINT ( 'NONE',  ( -0.2376451031371414890, -9.050179744156148232, 9.497303347810662544 ) ) ;
#197179=CARTESIAN_POINT ( 'NONE',  ( 1.163414459189984696E-15, 7.849261790823902629, -9.499999999999992895 ) ) ;
#197230=CARTESIAN_POINT ( 'NONE',  ( -9.578206935422265644, -9.900000000000005684, 0.1671882239536719994 ) ) ;
#197265=DIRECTION ( 'NONE',  ( 0.000000000000000000, 1.000000000000000000, 0.000000000000000000 ) ) ;
#197267=CARTESIAN_POINT ( 'NONE',  ( -7.681709917290613809, -6.443545996361864425, -7.726139724254739605 ) ) ;
#197280=VERTEX_POINT ( 'NONE', #206735 ) ;
#197323=CARTESIAN_POINT ( 'NONE',  ( 10.88932262995847822, -6.511064858252405330, -0.06814526087292289980 ) ) ;
#197332=CARTESIAN_POINT ( 'NONE',  ( 0.000000000000000000, 4.006659545634088992, 0.000000000000000000 ) ) ;
#197343=DIRECTION ( 'NONE',  ( 0.000000000000000000, 0.000000000000000000, 1.000000000000000000 ) ) ;
#197348=CARTESIAN_POINT ( 'NONE',  ( 9.834497819152550946, 3.956598013261174884, 6.044631300485357350 ) ) ;
#197392=CARTESIAN_POINT ( 'NONE',  ( 6.773846765307952822, -7.473374494058216300, -6.773846765307982132 ) ) ;
#197415=EDGE_LOOP ( 'NONE', ( #141125, #66101, #105109, #54246, #157184 ) ) ;
#197422=CARTESIAN_POINT ( 'NONE',  ( -0.07802162204111612320, -7.185026885904014726, 9.499679971350929009 ) ) ;
#197426=ORIENTED_EDGE ( 'NONE', *, *, #12907, .T. ) ;
#197437=EDGE_CURVE ( 'NONE', #184826, #196061, #69595, .T. ) ;
#197450=CARTESIAN_POINT ( 'NONE',  ( 10.91970695577495754, -5.907420853759267843, 0.08000000000000194456 ) ) ;
#197468=CARTESIAN_POINT ( 'NONE',  ( 0.07933194154487524519, -7.473374494045017968, -9.499668754385622194 ) ) ;
#197594=AXIS2_PLACEMENT_3D ( 'NONE', #14106, #2106, #84454 ) ;
#197644=ORIENTED_EDGE ( 'NONE', *, *, #151935, .F. ) ;
#197654=PLANE ( 'NONE',  #126261 ) ;
#197663=ORIENTED_EDGE ( 'NONE', *, *, #145289, .T. ) ;
#197664=CARTESIAN_POINT ( 'NONE',  ( 10.99970480893080627, -6.134628647623513231, 0.08058608058608522640 ) ) ;
#197676=ORIENTED_EDGE ( 'NONE', *, *, #54068, .T. ) ;
#197689=CARTESIAN_POINT ( 'NONE',  ( 0.4294077647110361440, -6.532648833121148968, 9.469892045836676431 ) ) ;
#197695=COLOUR_RGB ( '', 0.31764706, 0.68627451, 0.89019608) ;
#197718=CARTESIAN_POINT ( 'NONE',  ( 10.96562622554683664, -5.341077028191770104, -0.1833053738655282261 ) ) ;
#197732=ORIENTED_EDGE ( 'NONE', *, *, #83921, .F. ) ;
#197793=EDGE_CURVE ( 'NONE', #70421, #118245, #10150, .T. ) ;
#197808=CARTESIAN_POINT ( 'NONE',  ( 10.39230484541330313, 3.447199233515649386, 5.999999999999906741 ) ) ;
#197894=FACE_OUTER_BOUND ( 'NONE', #54157, .T. ) ;
#197900=CARTESIAN_POINT ( 'NONE',  ( 7.037870247915942734, -8.233137084989836652, -6.381095703207974701 ) ) ;
#197936=ADVANCED_FACE ( 'NONE', ( #128806 ), #114679, .T. ) ;
#197973=TOROIDAL_SURFACE ( 'NONE', #180824, 10.92000000000000171, 0.08000000000000000167 ) ;
#197979=DIRECTION ( 'NONE',  ( 0.000000000000000000, 0.000000000000000000, -1.000000000000000000 ) ) ;
#198048=( NAMED_UNIT ( * ) SI_UNIT ( $, .STERADIAN. ) SOLID_ANGLE_UNIT ( ) );
#198057=ADVANCED_FACE ( 'NONE', ( #49607 ), #194788, .T. ) ;
#198078=CARTESIAN_POINT ( 'NONE',  ( -9.567965691386884686, -9.756398209953335510, 0.1670094623740840944 ) ) ;
#198122=FACE_OUTER_BOUND ( 'NONE', #19970, .T. ) ;
#198132=AXIS2_PLACEMENT_3D ( 'NONE', #21316, #5060, #137253 ) ;
#198151=VECTOR ( 'NONE', #108301, 1000.000000000000000 ) ;
#198183=CARTESIAN_POINT ( 'NONE',  ( -0.09623479069434756616, -9.919835240146305466, -9.499512666137777117 ) ) ;
#198193=CARTESIAN_POINT ( 'NONE',  ( 6.773376349083131132, -7.473374494058229622, 6.661184041420955992 ) ) ;
#198209=CARTESIAN_POINT ( 'NONE',  ( 9.495347311156807635, -6.857257212219900921, -1.861063089699362494E-15 ) ) ;
#198232=EDGE_LOOP ( 'NONE', ( #124301, #108120, #130130, #147110 ) ) ;
#198271=B_SPLINE_CURVE_WITH_KNOTS ( 'NONE', 3,
 ( #40773, #206441, #55936, #106876, #41848, #207512, #107958, #173986, #10370, #192315 ),
 .UNSPECIFIED., .F., .F.,
 ( 4, 2, 2, 2, 4 ),
 ( 0.000000000000000000, 0.0002021113321160286787, 0.0004042226642320573575, 0.0006063339963480859820, 0.0008084453284641139560 ),
 .UNSPECIFIED. ) ;
#198287=DIRECTION ( 'NONE',  ( -0.007014632059889177630, -1.866992567669147331E-16, -0.9999753971658824625 ) ) ;
#198326=DIRECTION ( 'NONE',  ( 0.000000000000000000, 1.000000000000000000, 0.000000000000000000 ) ) ;
#198377=CARTESIAN_POINT ( 'NONE',  ( 7.721398836998350390, -5.827195405469540290, -7.721398836998385917 ) ) ;
#198411=EDGE_LOOP ( 'NONE', ( #95245, #70744, #66066, #103281, #185595 ) ) ;
#198444=ORIENTED_EDGE ( 'NONE', *, *, #169231, .F. ) ;
#198446=ORIENTED_EDGE ( 'NONE', *, *, #157926, .T. ) ;
#198448=FACE_OUTER_BOUND ( 'NONE', #16420, .T. ) ;
#198458=CARTESIAN_POINT ( 'NONE',  ( -6.717748655460328067, -7.473374494057241080, -6.717748655458897211 ) ) ;
#198509=CARTESIAN_POINT ( 'NONE',  ( -9.499771308870727182, -7.644320505141722677, -0.06917019444584229793 ) ) ;
#198572=ADVANCED_FACE ( 'NONE', ( #47307 ), #31048, .T. ) ;
#198605=AXIS2_PLACEMENT_3D ( 'NONE', #94022, #11665, #24712 ) ;
#198619=CARTESIAN_POINT ( 'NONE',  ( 0.07538891330674882263, -7.154544010627095219, -9.499700864329891914 ) ) ;
#198715=CARTESIAN_POINT ( 'NONE',  ( 9.473215147174835593, -6.532648913095251864, -0.3561222683123499433 ) ) ;
#198743=AXIS2_PLACEMENT_3D ( 'NONE', #4537, #118391, #119459 ) ;
#198757=ORIENTED_EDGE ( 'NONE', *, *, #102136, .F. ) ;
#198792=STYLED_ITEM ( 'NONE', ( #115824 ), #86509 ) ;
#198800=DIRECTION ( 'NONE',  ( 0.000000000000000000, 1.000000000000000000, 0.000000000000000000 ) ) ;
#198845=CARTESIAN_POINT ( 'NONE',  ( -0.04151047742771058618, -7.963884727586691525, -9.500000000000145661 ) ) ;
#198854=EDGE_CURVE ( 'NONE', #190376, #121012, #48467, .T. ) ;
#198872=CARTESIAN_POINT ( 'NONE',  ( 9.500385102287568273, -7.162053774861992572, -0.01083140255524945791 ) ) ;
#198898=AXIS2_PLACEMENT_3D ( 'NONE', #205703, #174311, #57338 ) ;
#198903=STYLED_ITEM ( 'NONE', ( #74626 ), #189681 ) ;
#198946=CARTESIAN_POINT ( 'NONE',  ( 0.4368516432692164941, -5.631911363926717762, 10.55905904256947636 ) ) ;
#199029=CARTESIAN_POINT ( 'NONE',  ( 9.578206935422253210, -9.900000000000005684, -0.1671882239536598425 ) ) ;
#199040=AXIS2_PLACEMENT_3D ( 'NONE', #142114, #43535, #205997 ) ;
#199113=EDGE_CURVE ( 'NONE', #116857, #71330, #185846, .T. ) ;
#199122=CARTESIAN_POINT ( 'NONE',  ( 0.000000000000000000, 1.000000000000000888, 0.000000000000000000 ) ) ;
#199123=DIRECTION ( 'NONE',  ( 0.000000000000000000, 1.000000000000000000, 0.000000000000000000 ) ) ;
#199147=EDGE_CURVE ( 'NONE', #191645, #90168, #53779, .T. ) ;
#199207=CARTESIAN_POINT ( 'NONE',  ( 2.450243370979061641, 1.813773193624685254, -11.74719778151168015 ) ) ;
#199250=CYLINDRICAL_SURFACE ( 'NONE', #175780, 0.08000000000000020983 ) ;
#199252=VERTEX_POINT ( 'NONE', #139312 ) ;
#199274=EDGE_CURVE ( 'NONE', #103298, #6442, #24452, .T. ) ;
#199309=( NAMED_UNIT ( * ) SI_UNIT ( $, .STERADIAN. ) SOLID_ANGLE_UNIT ( ) );
#199321=LINE ( 'NONE', #1120, #158855 ) ;
#199324=( BOUNDED_SURFACE ( )  B_SPLINE_SURFACE ( 3, 2, ( 
 ( #147632, #182233, #196376 ),
 ( #213650, #33857, #197422 ),
 ( #166000, #17585, #48016 ),
 ( #116244, #183306, #49064 ) ),
 .UNSPECIFIED., .F., .F., .T. ) 
 B_SPLINE_SURFACE_WITH_KNOTS ( ( 4, 4 ),
 ( 3, 3 ),
 ( -5.421010862427522170E-20, 9.170893477921754312E-05 ),
 ( 0.000000000000000000, 1.000000000000000000 ),
 .UNSPECIFIED. ) 
 GEOMETRIC_REPRESENTATION_ITEM ( )  RATIONAL_B_SPLINE_SURFACE ( (
 ( 1.000000000000000000, 0.6787756258918329344, 1.000000000000000000),
 ( 1.000000000000000000, 0.6894756946172844181, 1.000000000000000000),
 ( 1.000000000000000000, 0.6998898451712581847, 1.000000000000000000),
 ( 1.000000000000000000, 0.7100530722070645950, 1.000000000000000000) ) ) 
 REPRESENTATION_ITEM ( '' )  SURFACE ( )  );
#199430=MECHANICAL_DESIGN_GEOMETRIC_PRESENTATION_REPRESENTATION('',(#140729),#189092);
#199444=CARTESIAN_POINT ( 'NONE',  ( 9.496893780459336298, -9.200036371099118426, -0.2463816395386141112 ) ) ;
#199509=ORIENTED_EDGE ( 'NONE', *, *, #183561, .T. ) ;
#199525=CARTESIAN_POINT ( 'NONE',  ( 9.499685679921592296, -9.917013740047293524, -0.07729799388535055216 ) ) ;
#199548=B_SPLINE_CURVE_WITH_KNOTS ( 'NONE', 3,
 ( #107610, #23063, #56664, #5732, #122828, #70740, #53451 ),
 .UNSPECIFIED., .F., .F.,
 ( 4, 3, 4 ),
 ( 0.0001126021370636924715, 0.0006031550062628982618, 0.002006790698585274747 ),
 .UNSPECIFIED. ) ;
#199549=CARTESIAN_POINT ( 'NONE',  ( -7.439168848973998216, -6.893137084989842123, -8.103009739377998955 ) ) ;
#199582=ORIENTED_EDGE ( 'NONE', *, *, #188975, .T. ) ;
#199601=ADVANCED_FACE ( 'NONE', ( #14342 ), #59281, .T. ) ;
#199616=DIRECTION ( 'NONE',  ( -0.000000000000000000, -1.000000000000000000, -0.000000000000000000 ) ) ;
#199632=CARTESIAN_POINT ( 'NONE',  ( -6.735605996566196296E-15, -9.900000000000005684, 10.91970695577504458 ) ) ;
#199654=EDGE_LOOP ( 'NONE', ( #209950, #90601, #192298, #44392 ) ) ;
#199707=ORIENTED_EDGE ( 'NONE', *, *, #130618, .T. ) ;
#199717=CIRCLE ( 'NONE', #44212, 11.99999999999999112 ) ;
#199747=PRESENTATION_STYLE_ASSIGNMENT (( #49265 ) ) ;
#199748=B_SPLINE_CURVE_WITH_KNOTS ( 'NONE', 3,
 ( #158813, #42952, #75427, #58108, #190225, #76481, #90628, #24519, #119164, #91705 ),
 .UNSPECIFIED., .F., .F.,
 ( 4, 2, 2, 2, 4 ),
 ( 0.000000000000000000, 0.0002334048330869030008, 0.0004668096661738060016, 0.0007002144992607089481, 0.0009336193323476120031 ),
 .UNSPECIFIED. ) ;
#199763=ORIENTED_EDGE ( 'NONE', *, *, #97288, .T. ) ;
#199778=ADVANCED_FACE ( 'NONE', ( #101480 ), #178839, .T. ) ;
#199791=ORIENTED_EDGE ( 'NONE', *, *, #11694, .F. ) ;
#199804=CARTESIAN_POINT ( 'NONE',  ( -0.4366703603831086355, -8.283751815806034813, 10.40709768291845094 ) ) ;
#199805=CARTESIAN_POINT ( 'NONE',  ( -5.204170427930421283E-15, 3.467171072964057910, -11.99762841690768234 ) ) ;
#199862=CIRCLE ( 'NONE', #61507, 10.97656854249491687 ) ;
#199865=CARTESIAN_POINT ( 'NONE',  ( -0.1749484593404703747, -5.350147675656129032, -10.96499746917716678 ) ) ;
#199873=CARTESIAN_POINT ( 'NONE',  ( -10.91970695577495398, -6.134628647623513231, 8.483881999699072196E-15 ) ) ;
#199985=CYLINDRICAL_SURFACE ( 'NONE', #162056, 0.08000000000000020983 ) ;
#199999=CARTESIAN_POINT ( 'NONE',  ( -0.4655726814510630640, -8.186910006429405584, -9.501690549794776786 ) ) ;
#200016=VERTEX_POINT ( 'NONE', #197900 ) ;
#200064=CARTESIAN_POINT ( 'NONE',  ( -9.483257663143223937, -6.709848117146014701, 0.3912817730721166454 ) ) ;
#200109=CARTESIAN_POINT ( 'NONE',  ( 9.578284150245949036, -9.932867526282002757, -0.1622940087187645097 ) ) ;
#200135=CARTESIAN_POINT ( 'NONE',  ( -9.579665964935227151, -7.246166700194470067, 0.000000000000000000 ) ) ;
#200141=CARTESIAN_POINT ( 'NONE',  ( 0.2903707658989269080, -5.254568858751053284, 10.97058181929407894 ) ) ;
#200165=DIRECTION ( 'NONE',  ( 8.881784197001252323E-16, 0.000000000000000000, -1.000000000000000000 ) ) ;
#200174=EDGE_CURVE ( 'NONE', #200016, #182623, #175594, .T. ) ;
#200197=CARTESIAN_POINT ( 'NONE',  ( -9.500232605408747588, -7.619382996155716015, -0.01181297548859716086 ) ) ;
#200218=VECTOR ( 'NONE', #16220, 1000.000000000000000 ) ;
#200224=DIRECTION ( 'NONE',  ( -1.224646799147355426E-16, 0.000000000000000000, -1.000000000000000000 ) ) ;
#200276=CIRCLE ( 'NONE', #89620, 0.08000000000000020983 ) ;
#200277=CARTESIAN_POINT ( 'NONE',  ( 10.00198841338951716, 1.970899860167793616, 6.221464951635504725 ) ) ;
#200299=EDGE_CURVE ( 'NONE', #116857, #208229, #168605, .T. ) ;
#200307=CARTESIAN_POINT ( 'NONE',  ( -0.08676667164122778275, -9.915770458193639669, -9.499603944220581297 ) ) ;
#200318=CARTESIAN_POINT ( 'NONE',  ( -9.492660725451591119, -6.771447601804276850, 0.03895569783345646103 ) ) ;
#200319=CARTESIAN_POINT ( 'NONE',  ( 9.499679989893813570, -7.184999792974224420, 0.07801928546529238173 ) ) ;
#200355=VERTEX_POINT ( 'NONE', #110376 ) ;
#200363=CARTESIAN_POINT ( 'NONE',  ( 10.39230484541318589, 4.000000000000003553, -6.000000000000107470 ) ) ;
#200371=( GEOMETRIC_REPRESENTATION_CONTEXT ( 3 ) GLOBAL_UNCERTAINTY_ASSIGNED_CONTEXT ( ( #16116 ) ) GLOBAL_UNIT_ASSIGNED_CONTEXT ( ( #64787, #177125, #64440 ) ) REPRESENTATION_CONTEXT ( 'NONE', 'WORKASPACE' ) );
#200403=LINE ( 'NONE', #19529, #4419 ) ;
#200407=AXIS2_PLACEMENT_3D ( 'NONE', #95216, #132002, #161266 ) ;
#200418=DIRECTION ( 'NONE',  ( -0.03984146075563036599, -3.484297484818016589E-16, -0.9992060137953822085 ) ) ;
#200438=EDGE_CURVE ( 'NONE', #113976, #183546, #127267, .T. ) ;
#200466=EDGE_LOOP ( 'NONE', ( #196250, #187047, #128261, #135, #198757 ) ) ;
#200496=ADVANCED_FACE ( 'NONE', ( #212040 ), #210977, .F. ) ;
#200508=CARTESIAN_POINT ( 'NONE',  ( 9.486534023829911177, -9.006863021369365896, -0.5123739589067538569 ) ) ;
#200521=CARTESIAN_POINT ( 'NONE',  ( 0.000000000000000000, -9.999999999999994671, 0.000000000000000000 ) ) ;
#200527=ORIENTED_EDGE ( 'NONE', *, *, #7456, .T. ) ;
#200530=AXIS2_PLACEMENT_3D ( 'NONE', #30930, #28782, #61276 ) ;
#200537=FACE_OUTER_BOUND ( 'NONE', #60219, .T. ) ;
#200545=ORIENTED_EDGE ( 'NONE', *, *, #93956, .T. ) ;
#200578=CARTESIAN_POINT ( 'NONE',  ( 7.874499448206170094, -5.294771359305315173, -7.680942717881076298 ) ) ;
#200583=DIRECTION ( 'NONE',  ( 0.000000000000000000, 1.000000000000000000, 0.000000000000000000 ) ) ;
#200585=CARTESIAN_POINT ( 'NONE',  ( -10.99952653502856137, -9.917017194762472343, 0.1020740558599455700 ) ) ;
#200641=ORIENTED_EDGE ( 'NONE', *, *, #113228, .T. ) ;
#200691=EDGE_CURVE ( 'NONE', #53448, #194558, #120291, .T. ) ;
#200763=PLANE ( 'NONE',  #94689 ) ;
#200786=B_SPLINE_CURVE_WITH_KNOTS ( 'NONE', 3,
 ( #17904, #83990, #99199, #49379, #65587, #28060 ),
 .UNSPECIFIED., .F., .F.,
 ( 4, 2, 4 ),
 ( 0.000000000000000000, 0.0002955107118803974257, 0.0005910214237607931166 ),
 .UNSPECIFIED. ) ;
#200815=ORIENTED_EDGE ( 'NONE', *, *, #186726, .T. ) ;
#200866=ADVANCED_FACE ( 'NONE', ( #118898 ), #116873, .T. ) ;
#200868=CARTESIAN_POINT ( 'NONE',  ( 0.3912817730720326015, -6.709848117146032465, 9.483257663143165317 ) ) ;
#200892=CARTESIAN_POINT ( 'NONE',  ( 10.96785329849812918, -5.223431457505069098, -0.4373225248172805113 ) ) ;
#200906=ORIENTED_EDGE ( 'NONE', *, *, #186853, .F. ) ;
#200910=B_SPLINE_CURVE_WITH_KNOTS ( 'NONE', 3,
 ( #178308, #127503, #76514, #60267, #143708, #142625 ),
 .UNSPECIFIED., .F., .F.,
 ( 4, 2, 4 ),
 ( 0.000000000000000000, 0.001225895755212361464, 0.002451791510424722927 ),
 .UNSPECIFIED. ) ;
#200914=( NAMED_UNIT ( * ) SI_UNIT ( $, .STERADIAN. ) SOLID_ANGLE_UNIT ( ) );
#200970=CARTESIAN_POINT ( 'NONE',  ( 4.806723615010448736E-13, -7.868798029037617603, -9.500000000000001776 ) ) ;
#200993=ADVANCED_FACE ( 'NONE', ( #155612 ), #81432, .T. ) ;
#201007=CARTESIAN_POINT ( 'NONE',  ( 0.000000000000000000, 3.956598013261175772, 0.000000000000000000 ) ) ;
#201018=CARTESIAN_POINT ( 'NONE',  ( 10.98194350564910593, -7.666862915010147717, -0.6300133639306331190 ) ) ;
#201051=CARTESIAN_POINT ( 'NONE',  ( -7.720982910012857303, -6.306565840633416187, 7.834948813061215489 ) ) ;
#201067=EDGE_CURVE ( 'NONE', #139878, #213712, #113340, .T. ) ;
#201123=AXIS2_PLACEMENT_3D ( 'NONE', #141752, #26878, #159026 ) ;
#201124=EDGE_CURVE ( 'NONE', #94484, #89267, #102997, .T. ) ;
#201185=CARTESIAN_POINT ( 'NONE',  ( -10.99861993420630135, -9.955063214563455887, 0.1919715503786826039 ) ) ;
#201192=CARTESIAN_POINT ( 'NONE',  ( 9.578206935422253210, -9.900000000000005684, -0.1671882239536598425 ) ) ;
#201199=EDGE_CURVE ( 'NONE', #183422, #192481, #190826, .T. ) ;
#201239=AXIS2_PLACEMENT_3D ( 'NONE', #25464, #204183, #21171 ) ;
#201277=( LENGTH_UNIT ( ) NAMED_UNIT ( * ) SI_UNIT ( .MILLI., .METRE. ) );
#201294=CARTESIAN_POINT ( 'NONE',  ( 1.432836755002401904E-15, 0.9999999999999978906, -11.69999999999999041 ) ) ;
#201303=CARTESIAN_POINT ( 'NONE',  ( 8.794101853178714734, 3.696394713403113652, 7.873312689837477230 ) ) ;
#201359=CARTESIAN_POINT ( 'NONE',  ( -0.07933194154488883154, -9.900000000000005684, -9.499668754385620417 ) ) ;
#201376=CARTESIAN_POINT ( 'NONE',  ( 0.3793797362571560972, -6.699757570937929785, 10.99387514841215285 ) ) ;
#201394=CARTESIAN_POINT ( 'NONE',  ( 0.000000000000000000, 0.9999999999999978906, 11.69999999999999041 ) ) ;
#201412=DIRECTION ( 'NONE',  ( 0.000000000000000000, 0.000000000000000000, 1.000000000000000000 ) ) ;
#201463=CARTESIAN_POINT ( 'NONE',  ( 9.499065438569621378, -8.103879979615417284, -0.1510907968719069627 ) ) ;
#201466=AXIS2_PLACEMENT_3D ( 'NONE', #88311, #121954, #5952 ) ;
#201472=ORIENTED_EDGE ( 'NONE', *, *, #11734, .F. ) ;
#201478=DIRECTION ( 'NONE',  ( 0.000000000000000000, -1.000000000000000000, 0.000000000000000000 ) ) ;
#201484=CARTESIAN_POINT ( 'NONE',  ( 10.98765602437503830, -5.221050908132835566, 8.077306185017006456E-15 ) ) ;
#201509=CARTESIAN_POINT ( 'NONE',  ( -6.701130152864324785, -6.864242550357222861, 6.729185449012851983 ) ) ;
#201530=VERTEX_POINT ( 'NONE', #213919 ) ;
#201551=VERTEX_POINT ( 'NONE', #148954 ) ;
#201555=CARTESIAN_POINT ( 'NONE',  ( -0.1963700886235999477, -6.681311647492901962, -9.612263720970510406 ) ) ;
#201569=CARTESIAN_POINT ( 'NONE',  ( 9.499562137383495752, -9.414773216041249171, -0.1228851354130882229 ) ) ;
#201589=VERTEX_POINT ( 'NONE', #150029 ) ;
#201633=ORIENTED_EDGE ( 'NONE', *, *, #190367, .T. ) ;
#201640=CARTESIAN_POINT ( 'NONE',  ( -6.634380643896215624, -6.684699857435322023, -6.783773228136961819 ) ) ;
#201646=CARTESIAN_POINT ( 'NONE',  ( -6.396834479292728304, -8.176568542494925040, -7.055228938193916832 ) ) ;
#201659=CYLINDRICAL_SURFACE ( 'NONE', #48138, 10.24999999999998934 ) ;
#201662=EDGE_LOOP ( 'NONE', ( #210164, #58091, #28605, #63282 ) ) ;
#201674=DIRECTION ( 'NONE',  ( 0.000000000000000000, 1.000000000000000000, 0.000000000000000000 ) ) ;
#201684=EDGE_CURVE ( 'NONE', #178508, #94234, #50387, .T. ) ;
#201696=ADVANCED_FACE ( 'NONE', ( #151102 ), #157972, .T. ) ;
#201706=ADVANCED_FACE ( 'NONE', ( #187836 ), #139112, .F. ) ;
#201757=FACE_OUTER_BOUND ( 'NONE', #130769, .T. ) ;
#201765=B_SPLINE_CURVE_WITH_KNOTS ( 'NONE', 3,
 ( #119396, #170207, #4475, #202690, #21791, #54340, #103086, #87900 ),
 .UNSPECIFIED., .F., .F.,
 ( 4, 2, 2, 4 ),
 ( 0.000000000000000000, 0.0002034531274099171216, 0.0004069062548198347853, 0.0008138125096396682696 ),
 .UNSPECIFIED. ) ;
#201793=EDGE_CURVE ( 'NONE', #45587, #322, #35849, .T. ) ;
#201806=VERTEX_POINT ( 'NONE', #56783 ) ;
#201811=CARTESIAN_POINT ( 'NONE',  ( 6.770610912236886492, -7.154544010627095219, 6.663994888585879295 ) ) ;
#201834=CARTESIAN_POINT ( 'NONE',  ( 7.346809171966453889, -6.836568542494980250, 8.002408263930263388 ) ) ;
#201882=EDGE_CURVE ( 'NONE', #17720, #77260, #28191, .T. ) ;
#201919=CARTESIAN_POINT ( 'NONE',  ( -6.392587740394331419, -6.532648833121162291, -6.999862025036984292 ) ) ;
#201973=FACE_OUTER_BOUND ( 'NONE', #21010, .T. ) ;
#202058=CARTESIAN_POINT ( 'NONE',  ( -10.20634067979409565, 1.972237431424338716, 5.892633538919476166 ) ) ;
#202065=CARTESIAN_POINT ( 'NONE',  ( -10.04957930738605931, 3.829867255648770730, -5.932860765075387732 ) ) ;
#202067=EDGE_LOOP ( 'NONE', ( #98312, #72295, #116526, #29045 ) ) ;
#202088=CARTESIAN_POINT ( 'NONE',  ( 0.04536344973641179279, -10.00000000000001954, 9.579592128872851831 ) ) ;
#202093=B_SPLINE_CURVE_WITH_KNOTS ( 'NONE', 3,
 ( #53640, #119773, #102388, #169523, #134917, #168456, #152214 ),
 .UNSPECIFIED., .F., .F.,
 ( 4, 3, 4 ),
 ( 0.0001126021369352508755, 0.001495765174703660855, 0.002006790696433096138 ),
 .UNSPECIFIED. ) ;
#202096=DIRECTION ( 'NONE',  ( 0.000000000000000000, 1.000000000000000000, 0.000000000000000000 ) ) ;
#202103=EDGE_LOOP ( 'NONE', ( #68478, #200906, #22667, #163663 ) ) ;
#202113=CARTESIAN_POINT ( 'NONE',  ( -10.10286202908859465, -8.578580700073972665, 0.6127037010540659079 ) ) ;
#202122=ADVANCED_FACE ( 'NONE', ( #149530 ), #33637, .T. ) ;
#202142=VECTOR ( 'NONE', #7729, 1000.000000000000000 ) ;
#202152=CARTESIAN_POINT ( 'NONE',  ( 10.94445979172680694, -5.609732095436334554, -0.02903434592765111177 ) ) ;
#202157=B_SPLINE_CURVE_WITH_KNOTS ( 'NONE', 3,
 ( #163602, #28260, #94353, #11996 ),
 .UNSPECIFIED., .F., .F.,
 ( 4, 4 ),
 ( 0.000000000000000000, 6.033646489357627837E-05 ),
 .UNSPECIFIED. ) ;
#202181=CARTESIAN_POINT ( 'NONE',  ( 0.000000000000000000, 4.000000000000003553, 12.00000000000000178 ) ) ;
#202202=AXIS2_PLACEMENT_3D ( 'NONE', #73230, #74327, #159838 ) ;
#202228=CARTESIAN_POINT ( 'NONE',  ( -0.07538891330675576152, -7.154544010627095219, 9.499700864329900796 ) ) ;
#202251=B_SPLINE_CURVE_WITH_KNOTS ( 'NONE', 3,
 ( #158192, #42315, #9783, #154983 ),
 .UNSPECIFIED., .F., .F.,
 ( 4, 4 ),
 ( 0.0006294919072214896988, 0.001039439579420691623 ),
 .UNSPECIFIED. ) ;
#202339=COLOUR_RGB ( '', 0.08235294, 0.09019608, 0.10196078) ;
#202344=ADVANCED_FACE ( 'NONE', ( #170030 ), #137561, .T. ) ;
#202360=CARTESIAN_POINT ( 'NONE',  ( -0.4355862708380086046, -6.583980363594969631, -9.606148981167432765 ) ) ;
#202363=CIRCLE ( 'NONE', #109078, 0.08000000000000020983 ) ;
#202371=FACE_OUTER_BOUND ( 'NONE', #161563, .T. ) ;
#202413=EDGE_CURVE ( 'NONE', #157260, #90864, #141292, .T. ) ;
#202431=DIRECTION ( 'NONE',  ( 0.000000000000000000, 0.000000000000000000, 1.000000000000000000 ) ) ;
#202440=CARTESIAN_POINT ( 'NONE',  ( -0.08058605610039842881, -6.304485801116100241, 10.99970480911019699 ) ) ;
#202443=ORIENTED_EDGE ( 'NONE', *, *, #97172, .F. ) ;
#202457=EDGE_CURVE ( 'NONE', #144861, #129260, #58862, .T. ) ;
#202469=ORIENTED_EDGE ( 'NONE', *, *, #84925, .F. ) ;
#202476=CYLINDRICAL_SURFACE ( 'NONE', #64019, 0.09999999999999986677 ) ;
#202531=DIRECTION ( 'NONE',  ( 0.000000000000000000, 1.000000000000000000, 0.000000000000000000 ) ) ;
#202540=FACE_OUTER_BOUND ( 'NONE', #150001, .T. ) ;
#202541=FACE_OUTER_BOUND ( 'NONE', #149649, .T. ) ;
#202551=CARTESIAN_POINT ( 'NONE',  ( 10.97895254167818813, -5.212340523078044185, -0.4373349612950642729 ) ) ;
#202593=ORIENTED_EDGE ( 'NONE', *, *, #203566, .F. ) ;
#202598=ORIENTED_EDGE ( 'NONE', *, *, #154559, .F. ) ;
#202624=CARTESIAN_POINT ( 'NONE',  ( -7.730132016633767478, -5.756136661604486449, 7.730132016633794123 ) ) ;
#202635=CARTESIAN_POINT ( 'NONE',  ( 10.45358220256315285, 1.000000000000000888, -5.892590188894412329 ) ) ;
#202638=DIRECTION ( 'NONE',  ( 0.000000000000000000, -1.000000000000000000, 0.000000000000000000 ) ) ;
#202645=CARTESIAN_POINT ( 'NONE',  ( -10.86205067566995730, -6.804704122739859251, 0.3107038660269559327 ) ) ;
#202659=ORIENTED_EDGE ( 'NONE', *, *, #148379, .F. ) ;
#202690=CARTESIAN_POINT ( 'NONE',  ( 10.14641618983893068, 3.870538056096204826, -5.683069686889757222 ) ) ;
#202708=ORIENTED_EDGE ( 'NONE', *, *, #104440, .T. ) ;
#202712=CARTESIAN_POINT ( 'NONE',  ( 0.4373225248172820656, -7.723431457505077979, -10.96785329849813273 ) ) ;
#202713=DIRECTION ( 'NONE',  ( 0.7347175152297780176, 0.000000000000000000, -0.6783731810844091381 ) ) ;
#202721=CARTESIAN_POINT ( 'NONE',  ( 9.499717950937025535, -9.918872507113817960, -0.07320418461264667498 ) ) ;
#202732=EDGE_CURVE ( 'NONE', #193316, #129112, #213815, .T. ) ;
#202740=DIRECTION ( 'NONE',  ( 0.000000000000000000, 0.000000000000000000, -1.000000000000000000 ) ) ;
#202750=DIRECTION ( 'NONE',  ( -0.03984146075563027578, 0.000000000000000000, -0.9992060137953822085 ) ) ;
#202870=DIRECTION ( 'NONE',  ( -0.000000000000000000, 1.000000000000000000, -0.000000000000000000 ) ) ;
#202937=CARTESIAN_POINT ( 'NONE',  ( -10.99970480893081337, -5.907420853759282053, -0.08058608058607207025 ) ) ;
#202956=CARTESIAN_POINT ( 'NONE',  ( -2.276824562219559311E-15, -8.030730635398800388, -11.29670623088187398 ) ) ;
#202997=CARTESIAN_POINT ( 'NONE',  ( 10.99526901688165026, -7.794005300192742069, -0.3296348669024388722 ) ) ;
#203006=CARTESIAN_POINT ( 'NONE',  ( 0.2039282260587823581, -6.674536912880641104, 9.612297698795920553 ) ) ;
#203056=VECTOR ( 'NONE', #182694, 1000.000000000000000 ) ;
#203108=ADVANCED_FACE ( 'NONE', ( #133304 ), #37333, .T. ) ;
#203172=CARTESIAN_POINT ( 'NONE',  ( 6.511381374296898450, -8.144978210217303172, 6.953912913643685023 ) ) ;
#203182=EDGE_CURVE ( 'NONE', #62943, #95548, #185446, .T. ) ;
#203194=DIRECTION ( 'NONE',  ( -0.000000000000000000, 1.000000000000000000, -0.000000000000000000 ) ) ;
#203216=EDGE_LOOP ( 'NONE', ( #26246, #65775, #52027, #110073, #46640, #183241, #86888, #80491, #37719, #196079, #206975, #4991, #50430, #73189, #69785, #180581, #4299, #54122, #185676, #118687, #105133 ) ) ;
#203263=CARTESIAN_POINT ( 'NONE',  ( 11.40591166468351503, 3.507114751586604129, -3.706005353348470255 ) ) ;
#203266=DIRECTION ( 'NONE',  ( 1.000000000000000000, 0.000000000000000000, 0.000000000000000000 ) ) ;
#203310=ORIENTED_EDGE ( 'NONE', *, *, #205165, .F. ) ;
#203367=CARTESIAN_POINT ( 'NONE',  ( -9.499606442108966320, -9.900000000000019895, 0.08647222121522583904 ) ) ;
#203391=DIRECTION ( 'NONE',  ( -0.000000000000000000, 1.000000000000000000, -0.000000000000000000 ) ) ;
#203402=EDGE_CURVE ( 'NONE', #183550, #102475, #92726, .T. ) ;
#203407=DIRECTION ( 'NONE',  ( 0.000000000000000000, -1.000000000000000000, 0.000000000000000000 ) ) ;
#203413=VECTOR ( 'NONE', #61298, 1000.000000000000000 ) ;
#203426=CARTESIAN_POINT ( 'NONE',  ( -0.4294077647110585150, -6.532648833121148968, -9.469892045836655114 ) ) ;
#203429=ADVANCED_FACE ( 'NONE', ( #186266 ), #152267, .F. ) ;
#203439=CARTESIAN_POINT ( 'NONE',  ( -0.1370650511771418500, -7.902328468025382691, 10.96100467917833399 ) ) ;
#203507=CARTESIAN_POINT ( 'NONE',  ( -6.845108005540232021, -7.986884274785872151, 6.643335646896343150 ) ) ;
#203514=AXIS2_PLACEMENT_3D ( 'NONE', #87334, #1785, #138232 ) ;
#203540=DIRECTION ( 'NONE',  ( 0.000000000000000000, 1.084202172485501594E-14, -1.000000000000000000 ) ) ;
#203545=EDGE_LOOP ( 'NONE', ( #111763, #189670, #149300, #202469 ) ) ;
#203566=EDGE_CURVE ( 'NONE', #78601, #45420, #186215, .T. ) ;
#203569=PRESENTATION_STYLE_ASSIGNMENT (( #168959 ) ) ;
#203618=DIRECTION ( 'NONE',  ( -0.000000000000000000, 1.000000000000000000, -0.000000000000000000 ) ) ;
#203635=ADVANCED_FACE ( 'NONE', ( #95202 ), #123515, .T. ) ;
#203647=ORIENTED_EDGE ( 'NONE', *, *, #205165, .T. ) ;
#203656=EDGE_LOOP ( 'NONE', ( #163351, #56827, #2534 ) ) ;
#203670=DIRECTION ( 'NONE',  ( 0.000000000000000000, 0.000000000000000000, 1.000000000000000000 ) ) ;
#203687=CARTESIAN_POINT ( 'NONE',  ( 10.38614328979755719, 3.507114751586604129, -5.996442624206805405 ) ) ;
#203729=CARTESIAN_POINT ( 'NONE',  ( 9.811039896441892338, -7.242250812739402299, 1.725646424474048093E-15 ) ) ;
#203732=CARTESIAN_POINT ( 'NONE',  ( -7.710100441483604072, -6.699703214240861904, -7.845789747616953136 ) ) ;
#203777=CARTESIAN_POINT ( 'NONE',  ( 0.04151047742771083598, -7.963884727586698631, 9.500000000000147438 ) ) ;
#203804=DIRECTION ( 'NONE',  ( 0.000000000000000000, 1.000000000000000000, 0.000000000000000000 ) ) ;
#203811=PLANE ( 'NONE',  #144680 ) ;
#203821=ADVANCED_FACE ( 'NONE', ( #38720 ), #159217, .T. ) ;
#203829=ORIENTED_EDGE ( 'NONE', *, *, #92379, .T. ) ;
#203838=CARTESIAN_POINT ( 'NONE',  ( 7.550983558724411182, -6.148216694138056937, -7.550983558724436051 ) ) ;
#203894=CARTESIAN_POINT ( 'NONE',  ( 0.1007326007325774070, -9.920000000000095852, 10.99953876047307944 ) ) ;
#203907=CARTESIAN_POINT ( 'NONE',  ( -0.1520312049661516063, -8.104757123234351823, -9.499050059654539524 ) ) ;
#204007=CARTESIAN_POINT ( 'NONE',  ( 6.717278222822382183, 7.849261790823902629, -6.830415307812251591 ) ) ;
#204013=VERTEX_POINT ( 'NONE', #138364 ) ;
#204018=DIRECTION ( 'NONE',  ( -0.000000000000000000, -1.000000000000000000, -0.000000000000000000 ) ) ;
#204045=ORIENTED_EDGE ( 'NONE', *, *, #79889, .T. ) ;
#204050=CYLINDRICAL_SURFACE ( 'NONE', #176933, 0.08000000000000020983 ) ;
#204059=CARTESIAN_POINT ( 'NONE',  ( 8.043940816608021294, -6.893137084989709784, -7.503508839934921681 ) ) ;
#204069=CARTESIAN_POINT ( 'NONE',  ( 0.08246874231330963978, -9.908734156519555469, 10.99969088041220999 ) ) ;
#204094=COLOUR_RGB ( '', 0.66274510, 0.83137255, 0.94901961) ;
#204183=DIRECTION ( 'NONE',  ( -0.000000000000000000, -1.000000000000000000, -0.000000000000000000 ) ) ;
#204192=CARTESIAN_POINT ( 'NONE',  ( -10.53927507717405909, 2.018041202054385419, 6.084853302870027569 ) ) ;
#204210=CARTESIAN_POINT ( 'NONE',  ( -9.499643733017421710, -9.912496545390952818, 0.08228199421455106854 ) ) ;
#204211=CARTESIAN_POINT ( 'NONE',  ( 10.96381302404140179, -7.750949308402022453, -0.4891431138946180646 ) ) ;
#204228=EDGE_CURVE ( 'NONE', #183752, #115982, #110324, .T. ) ;
#204240=ORIENTED_EDGE ( 'NONE', *, *, #42999, .F. ) ;
#204272=EDGE_LOOP ( 'NONE', ( #5840, #152607, #165328, #88110 ) ) ;
#204280=SURFACE_SIDE_STYLE ('',( #171819 ) ) ;
#204316=CARTESIAN_POINT ( 'NONE',  ( -9.469892045836674654, -6.532648833121162291, 0.4294077647110516871 ) ) ;
#204317=CARTESIAN_POINT ( 'NONE',  ( 9.578928831967440161, -9.999999999999978684, -0.1215685829351341452 ) ) ;
#204321=CARTESIAN_POINT ( 'NONE',  ( 0.000000000000000000, -2.000000000000001776, 10.24999999999998934 ) ) ;
#204359=CARTESIAN_POINT ( 'NONE',  ( -6.824425546749161242, -8.104785249476792686, 6.609253696060804373 ) ) ;
#204428=UNCERTAINTY_MEASURE_WITH_UNIT (LENGTH_MEASURE( 1.000000000000000082E-05 ), #33353, 'distance_accuracy_value', 'NONE');
#204430=CARTESIAN_POINT ( 'NONE',  ( -10.99943592164172834, -8.407420853759269619, 0.1113975120798846308 ) ) ;
#204434=LINE ( 'NONE', #188203, #190007 ) ;
#204435=CARTESIAN_POINT ( 'NONE',  ( -7.058808231563621582, -6.527411821100059797, 6.446420058208181203 ) ) ;
#204449=( NAMED_UNIT ( * ) PLANE_ANGLE_UNIT ( ) SI_UNIT ( $, .RADIAN. ) );
#204462=ORIENTED_EDGE ( 'NONE', *, *, #40921, .T. ) ;
#204470=FACE_OUTER_BOUND ( 'NONE', #10610, .T. ) ;
#204480=CARTESIAN_POINT ( 'NONE',  ( -6.673079560224743467, -7.008190897455698121, 6.761669295867172025 ) ) ;
#204505=CARTESIAN_POINT ( 'NONE',  ( 8.762124912781171560, 3.934209603697781166, 7.549522310265921021 ) ) ;
#204559=CARTESIAN_POINT ( 'NONE',  ( -0.08832626591289140239, -9.919998018383708427, -9.499595568239943333 ) ) ;
#204576=CARTESIAN_POINT ( 'NONE',  ( -9.474246188248169886, -6.532648833121168508, 0.3333842132581058548 ) ) ;
#204579=ORIENTED_EDGE ( 'NONE', *, *, #143132, .T. ) ;
#204589=CARTESIAN_POINT ( 'NONE',  ( -9.490416961614045022, -9.037429132956699362, 0.4317745627846718559 ) ) ;
#204595=LINE ( 'NONE', #56248, #129762 ) ;
#204616=ORIENTED_EDGE ( 'NONE', *, *, #106413, .T. ) ;
#204617=FACE_OUTER_BOUND ( 'NONE', #172262, .T. ) ;
#204625=CARTESIAN_POINT ( 'NONE',  ( 0.08058608058606961388, -5.907420853759267843, -10.99970480893079738 ) ) ;
#204648=DIRECTION ( 'NONE',  ( -0.000000000000000000, 1.000000000000000000, -0.000000000000000000 ) ) ;
#204663=CIRCLE ( 'NONE', #52541, 6.329999999999995630 ) ;
#204666=CARTESIAN_POINT ( 'NONE',  ( -10.36809559534898284, -7.321523296574929063, 0.4642244361878736236 ) ) ;
#204686=CARTESIAN_POINT ( 'NONE',  ( 9.569423160901791903, -7.256398209936433474, 9.269928574751062911E-15 ) ) ;
#204789=CARTESIAN_POINT ( 'NONE',  ( -10.90207482560803420, -7.666862915010147717, 0.6254314485565921622 ) ) ;
#204797=AXIS2_PLACEMENT_3D ( 'NONE', #99016, #137658, #86757 ) ;
#204799=VERTEX_POINT ( 'NONE', #186954 ) ;
#204826=AXIS2_PLACEMENT_3D ( 'NONE', #80297, #164741, #99742 ) ;
#204829=CARTESIAN_POINT ( 'NONE',  ( 6.880414557363751626, -8.057948861126641660, -6.598949805828051574 ) ) ;
#204837=ORIENTED_EDGE ( 'NONE', *, *, #182421, .T. ) ;
#204853=CARTESIAN_POINT ( 'NONE',  ( 6.661184041420940005, -7.246166700180828535, -6.773376349083132908 ) ) ;
#204865=DIRECTION ( 'NONE',  ( 0.9999455182791218144, -5.694964898128450927E-17, -0.01043841336116897549 ) ) ;
#204878=EDGE_CURVE ( 'NONE', #34907, #156, #110243, .T. ) ;
#204881=AXIS2_PLACEMENT_3D ( 'NONE', #136779, #117381, #86951 ) ;
#204886=CIRCLE ( 'NONE', #111598, 0.07999999999999993228 ) ;
#204909=ORIENTED_EDGE ( 'NONE', *, *, #50401, .F. ) ;
#204949=B_SPLINE_CURVE_WITH_KNOTS ( 'NONE', 3,
 ( #131173, #81293, #176664, #197163, #147370, #213396 ),
 .UNSPECIFIED., .F., .F.,
 ( 4, 2, 4 ),
 ( 0.0004044236633722958431, 0.0006920484658239115742, 0.0009796732682755271426 ),
 .UNSPECIFIED. ) ;
#204951=AXIS2_PLACEMENT_3D ( 'NONE', #182654, #195730, #149095 ) ;
#204968=SURFACE_STYLE_FILL_AREA ( #105386 ) ;
#205038=FACE_OUTER_BOUND ( 'NONE', #207240, .T. ) ;
#205047=CARTESIAN_POINT ( 'NONE',  ( -6.719405205104948209, -7.217450603038109591, 6.716119544743302860 ) ) ;
#205061=CARTESIAN_POINT ( 'NONE',  ( -0.04699017840227408260, -9.984793624843945281, -10.91963405940077791 ) ) ;
#205086=AXIS2_PLACEMENT_3D ( 'NONE', #197450, #62137, #115211 ) ;
#205088=CARTESIAN_POINT ( 'NONE',  ( -6.775479680898469859, -7.217880409000358100, -6.775479680898433443 ) ) ;
#205121=ORIENTED_EDGE ( 'NONE', *, *, #27140, .F. ) ;
#205127=AXIS2_PLACEMENT_3D ( 'NONE', #42526, #104306, #136808 ) ;
#205129=CARTESIAN_POINT ( 'NONE',  ( 7.524604700374169397, -5.166862990899455887, 8.024185963717899384 ) ) ;
#205140=CARTESIAN_POINT ( 'NONE',  ( 0.2834499523633389750, -6.554910290221304336, 9.477100695693453147 ) ) ;
#205165=EDGE_CURVE ( 'NONE', #117856, #45686, #137166, .T. ) ;
#205168=CARTESIAN_POINT ( 'NONE',  ( 0.000000000000000000, 3.079999999999999183, 0.000000000000000000 ) ) ;
#205182=AXIS2_PLACEMENT_3D ( 'NONE', #44489, #174496, #139860 ) ;
#205192=CARTESIAN_POINT ( 'NONE',  ( -1.387778780781445676E-14, -5.907420853759282053, -10.91970695577495398 ) ) ;
#205281=ORIENTED_EDGE ( 'NONE', *, *, #59332, .T. ) ;
#205282=B_SPLINE_CURVE_WITH_KNOTS ( 'NONE', 3,
 ( #145763, #16753, #30920, #45042, #47177, #63402, #194464 ),
 .UNSPECIFIED., .F., .F.,
 ( 4, 3, 4 ),
 ( 4.336808689942000884E-19, 0.0008000000000004425012, 0.002977368225425618478 ),
 .UNSPECIFIED. ) ;
#205295=CARTESIAN_POINT ( 'NONE',  ( -9.499717950937029087, -9.918872507113817960, 0.07320418461264667498 ) ) ;
#205341=B_SPLINE_CURVE_WITH_KNOTS ( 'NONE', 3,
 ( #82304, #29312, #147333, #213362, #161458, #160377, #64983 ),
 .UNSPECIFIED., .F., .F.,
 ( 4, 3, 4 ),
 ( 0.0001126021370636923631, 0.0006031550062628982618, 0.002006790698585272145 ),
 .UNSPECIFIED. ) ;
#205349=( NAMED_UNIT ( * ) SI_UNIT ( $, .STERADIAN. ) SOLID_ANGLE_UNIT ( ) );
#205361=CARTESIAN_POINT ( 'NONE',  ( -10.39649820107528733, 2.629643693813587646, 5.992760101887464330 ) ) ;
#205364=CARTESIAN_POINT ( 'NONE',  ( 0.000000000000000000, 3.079999999999999183, 0.000000000000000000 ) ) ;
#205368=PRESENTATION_STYLE_ASSIGNMENT (( #157721 ) ) ;
#205391=VERTEX_POINT ( 'NONE', #157682 ) ;
#205402=ORIENTED_EDGE ( 'NONE', *, *, #32385, .T. ) ;
#205404=CARTESIAN_POINT ( 'NONE',  ( 11.40816717570227468, 3.487142912321097299, -3.706738213303538920 ) ) ;
#205408=AXIS2_PLACEMENT_3D ( 'NONE', #62972, #45687, #145346 ) ;
#205459=ORIENTED_EDGE ( 'NONE', *, *, #5382, .F. ) ;
#205507=( BOUNDED_SURFACE ( )  B_SPLINE_SURFACE ( 3, 2, ( 
 ( #4370, #101909, #120367 ),
 ( #5435, #71514, #19580 ),
 ( #22759, #88876, #85652 ),
 ( #70440, #151739, #186342 ),
 ( #157882, #137626, #171169 ),
 ( #55294, #95017, #11598 ),
 ( #12658, #128653, #13729 ),
 ( #27859, #144856, #113450 ) ),
 .UNSPECIFIED., .F., .F., .T. ) 
 B_SPLINE_SURFACE_WITH_KNOTS ( ( 4, 2, 2, 4 ),
 ( 3, 3 ),
 ( 0.000000000000000000, 0.0004924884914732721459, 0.0007387327372099082188, 0.0009849769829465442918 ),
 ( 0.000000000000000000, 1.000000000000000000 ),
 .UNSPECIFIED. ) 
 GEOMETRIC_REPRESENTATION_ITEM ( )  RATIONAL_B_SPLINE_SURFACE ( (
 ( 1.000000000000000000, 0.7045118851637635071, 1.000000000000000000),
 ( 1.000000000000000000, 0.7593505504062313394, 1.000000000000000000),
 ( 1.000000000000000000, 0.8104906253035955022, 1.000000000000000000),
 ( 1.000000000000000000, 0.8722646935499712706, 1.000000000000000000),
 ( 1.000000000000000000, 0.8905178607894789211, 1.000000000000000000),
 ( 1.000000000000000000, 0.9170530604353609450, 1.000000000000000000),
 ( 1.000000000000000000, 0.9248184710077420601, 1.000000000000000000),
 ( 1.000000000000000000, 0.9238795325112880708, 1.000000000000000000) ) ) 
 REPRESENTATION_ITEM ( '' )  SURFACE ( )  );
#205542=CARTESIAN_POINT ( 'NONE',  ( -10.99943592164172657, -8.240513804456425007, 0.1113975120798868373 ) ) ;
#205578=CARTESIAN_POINT ( 'NONE',  ( -0.3106162252735292229, -6.604184692106364274, -9.611175950047666561 ) ) ;
#205612=ORIENTED_EDGE ( 'NONE', *, *, #84925, .T. ) ;
#205626=VECTOR ( 'NONE', #27702, 1000.000000000000000 ) ;
#205646=CARTESIAN_POINT ( 'NONE',  ( 8.043985462411169962, -6.893136966056886195, -7.503460210123559015 ) ) ;
#205658=ORIENTED_EDGE ( 'NONE', *, *, #30312, .T. ) ;
#205661=PLANE ( 'NONE',  #38553 ) ;
#205662=CARTESIAN_POINT ( 'NONE',  ( 10.96027417533446524, -7.850147675656145907, -0.3662874062585380619 ) ) ;
#205679=CARTESIAN_POINT ( 'NONE',  ( -6.689804758640344851, -7.818797203689483943, 6.745710774230989415 ) ) ;
#205688=CARTESIAN_POINT ( 'NONE',  ( 0.09999999999999592548, -9.999999999999994671, 6.938893903907228378E-15 ) ) ;
#205689=CARTESIAN_POINT ( 'NONE',  ( 10.32992389895506413, 1.000000000000000888, 6.106772653521394645 ) ) ;
#205703=CARTESIAN_POINT ( 'NONE',  ( 0.000000000000000000, 1.000000000000000888, 0.000000000000000000 ) ) ;
#205716=CARTESIAN_POINT ( 'NONE',  ( -11.46094690312891551, 3.019799309332925841, 3.723887386306169667 ) ) ;
#205726=DIRECTION ( 'NONE',  ( 1.000000000000000000, 0.000000000000000000, 0.000000000000000000 ) ) ;
#205728=EDGE_CURVE ( 'NONE', #67222, #16465, #107631, .T. ) ;
#205737=ORIENTED_EDGE ( 'NONE', *, *, #45640, .T. ) ;
#205749=B_SPLINE_CURVE_WITH_KNOTS ( 'NONE', 3,
 ( #209915, #14908, #109315, #161193, #142843, #113576, #76727, #43202 ),
 .UNSPECIFIED., .F., .F.,
 ( 4, 2, 2, 4 ),
 ( 0.000000000000000000, 0.0004970278158210351136, 0.0007455417237315527246, 0.0009940556316420702272 ),
 .UNSPECIFIED. ) ;
#205754=DIRECTION ( 'NONE',  ( 0.000000000000000000, 0.000000000000000000, -1.000000000000000000 ) ) ;
#205768=DIRECTION ( 'NONE',  ( -1.000000000000000000, 0.000000000000000000, 0.000000000000000000 ) ) ;
#205822=EDGE_CURVE ( 'NONE', #175582, #54346, #6640, .T. ) ;
#205838=CARTESIAN_POINT ( 'NONE',  ( -0.003376046620573100454, -7.161464053357560644, -9.586610838029425707 ) ) ;
#205881=CARTESIAN_POINT ( 'NONE',  ( 0.2376451031371469291, -9.050179744156142903, -9.497303347810662544 ) ) ;
#205883=CARTESIAN_POINT ( 'NONE',  ( -10.55905904256947636, -5.631911363926716874, 0.4368516432692268747 ) ) ;
#205884=EDGE_LOOP ( 'NONE', ( #162824, #57447, #153461, #145228, #66608 ) ) ;
#205894=DIRECTION ( 'NONE',  ( 0.000000000000000000, 1.000000000000000000, 0.000000000000000000 ) ) ;
#205917=VERTEX_POINT ( 'NONE', #213956 ) ;
#205922=ORIENTED_EDGE ( 'NONE', *, *, #124338, .T. ) ;
#205938=CARTESIAN_POINT ( 'NONE',  ( -10.99944587961302034, -9.906575223978485667, 0.1104109902703137719 ) ) ;
#205997=DIRECTION ( 'NONE',  ( 0.000000000000000000, 0.000000000000000000, 1.000000000000000000 ) ) ;
#206056=CARTESIAN_POINT ( 'NONE',  ( -0.3909723190920246227, -8.176244038172828965, -9.516020521606723293 ) ) ;
#206106=B_SPLINE_CURVE_WITH_KNOTS ( 'NONE', 3,
 ( #205838, #57471, #123631, #189594, #201555, #44433, #178691, #125749 ),
 .UNSPECIFIED., .F., .F.,
 ( 4, 2, 2, 4 ),
 ( 0.000000000000000000, 0.0003954713701971531467, 0.0005932070552957296929, 0.0007909427403943062934 ),
 .UNSPECIFIED. ) ;
#206109=CARTESIAN_POINT ( 'NONE',  ( 10.85353573482951717, -6.836568542495036205, -0.4635785636673637189 ) ) ;
#206119=( BOUNDED_SURFACE ( )  B_SPLINE_SURFACE ( 3, 2, ( 
 ( #75925, #43447, #59670 ),
 ( #14092, #44512, #46637 ),
 ( #160376, #76978, #45577 ),
 ( #80182, #29311, #211236 ),
 ( #61808, #28241, #209097 ),
 ( #62862, #127978, #146287 ),
 ( #193930, #11978, #110629 ),
 ( #111693, #130087, #176630 ) ),
 .UNSPECIFIED., .F., .F., .T. ) 
 B_SPLINE_SURFACE_WITH_KNOTS ( ( 4, 2, 2, 4 ),
 ( 3, 3 ),
 ( 0.000000000000000000, 0.0002568729646053923097, 0.0005137459292107846194, 0.001027491858421569239 ),
 ( 0.000000000000000000, 1.000000000000000000 ),
 .UNSPECIFIED. ) 
 GEOMETRIC_REPRESENTATION_ITEM ( )  RATIONAL_B_SPLINE_SURFACE ( (
 ( 1.000000000000000000, 0.3826834323651031600, 1.000000000000000000),
 ( 1.000000000000000000, 0.3847114443838287601, 1.000000000000000000),
 ( 1.000000000000000000, 0.4039255759070156659, 1.000000000000000000),
 ( 1.000000000000000000, 0.4557194474500481651, 1.000000000000000000),
 ( 1.000000000000000000, 0.4874388927525016291, 1.000000000000000000),
 ( 1.000000000000000000, 0.5833547384513821932, 1.000000000000000000),
 ( 1.000000000000000000, 0.6470545345839008311, 1.000000000000000000),
 ( 1.000000000000000000, 0.7045118851637607316, 1.000000000000000000) ) ) 
 REPRESENTATION_ITEM ( '' )  SURFACE ( )  );
#206144=ADVANCED_FACE ( 'NONE', ( #117622 ), #17892, .T. ) ;
#206152=B_SPLINE_CURVE_WITH_KNOTS ( 'NONE', 3,
 ( #206516, #46183, #190265, #157797 ),
 .UNSPECIFIED., .F., .F.,
 ( 4, 4 ),
 ( 0.000000000000000000, 6.033646489354576486E-05 ),
 .UNSPECIFIED. ) ;
#206177=AXIS2_PLACEMENT_3D ( 'NONE', #100046, #149874, #69648 ) ;
#206202=CARTESIAN_POINT ( 'NONE',  ( 6.981856502304780498, -6.709867743870614021, -6.429544252030573226 ) ) ;
#206207=CARTESIAN_POINT ( 'NONE',  ( 7.694877102302470462, -5.389939693150867406, 7.860745937262088923 ) ) ;
#206220=CARTESIAN_POINT ( 'NONE',  ( 0.003376046620569739427, -7.161464053357565973, 9.586610838029432813 ) ) ;
#206222=CARTESIAN_POINT ( 'NONE',  ( -7.664830294503444996, -9.999999999999994671, 7.777967379493320621 ) ) ;
#206345=DIRECTION ( 'NONE',  ( -1.000000000000000000, 0.000000000000000000, 0.000000000000000000 ) ) ;
#206347=CARTESIAN_POINT ( 'NONE',  ( -6.827626583076781053, -7.154544010627095219, -6.720112740279224006 ) ) ;
#206352=VERTEX_POINT ( 'NONE', #150066 ) ;
#206391=DIRECTION ( 'NONE',  ( 0.6783731810844091381, 0.000000000000000000, 0.7347175152297780176 ) ) ;
#206395=EDGE_CURVE ( 'NONE', #74942, #191954, #200276, .T. ) ;
#206441=CARTESIAN_POINT ( 'NONE',  ( 2.483409115735829786, 3.555461883994702532, -11.68352130004405431 ) ) ;
#206446=CARTESIAN_POINT ( 'NONE',  ( 2.019980081995985000, 3.974415841077576061, -11.36314192354172370 ) ) ;
#206464=ORIENTED_EDGE ( 'NONE', *, *, #176359, .T. ) ;
#206516=CARTESIAN_POINT ( 'NONE',  ( -3.469446951953614189E-15, 3.507114751586604129, 11.99288524841339054 ) ) ;
#206526=VERTEX_POINT ( 'NONE', #4824 ) ;
#206563=CARTESIAN_POINT ( 'NONE',  ( 0.000000000000000000, -8.233137084989849086, 0.000000000000000000 ) ) ;
#206577=ORIENTED_EDGE ( 'NONE', *, *, #43574, .F. ) ;
#206622=PRESENTATION_STYLE_ASSIGNMENT (( #140610 ) ) ;
#206629=CARTESIAN_POINT ( 'NONE',  ( -10.66594405399932910, -7.024005795609703284, 0.4637852190794224949 ) ) ;
#206641=MECHANICAL_DESIGN_GEOMETRIC_PRESENTATION_REPRESENTATION('',(#109931),#33933);
#206648=LINE ( 'NONE', #58281, #106743 ) ;
#206650=ADVANCED_FACE ( 'NONE', ( #38436 ), #36287, .T. ) ;
#206659=CARTESIAN_POINT ( 'NONE',  ( 0.08058608058607380498, -8.407420853759283830, 10.99970480893082225 ) ) ;
#206682=EDGE_LOOP ( 'NONE', ( #159320, #1902, #53827, #84608, #192304 ) ) ;
#206693=CARTESIAN_POINT ( 'NONE',  ( -2.494940289813118994, 3.447199233515649386, 11.73777120880565583 ) ) ;
#206703=LINE ( 'NONE', #128739, #72624 ) ;
#206733=CARTESIAN_POINT ( 'NONE',  ( -0.07933191607319768635, -9.582912294610101966, -9.499668754598335596 ) ) ;
#206734=CARTESIAN_POINT ( 'NONE',  ( -0.3868823266961807228, 2.515145635913766053, 11.70808416779825478 ) ) ;
#206735=CARTESIAN_POINT ( 'NONE',  ( 0.000000000000000000, -7.473374494045017968, 9.579665964948883783 ) ) ;
#206746=FILL_AREA_STYLE_COLOUR ( '', #162537 ) ;
#206784=AXIS2_PLACEMENT_3D ( 'NONE', #8280, #170785, #139373 ) ;
#206785=AXIS2_PLACEMENT_3D ( 'NONE', #159158, #63787, #195932 ) ;
#206830=DIRECTION ( 'NONE',  ( 0.000000000000000000, 1.000000000000000000, 0.000000000000000000 ) ) ;
#206831=CIRCLE ( 'NONE', #110128, 10.91999999999999105 ) ;
#206891=FACE_OUTER_BOUND ( 'NONE', #94305, .T. ) ;
#206919=CARTESIAN_POINT ( 'NONE',  ( 9.579665964948882007, -7.473374494045003757, 1.734723475976807094E-15 ) ) ;
#206929=CIRCLE ( 'NONE', #72090, 0.07999999999999948819 ) ;
#206949=CARTESIAN_POINT ( 'NONE',  ( -10.96785329849812562, -5.223431457505089526, 0.4373225248172959434 ) ) ;
#206959=DIRECTION ( 'NONE',  ( -0.9962287396576089415, -0.08676576675286086504, 0.000000000000000000 ) ) ;
#206975=ORIENTED_EDGE ( 'NONE', *, *, #151857, .F. ) ;
#206986=VERTEX_POINT ( 'NONE', #23227 ) ;
#207002=LINE ( 'NONE', #58633, #202142 ) ;
#207024=CARTESIAN_POINT ( 'NONE',  ( -7.800371912476627756, -5.581885079358433366, -7.755938900619404386 ) ) ;
#207029=CARTESIAN_POINT ( 'NONE',  ( 11.00057242252828260, -6.459673408256681348, -0.07917133907639190005 ) ) ;
#207035=DIRECTION ( 'NONE',  ( -0.000000000000000000, -1.000000000000000000, -0.000000000000000000 ) ) ;
#207054=CARTESIAN_POINT ( 'NONE',  ( -0.02890288085937701978, -9.971207159576024992, -9.579616049094559216 ) ) ;
#207057=ORIENTED_EDGE ( 'NONE', *, *, #140442, .T. ) ;
#207084=B_SPLINE_CURVE_WITH_KNOTS ( 'NONE', 3,
 ( #185041, #87569, #152559, #5208, #7358, #38816, #21461 ),
 .UNSPECIFIED., .F., .F.,
 ( 4, 3, 4 ),
 ( 3.314949680323544927E-05, 0.0009000000012044580581, 0.001958074173707496923 ),
 .UNSPECIFIED. ) ;
#207104=EDGE_CURVE ( 'NONE', #144299, #183707, #43801, .T. ) ;
#207171=ORIENTED_EDGE ( 'NONE', *, *, #7685, .T. ) ;
#207174=DIRECTION ( 'NONE',  ( -0.1470157664651973450, 0.7071067811865536790, 0.6916548014802195166 ) ) ;
#207182=AXIS2_PLACEMENT_3D ( 'NONE', #118296, #116162, #179 ) ;
#207208=CARTESIAN_POINT ( 'NONE',  ( -7.385065802799712031, -6.893137084989842123, -8.044078759455182137 ) ) ;
#207235=FACE_OUTER_BOUND ( 'NONE', #103648, .T. ) ;
#207240=EDGE_LOOP ( 'NONE', ( #121850, #5287, #61953, #130242, #89950, #187815 ) ) ;
#207247=EDGE_CURVE ( 'NONE', #55414, #114731, #16905, .T. ) ;
#207253=CARTESIAN_POINT ( 'NONE',  ( -10.40709887848274562, 1.794419290072776896, 5.561702625701074432 ) ) ;
#207265=ORIENTED_EDGE ( 'NONE', *, *, #155215, .T. ) ;
#207278=CARTESIAN_POINT ( 'NONE',  ( 11.41267819554179042, 3.447199233515649386, -3.708203932499494648 ) ) ;
#207280=CARTESIAN_POINT ( 'NONE',  ( 7.518896314322763175, -5.199789852012120406, 8.029456579251585069 ) ) ;
#207291=CARTESIAN_POINT ( 'NONE',  ( 0.000000000000000000, -5.166862915010145052, 0.000000000000000000 ) ) ;
#207294=DIRECTION ( 'NONE',  ( 0.000000000000000000, 0.000000000000000000, 1.000000000000000000 ) ) ;
#207315=EDGE_CURVE ( 'NONE', #189233, #145242, #37739, .T. ) ;
#207338=FACE_OUTER_BOUND ( 'NONE', #191167, .T. ) ;
#207357=CARTESIAN_POINT ( 'NONE',  ( -2.505492374191539362, 3.019799309333035975, 11.78741486269014516 ) ) ;
#207416=CARTESIAN_POINT ( 'NONE',  ( 7.721398836998391246, -5.907420853759296264, 7.721398836998372595 ) ) ;
#207440=DIRECTION ( 'NONE',  ( -0.000000000000000000, -1.000000000000000000, -0.000000000000000000 ) ) ;
#207452=AXIS2_PLACEMENT_3D ( 'NONE', #130219, #29450, #213492 ) ;
#207483=CARTESIAN_POINT ( 'NONE',  ( -0.04341786867410972472, -5.575210796978270267, 11.00023563321887643 ) ) ;
#207493=ORIENTED_EDGE ( 'NONE', *, *, #201124, .F. ) ;
#207499=ORIENTED_EDGE ( 'NONE', *, *, #181839, .F. ) ;
#207501=EDGE_CURVE ( 'NONE', #121080, #104249, #205749, .T. ) ;
#207502=ORIENTED_EDGE ( 'NONE', *, *, #22175, .T. ) ;
#207512=CARTESIAN_POINT ( 'NONE',  ( 2.315885204923604057, 3.829536045110822684, -11.43841291973004992 ) ) ;
#207522=ORIENTED_EDGE ( 'NONE', *, *, #190633, .T. ) ;
#207536=CARTESIAN_POINT ( 'NONE',  ( -0.1531059978909564412, -6.764708007038255921, -10.99917004716958857 ) ) ;
#207563=EDGE_CURVE ( 'NONE', #133392, #209973, #54969, .T. ) ;
#207573=DIRECTION ( 'NONE',  ( -0.03984146075563027578, 0.000000000000000000, 0.9992060137953822085 ) ) ;
#207669=CARTESIAN_POINT ( 'NONE',  ( -6.783773251375875724, -6.684699875907230471, 6.634380621478824125 ) ) ;
#207690=CARTESIAN_POINT ( 'NONE',  ( 10.91927143613603945, -9.998067526917994385, -0.1131244342389418484 ) ) ;
#207703=VERTEX_POINT ( 'NONE', #10145 ) ;
#207710=DIRECTION ( 'NONE',  ( 0.000000000000000000, 1.000000000000000000, 0.000000000000000000 ) ) ;
#207729=CARTESIAN_POINT ( 'NONE',  ( -0.1360919303236346745, -7.795524846228471638, 10.99936842639231571 ) ) ;
#207792=CARTESIAN_POINT ( 'NONE',  ( 0.1981138333790652684, -9.280569609800584985, -9.498748750704418597 ) ) ;
#207806=PRESENTATION_STYLE_ASSIGNMENT (( #43216 ) ) ;
#207812=CARTESIAN_POINT ( 'NONE',  ( -7.037870247915987143, -8.199999999999986855, 6.381095703207952496 ) ) ;
#207870=VERTEX_POINT ( 'NONE', #61042 ) ;
#207888=ORIENTED_EDGE ( 'NONE', *, *, #118553, .F. ) ;
#207905=CARTESIAN_POINT ( 'NONE',  ( -0.08269815893113435790, -5.360092950639682385, -10.99976946526262900 ) ) ;
#207919=CARTESIAN_POINT ( 'NONE',  ( -1.355252715606880543E-15, 3.019799309333170978, 12.05075272264442177 ) ) ;
#207955=EDGE_LOOP ( 'NONE', ( #189553, #15245, #61614, #142652 ) ) ;
#207981=CARTESIAN_POINT ( 'NONE',  ( -10.02012520139310681, 1.794419290072776896, -6.231960695612073664 ) ) ;
#208043=FACE_OUTER_BOUND ( 'NONE', #200466, .T. ) ;
#208054=CARTESIAN_POINT ( 'NONE',  ( -10.98194350564911481, -7.666862915010147717, 0.6300133639306313427 ) ) ;
#208174=CARTESIAN_POINT ( 'NONE',  ( -1.138412281109779656E-15, -8.526088927970992160, 10.80093815994596262 ) ) ;
#208229=VERTEX_POINT ( 'NONE', #107728 ) ;
#208240=AXIS2_PLACEMENT_3D ( 'NONE', #56164, #122328, #185072 ) ;
#208257=EDGE_CURVE ( 'NONE', #182623, #192862, #79240, .T. ) ;
#208263=CARTESIAN_POINT ( 'NONE',  ( -0.02191186323001123593, -9.962467934940974601, -10.91967397018793129 ) ) ;
#208295=ORIENTED_EDGE ( 'NONE', *, *, #202413, .T. ) ;
#208297=AXIS2_PLACEMENT_3D ( 'NONE', #173440, #188592, #189656 ) ;
#208304=ORIENTED_EDGE ( 'NONE', *, *, #107978, .T. ) ;
#208314=EDGE_LOOP ( 'NONE', ( #193825, #76935, #212404, #133129 ) ) ;
#208329=ORIENTED_EDGE ( 'NONE', *, *, #139632, .T. ) ;
#208336=CARTESIAN_POINT ( 'NONE',  ( -9.499700864329909678, -7.154544010627095219, -0.07538891330675204228 ) ) ;
#208356=CIRCLE ( 'NONE', #31972, 0.08000000000000020983 ) ;
#208358=AXIS2_PLACEMENT_3D ( 'NONE', #73835, #144222, #210216 ) ;
#208362=CARTESIAN_POINT ( 'NONE',  ( 0.09005296632881229502, -9.916958724994124452, 10.99963137851698924 ) ) ;
#208367=CARTESIAN_POINT ( 'NONE',  ( 10.91962425643199985, -9.999999999999994671, -0.09058751758333170867 ) ) ;
#208381=EDGE_CURVE ( 'NONE', #156, #78199, #102407, .T. ) ;
#208388=DIRECTION ( 'NONE',  ( 0.000000000000000000, -1.000000000000000000, 0.000000000000000000 ) ) ;
#208445=CIRCLE ( 'NONE', #66492, 9.616019636405020776 ) ;
#208534=CARTESIAN_POINT ( 'NONE',  ( 0.3617173305617603640, -5.199791778942882026, 10.99431798667029803 ) ) ;
#208541=B_SPLINE_CURVE_WITH_KNOTS ( 'NONE', 3,
 ( #169977, #38922, #204589, #151622, #101790, #185151, #85532, #3188 ),
 .UNSPECIFIED., .F., .F.,
 ( 4, 2, 2, 4 ),
 ( 2.602085213965248775E-18, 0.0002461874215021552068, 0.0004923748430043078115, 0.0009847496860086130208 ),
 .UNSPECIFIED. ) ;
#208553=ORIENTED_EDGE ( 'NONE', *, *, #118098, .F. ) ;
#208554=CARTESIAN_POINT ( 'NONE',  ( -9.579665964935227151, -7.246166700194470067, 0.000000000000000000 ) ) ;
#208586=CARTESIAN_POINT ( 'NONE',  ( -0.07917133907641019097, -6.459673408256690230, -11.00057242252814760 ) ) ;
#208589=CARTESIAN_POINT ( 'NONE',  ( 0.000000000000000000, 4.000000000000003553, -11.99999999999999112 ) ) ;
#208590=( BOUNDED_SURFACE ( )  B_SPLINE_SURFACE ( 3, 2, ( 
 ( #38342, #170466, #57793 ),
 ( #26348, #5803, #7957 ),
 ( #122897, #125016, #91386 ),
 ( #24201, #106597, #137989 ) ),
 .UNSPECIFIED., .F., .F., .T. ) 
 B_SPLINE_SURFACE_WITH_KNOTS ( ( 4, 4 ),
 ( 3, 3 ),
 ( 0.000000000000000000, 3.124373798653399658E-05 ),
 ( 0.000000000000000000, 1.000000000000000000 ),
 .UNSPECIFIED. ) 
 GEOMETRIC_REPRESENTATION_ITEM ( )  RATIONAL_B_SPLINE_SURFACE ( (
 ( 1.000000000000000000, 0.7071067811870779263, 1.000000000000000000),
 ( 1.000000000000000000, 0.7053575014263694376, 1.000000000000000000),
 ( 1.000000000000000000, 0.7044883013754974499, 1.000000000000000000),
 ( 1.000000000000000000, 0.7045118851642885316, 1.000000000000000000) ) ) 
 REPRESENTATION_ITEM ( '' )  SURFACE ( )  );
#208592=CIRCLE ( 'NONE', #97941, 10.99999999999999112 ) ;
#208621=EDGE_LOOP ( 'NONE', ( #171556, #123568, #15707, #146147 ) ) ;
#208659=CIRCLE ( 'NONE', #98006, 0.07999999999999940492 ) ;
#208662=ORIENTED_EDGE ( 'NONE', *, *, #152831, .F. ) ;
#208685=B_SPLINE_CURVE_WITH_KNOTS ( 'NONE', 3,
 ( #98236, #164291, #15879, #148049, #65685, #131832, #99299, #16942, #83021, #66743 ),
 .UNSPECIFIED., .F., .F.,
 ( 4, 2, 2, 2, 4 ),
 ( 0.000000000000000000, 0.0002334048330869045729, 0.0004668096661738091457, 0.0007002144992607138270, 0.0009336193323476185083 ),
 .UNSPECIFIED. ) ;
#208716=EDGE_CURVE ( 'NONE', #16492, #206986, #33917, .T. ) ;
#208726=EDGE_LOOP ( 'NONE', ( #171243, #162596, #18098, #14171, #159818 ) ) ;
#208730=ORIENTED_EDGE ( 'NONE', *, *, #108052, .F. ) ;
#208744=FACE_OUTER_BOUND ( 'NONE', #21780, .T. ) ;
#208750=LINE ( 'NONE', #128676, #317 ) ;
#208757=CARTESIAN_POINT ( 'NONE',  ( -6.776587425048114177, -7.030236945366979739, -6.796206128891399523 ) ) ;
#208758=EDGE_LOOP ( 'NONE', ( #131005, #122194, #160923, #151074, #59293 ) ) ;
#208782=CARTESIAN_POINT ( 'NONE',  ( 9.568546172724150978, -8.233137084989836652, -0.4683205530892405877 ) ) ;
#208806=ORIENTED_EDGE ( 'NONE', *, *, #95154, .T. ) ;
#208810=CARTESIAN_POINT ( 'NONE',  ( -2.493461049780994365, 3.507114751586604129, 11.73081193161140590 ) ) ;
#208816=ADVANCED_FACE ( 'NONE', ( #5597 ), #203811, .T. ) ;
#208839=CARTESIAN_POINT ( 'NONE',  ( 9.606148981167590861, -6.583980363595129504, -0.4355862708379804604 ) ) ;
#208871=ORIENTED_EDGE ( 'NONE', *, *, #89214, .T. ) ;
#208955=ADVANCED_FACE ( 'NONE', ( #83676 ), #58049, .T. ) ;
#208961=FACE_OUTER_BOUND ( 'NONE', #198411, .T. ) ;
#208962=ORIENTED_EDGE ( 'NONE', *, *, #78852, .T. ) ;
#208982=FACE_OUTER_BOUND ( 'NONE', #170400, .T. ) ;
#209023=CIRCLE ( 'NONE', #195297, 0.08000000000000020983 ) ;
#209050=CARTESIAN_POINT ( 'NONE',  ( 0.000000000000000000, 0.2000000000000057288, -11.50000000000000000 ) ) ;
#209064=CARTESIAN_POINT ( 'NONE',  ( 6.726765607527583235, -8.198316282514454656, 6.726765607527558366 ) ) ;
#209097=CARTESIAN_POINT ( 'NONE',  ( 7.586009164902111301, -6.657020681837064302, 7.796438949605565938 ) ) ;
#209100=ORIENTED_EDGE ( 'NONE', *, *, #213856, .F. ) ;
#209105=ORIENTED_EDGE ( 'NONE', *, *, #78185, .F. ) ;
#209115=VECTOR ( 'NONE', #52012, 1000.000000000000000 ) ;
#209117=FACE_OUTER_BOUND ( 'NONE', #74862, .T. ) ;
#209174=CARTESIAN_POINT ( 'NONE',  ( -7.772296586883777003, -5.601927612791864242, -7.784592198500460469 ) ) ;
#209177=ORIENTED_EDGE ( 'NONE', *, *, #98691, .T. ) ;
#209183=CARTESIAN_POINT ( 'NONE',  ( 7.752014238602739730E-16, 3.079999999999999183, 6.329999999999995630 ) ) ;
#209258=CARTESIAN_POINT ( 'NONE',  ( -10.99970480893081692, -5.740513804456437441, -0.08058608058607553970 ) ) ;
#209327=CARTESIAN_POINT ( 'NONE',  ( 7.725699985795420055, -5.832912386296867702, 7.725699985795402291 ) ) ;
#209328=VERTEX_POINT ( 'NONE', #27214 ) ;
#209352=CARTESIAN_POINT ( 'NONE',  ( -6.392587740394328755, -6.532648833121157850, -6.999862025036979851 ) ) ;
#209394=CARTESIAN_POINT ( 'NONE',  ( -9.488025208946957889, -6.683951901172175525, 0.1062647697984211714 ) ) ;
#209419=CARTESIAN_POINT ( 'NONE',  ( 0.1007326007325878847, -9.919999999999998153, 10.99953876047308476 ) ) ;
#209470=FILL_AREA_STYLE ('',( #6993 ) ) ;
#209539=ORIENTED_EDGE ( 'NONE', *, *, #102049, .T. ) ;
#209622=VECTOR ( 'NONE', #156973, 1000.000000000000000 ) ;
#209631=VECTOR ( 'NONE', #47197, 1000.000000000000000 ) ;
#209664=ORIENTED_EDGE ( 'NONE', *, *, #10396, .F. ) ;
#209670=DIRECTION ( 'NONE',  ( 0.000000000000000000, 0.000000000000000000, 1.000000000000000000 ) ) ;
#209677=CARTESIAN_POINT ( 'NONE',  ( -1.040834085586084257E-14, -7.242250812739412957, 9.811039896441885233 ) ) ;
#209695=AXIS2_PLACEMENT_3D ( 'NONE', #102804, #140404, #26608 ) ;
#209749=CARTESIAN_POINT ( 'NONE',  ( -9.578206935422265644, -9.900000000000005684, 0.1671882239536719994 ) ) ;
#209752=CARTESIAN_POINT ( 'NONE',  ( 7.173763318589350568, -6.681223591463127498, 7.173763318589327476 ) ) ;
#209776=CARTESIAN_POINT ( 'NONE',  ( 10.91255906795568364, 3.426985321572577181, -3.952372590954820630 ) ) ;
#209830=DIRECTION ( 'NONE',  ( 0.000000000000000000, 1.000000000000000000, 0.000000000000000000 ) ) ;
#209845=CARTESIAN_POINT ( 'NONE',  ( -9.623574082427422738, -9.090902906714937615, 0.4644248560400319747 ) ) ;
#209853=CARTESIAN_POINT ( 'NONE',  ( 0.000000000000000000, -8.407420853759283830, 10.91970695577495931 ) ) ;
#209897=EDGE_LOOP ( 'NONE', ( #99711, #64883, #37795, #24302 ) ) ;
#209909=CARTESIAN_POINT ( 'NONE',  ( 9.499050059654537748, -8.104757123234188398, -0.1520312049662329856 ) ) ;
#209915=CARTESIAN_POINT ( 'NONE',  ( 10.99970480893080627, -5.907420853759282053, 0.08058608058608522640 ) ) ;
#209950=ORIENTED_EDGE ( 'NONE', *, *, #34900, .T. ) ;
#209970=CARTESIAN_POINT ( 'NONE',  ( -11.34781316621061009, 4.021557182957057996, 3.687128006872979924 ) ) ;
#209973=VERTEX_POINT ( 'NONE', #158308 ) ;
#209980=B_SPLINE_CURVE_WITH_KNOTS ( 'NONE', 3,
 ( #137708, #93237, #175540, #189635, #203729, #56447, #40201 ),
 .UNSPECIFIED., .F., .F.,
 ( 4, 3, 4 ),
 ( 0.0001135037245265641654, 0.001517139415464318795, 0.002007692284160929319 ),
 .UNSPECIFIED. ) ;
#210014=CARTESIAN_POINT ( 'NONE',  ( 7.721398836998350390, -5.907420853759296264, -7.721398836998385917 ) ) ;
#210041=CARTESIAN_POINT ( 'NONE',  ( -6.720112740279242658, -7.154544010627095219, 6.827626583076779276 ) ) ;
#210043=CARTESIAN_POINT ( 'NONE',  ( -0.3868239129444561164, 2.972657967446814542, 11.65375889120575614 ) ) ;
#210048=CARTESIAN_POINT ( 'NONE',  ( -10.30245174296173793, 3.603753425775782393, 5.948123287112152546 ) ) ;
#210108=CARTESIAN_POINT ( 'NONE',  ( 10.32992389895506413, 1.000000000000000888, 6.106772653521394645 ) ) ;
#210137=CARTESIAN_POINT ( 'NONE',  ( 6.389500218612170990, -8.186910008818841789, 7.047919418996371199 ) ) ;
#210164=ORIENTED_EDGE ( 'NONE', *, *, #182674, .T. ) ;
#210172=VERTEX_POINT ( 'NONE', #146338 ) ;
#210183=FILL_AREA_STYLE ('',( #110641 ) ) ;
#210216=DIRECTION ( 'NONE',  ( 0.000000000000000000, 0.000000000000000000, 1.000000000000000000 ) ) ;
#210232=CIRCLE ( 'NONE', #148102, 11.49999999999998934 ) ;
#210250=ORIENTED_EDGE ( 'NONE', *, *, #127713, .T. ) ;
#210279=ORIENTED_EDGE ( 'NONE', *, *, #54844, .T. ) ;
#210303=UNCERTAINTY_MEASURE_WITH_UNIT (LENGTH_MEASURE( 1.000000000000000082E-05 ), #71987, 'distance_accuracy_value', 'NONE');
#210330=ORIENTED_EDGE ( 'NONE', *, *, #131984, .T. ) ;
#210374=CARTESIAN_POINT ( 'NONE',  ( -10.48884024596653397, 1.000000000000000888, 5.608780650328914597 ) ) ;
#210400=FILL_AREA_STYLE ('',( #176851 ) ) ;
#210437=FACE_OUTER_BOUND ( 'NONE', #188428, .T. ) ;
#210459=DIRECTION ( 'NONE',  ( -0.9989777552170298058, -5.711963089865910869E-16, -0.04520447523801467832 ) ) ;
#210461=EDGE_CURVE ( 'NONE', #166319, #179385, #23706, .T. ) ;
#210489=B_SPLINE_CURVE_WITH_KNOTS ( 'NONE', 3,
 ( #57299, #189426, #10657, #11725, #191540, #41067, #125578 ),
 .UNSPECIFIED., .F., .F.,
 ( 4, 3, 4 ),
 ( 0.0001126021370637016465, 0.0006031550062628992376, 0.002006790698585265206 ),
 .UNSPECIFIED. ) ;
#210519=CARTESIAN_POINT ( 'NONE',  ( -7.446209719563359641, -5.223431457505076203, -8.064677165291183059 ) ) ;
#210527=( GEOMETRIC_REPRESENTATION_CONTEXT ( 3 ) GLOBAL_UNCERTAINTY_ASSIGNED_CONTEXT ( ( #1684 ) ) GLOBAL_UNIT_ASSIGNED_CONTEXT ( ( #105985, #23597, #178409 ) ) REPRESENTATION_CONTEXT ( 'NONE', 'WORKASPACE' ) );
#210635=FACE_OUTER_BOUND ( 'NONE', #35298, .T. ) ;
#210687=CIRCLE ( 'NONE', #193531, 11.54340198673881979 ) ;
#210702=ADVANCED_FACE ( 'NONE', ( #18419 ), #67151, .T. ) ;
#210735=AXIS2_PLACEMENT_3D ( 'NONE', #125993, #79296, #43617 ) ;
#210780=CARTESIAN_POINT ( 'NONE',  ( -7.720982897393583677, -5.823938088759706311, 7.834948825496934610 ) ) ;
#210810=CARTESIAN_POINT ( 'NONE',  ( 0.000000000000000000, -9.999999999999994671, 0.000000000000000000 ) ) ;
#210854=CARTESIAN_POINT ( 'NONE',  ( -0.4366903032815979135, -8.287795860939835890, 10.40306649911375736 ) ) ;
#210864=ORIENTED_EDGE ( 'NONE', *, *, #131239, .F. ) ;
#210866=CARTESIAN_POINT ( 'NONE',  ( -1.040834085586084257E-14, 0.000000000000000000, -9.579665964948867796 ) ) ;
#210890=CARTESIAN_POINT ( 'NONE',  ( 8.832353407160718817, 3.956598013261175772, 7.432338980325266853 ) ) ;
#210893=ADVANCED_FACE ( 'NONE', ( #185177 ), #78858, .F. ) ;
#210977=CYLINDRICAL_SURFACE ( 'NONE', #137549, 8.049999999999993605 ) ;
#210978=CIRCLE ( 'NONE', #6892, 0.08000000000000020983 ) ;
#211010=APPLICATION_CONTEXT ( 'automotive_design' ) ;
#211020=CARTESIAN_POINT ( 'NONE',  ( 0.1370650511771386582, -7.902328468025380914, -10.96100467917833221 ) ) ;
#211023=FILL_AREA_STYLE ('',( #64785 ) ) ;
#211108=CARTESIAN_POINT ( 'NONE',  ( -0.1288460037566284688, -8.008893676011963336, -9.499262961676866013 ) ) ;
#211125=CARTESIAN_POINT ( 'NONE',  ( -0.07933191752142512709, -7.643695121331865572, 9.499668754586258146 ) ) ;
#211135=ORIENTED_EDGE ( 'NONE', *, *, #5562, .F. ) ;
#211202=AXIS2_PLACEMENT_3D ( 'NONE', #66377, #101034, #36034 ) ;
#211236=CARTESIAN_POINT ( 'NONE',  ( 7.547439985188200140, -6.717993526550342764, 7.827294160508124321 ) ) ;
#211237=CARTESIAN_POINT ( 'NONE',  ( 6.725651841507260364, -7.791858861492839239, -6.710064404886719736 ) ) ;
#211250=DIRECTION ( 'NONE',  ( 0.000000000000000000, -1.000000000000000000, 0.000000000000000000 ) ) ;
#211252=CARTESIAN_POINT ( 'NONE',  ( -10.94305301526627439, -8.100264386820972717, 0.2223449190352171922 ) ) ;
#211265=EDGE_CURVE ( 'NONE', #21086, #183752, #206929, .T. ) ;
#211310=EDGE_LOOP ( 'NONE', ( #94842, #123676, #113062, #64238 ) ) ;
#211320=CARTESIAN_POINT ( 'NONE',  ( -11.21996551234719774, 1.000000000000000888, 3.949207502427040772 ) ) ;
#211396=DIRECTION ( 'NONE',  ( 0.000000000000000000, 1.000000000000000000, 0.000000000000000000 ) ) ;
#211495=ADVANCED_FACE ( 'NONE', ( #137531 ), #92825, .T. ) ;
#211546=CARTESIAN_POINT ( 'NONE',  ( 0.000000000000000000, -9.999999999999994671, 0.000000000000000000 ) ) ;
#211633=ORIENTED_EDGE ( 'NONE', *, *, #202732, .T. ) ;
#211690=CARTESIAN_POINT ( 'NONE',  ( -1.040834085586084257E-14, -9.746166700180788567, -9.579665964948867796 ) ) ;
#211698=DIRECTION ( 'NONE',  ( 0.000000000000000000, 1.000000000000000000, 0.000000000000000000 ) ) ;
#211764=AXIS2_PLACEMENT_3D ( 'NONE', #99938, #83668, #79419 ) ;
#211786=CARTESIAN_POINT ( 'NONE',  ( 6.773846765317333762, -7.552951973956472997, 6.773846765317311558 ) ) ;
#211817=DIRECTION ( 'NONE',  ( 0.000000000000000000, 0.000000000000000000, 1.000000000000000000 ) ) ;
#211832=( NAMED_UNIT ( * ) SI_UNIT ( $, .STERADIAN. ) SOLID_ANGLE_UNIT ( ) );
#211847=AXIS2_PLACEMENT_3D ( 'NONE', #37499, #73182, #74280 ) ;
#211867=CARTESIAN_POINT ( 'NONE',  ( 0.000000000000000000, 0.000000000000000000, 0.000000000000000000 ) ) ;
#211912=DIRECTION ( 'NONE',  ( 0.000000000000000000, -1.000000000000000000, 0.000000000000000000 ) ) ;
#211917=CIRCLE ( 'NONE', #173932, 11.99999999999999112 ) ;
#211923=DIRECTION ( 'NONE',  ( 0.000000000000000000, 1.000000000000000000, 0.000000000000000000 ) ) ;
#211931=ORIENTED_EDGE ( 'NONE', *, *, #147046, .F. ) ;
#211939=CARTESIAN_POINT ( 'NONE',  ( -5.204170427930421283E-15, -5.907420853759282053, 10.91970695577496997 ) ) ;
#211941=ORIENTED_EDGE ( 'NONE', *, *, #83989, .T. ) ;
#212002=ORIENTED_EDGE ( 'NONE', *, *, #175718, .F. ) ;
#212037=CARTESIAN_POINT ( 'NONE',  ( 9.499633399276474321, -8.038540703696423151, -0.09463244300327215697 ) ) ;
#212040=FACE_OUTER_BOUND ( 'NONE', #2865, .T. ) ;
#212049=EDGE_CURVE ( 'NONE', #177991, #147438, #151122, .T. ) ;
#212066=ORIENTED_EDGE ( 'NONE', *, *, #104440, .F. ) ;
#212082=CARTESIAN_POINT ( 'NONE',  ( 0.3532572990641478228, -7.666862990898835051, -10.99465531782955985 ) ) ;
#212086=DIRECTION ( 'NONE',  ( 0.000000000000000000, 1.000000000000000000, 0.000000000000000000 ) ) ;
#212129=UNCERTAINTY_MEASURE_WITH_UNIT (LENGTH_MEASURE( 1.000000000000000082E-05 ), #52892, 'distance_accuracy_value', 'NONE');
#212186=VERTEX_POINT ( 'NONE', #202228 ) ;
#212189=CARTESIAN_POINT ( 'NONE',  ( -3.680781672293562123E-15, -7.473374494045017080, 9.500331257164628340 ) ) ;
#212210=CONICAL_SURFACE ( 'NONE', #118902, 6.540947088288920241, 0.7853981633974536081 ) ;
#212244=CARTESIAN_POINT ( 'NONE',  ( 9.858406733136194415E-16, 1.000000000000000888, -8.050000000000000711 ) ) ;
#212249=CARTESIAN_POINT ( 'NONE',  ( -7.004500933659075557, -6.920331743269713343, -7.004500933659044470 ) ) ;
#212277=EDGE_LOOP ( 'NONE', ( #197663, #29224 ) ) ;
#212304=CARTESIAN_POINT ( 'NONE',  ( 9.000007961041747606, 1.000000000000000888, 7.937244906211794238 ) ) ;
#212320=FILL_AREA_STYLE_COLOUR ( '', #15689 ) ;
#212373=CARTESIAN_POINT ( 'NONE',  ( -9.512045263456270661, -8.176568542494905500, 0.4655551865852137206 ) ) ;
#212375=B_SPLINE_CURVE_WITH_KNOTS ( 'NONE', 3,
 ( #26073, #190700, #158236, #9826 ),
 .UNSPECIFIED., .F., .F.,
 ( 4, 4 ),
 ( 0.0005671806269306270149, 0.0008743016172331019402 ),
 .UNSPECIFIED. ) ;
#212404=ORIENTED_EDGE ( 'NONE', *, *, #203566, .T. ) ;
#212430=EDGE_CURVE ( 'NONE', #170100, #125304, #140793, .T. ) ;
#212434=DIRECTION ( 'NONE',  ( -0.000000000000000000, 1.000000000000000000, -0.000000000000000000 ) ) ;
#212442=CARTESIAN_POINT ( 'NONE',  ( -6.796618584846395805, -7.026643280347676601, 6.776593369754376539 ) ) ;
#212558=CARTESIAN_POINT ( 'NONE',  ( 10.96785329849812562, -5.223431457505089526, -0.4373225248172959434 ) ) ;
#212577=CARTESIAN_POINT ( 'NONE',  ( 7.836475020641954004, -5.360178282914183967, -7.719547554928811728 ) ) ;
#212606=CARTESIAN_POINT ( 'NONE',  ( -9.491250020638663187, -6.775781654326522130, 0.2167848519283762654 ) ) ;
#212633=DIRECTION ( 'NONE',  ( 0.000000000000000000, 0.000000000000000000, 1.000000000000000000 ) ) ;
#212646=CARTESIAN_POINT ( 'NONE',  ( -11.02381569330256283, 2.441452740530747789, 3.988656969163915100 ) ) ;
#212647=CARTESIAN_POINT ( 'NONE',  ( -10.91970695577495931, 0.000000000000000000, 0.000000000000000000 ) ) ;
#212733=( GEOMETRIC_REPRESENTATION_CONTEXT ( 3 ) GLOBAL_UNCERTAINTY_ASSIGNED_CONTEXT ( ( #14992 ) ) GLOBAL_UNIT_ASSIGNED_CONTEXT ( ( #112474, #12751, #195792 ) ) REPRESENTATION_CONTEXT ( 'NONE', 'WORKASPACE' ) );
#212798=CARTESIAN_POINT ( 'NONE',  ( -10.99126615174920474, -5.166862915010145052, 0.4382560683119315903 ) ) ;
#212804=CIRCLE ( 'NONE', #157488, 10.91999999999999105 ) ;
#212863=DIRECTION ( 'NONE',  ( 0.000000000000000000, 1.000000000000000000, 0.000000000000000000 ) ) ;
#212901=FILL_AREA_STYLE_COLOUR ( '', #181897 ) ;
#212973=CARTESIAN_POINT ( 'NONE',  ( 11.02381569330252908, 2.441452740530748233, -3.988656969163989707 ) ) ;
#212977=TOROIDAL_SURFACE ( 'NONE', #133559, 11.29999999999999893, 0.2000000000000000111 ) ;
#212983=CARTESIAN_POINT ( 'NONE',  ( 10.38813158755803556, 2.629643693813619620, 6.007251501586638121 ) ) ;
#213004=EDGE_CURVE ( 'NONE', #90309, #107434, #196738, .T. ) ;
#213011=CARTESIAN_POINT ( 'NONE',  ( -0.4350687514514811616, -5.166862915010145052, -10.91132967064556425 ) ) ;
#213015=CARTESIAN_POINT ( 'NONE',  ( -11.06389876992414578, 3.829536045110820464, 3.713591040152699030 ) ) ;
#213028=CIRCLE ( 'NONE', #112782, 11.49999999999998934 ) ;
#213062=( BOUNDED_SURFACE ( )  B_SPLINE_SURFACE ( 3, 2, ( 
 ( #87839, #73712, #22805 ),
 ( #188527, #139810, #202624 ),
 ( #170143, #53201, #186386 ),
 ( #55336, #38023, #120411 ),
 ( #171211, #157116, #119332 ),
 ( #20677, #185319, #41240 ),
 ( #122565, #6558, #8705 ),
 ( #153910, #105174, #169078 ) ),
 .UNSPECIFIED., .F., .F., .T. ) 
 B_SPLINE_SURFACE_WITH_KNOTS ( ( 4, 2, 2, 4 ),
 ( 3, 3 ),
 ( 0.000000000000000000, 0.0004924884914732730132, 0.0007387327372099095199, 0.0009849769829465460265 ),
 ( 0.000000000000000000, 1.000000000000000000 ),
 .UNSPECIFIED. ) 
 GEOMETRIC_REPRESENTATION_ITEM ( )  RATIONAL_B_SPLINE_SURFACE ( (
 ( 1.000000000000000000, 0.7045118851637662827, 1.000000000000000000),
 ( 1.000000000000000000, 0.7593505504062139089, 1.000000000000000000),
 ( 1.000000000000000000, 0.8104906253036173736, 1.000000000000000000),
 ( 1.000000000000000000, 0.8722646935499589471, 1.000000000000000000),
 ( 1.000000000000000000, 0.8905178607894793652, 1.000000000000000000),
 ( 1.000000000000000000, 0.9170530604353642756, 1.000000000000000000),
 ( 1.000000000000000000, 0.9248184710077380632, 1.000000000000000000),
 ( 1.000000000000000000, 0.9238795325112880708, 1.000000000000000000) ) ) 
 REPRESENTATION_ITEM ( '' )  SURFACE ( )  );
#213072=PRESENTATION_STYLE_ASSIGNMENT (( #164346 ) ) ;
#213074=CARTESIAN_POINT ( 'NONE',  ( -9.481348452320373710, -9.006862915010128035, 0.5950054837411764552 ) ) ;
#213100=ORIENTED_EDGE ( 'NONE', *, *, #158732, .F. ) ;
#213124=FACE_OUTER_BOUND ( 'NONE', #203545, .T. ) ;
#213152=CARTESIAN_POINT ( 'NONE',  ( 0.2721095781817989834, -7.697284395437333337, -10.99684423689256008 ) ) ;
#213157=CARTESIAN_POINT ( 'NONE',  ( 9.579592329539993401, -9.999999999999994671, -0.07839159645131119070 ) ) ;
#213219=CARTESIAN_POINT ( 'NONE',  ( -2.486770427477412948, 2.630042260599927850, 11.73951962969540297 ) ) ;
#213222=DIRECTION ( 'NONE',  ( 0.000000000000000000, 0.000000000000000000, 1.000000000000000000 ) ) ;
#213251=CARTESIAN_POINT ( 'NONE',  ( -10.98598255107576627, -7.721050908199745599, 0.1917610387292554008 ) ) ;
#213252=CIRCLE ( 'NONE', #178812, 0.07999999999999980738 ) ;
#213266=CARTESIAN_POINT ( 'NONE',  ( -6.663994888585885512, -7.154544010627095219, 6.770610912236877610 ) ) ;
#213275=CIRCLE ( 'NONE', #137244, 0.08000000000000020983 ) ;
#213278=EDGE_CURVE ( 'NONE', #90309, #186972, #4816, .T. ) ;
#213314=CIRCLE ( 'NONE', #36914, 0.08000000000000020983 ) ;
#213329=CARTESIAN_POINT ( 'NONE',  ( -9.606148981167596190, -6.583980363595129504, 0.4355862708379978354 ) ) ;
#213361=CARTESIAN_POINT ( 'NONE',  ( 0.06712503953320783645, -9.995102581657556939, 9.579544693637551234 ) ) ;
#213362=CARTESIAN_POINT ( 'NONE',  ( -7.019253602638888090, -7.126685749119995528, -7.019253602638846345 ) ) ;
#213381=( LENGTH_UNIT ( ) NAMED_UNIT ( * ) SI_UNIT ( .MILLI., .METRE. ) );
#213396=CARTESIAN_POINT ( 'NONE',  ( -0.4294425147611594107, -9.006862915010128035, 9.490288674561789151 ) ) ;
#213438=CARTESIAN_POINT ( 'NONE',  ( -0.01315889736799453862, -9.583523248313889908, 9.500441148486922671 ) ) ;
#213455=DIRECTION ( 'NONE',  ( 0.000000000000000000, 1.000000000000000000, 0.000000000000000000 ) ) ;
#213463=CARTESIAN_POINT ( 'NONE',  ( -9.579764304849156531, -9.999999999999994671, 0.06720017513374074158 ) ) ;
#213492=DIRECTION ( 'NONE',  ( 0.000000000000000000, 0.000000000000000000, 1.000000000000000000 ) ) ;
#213551=CARTESIAN_POINT ( 'NONE',  ( 10.89523958697327011, -6.437359833193944780, -0.04208621775141048460 ) ) ;
#213558=DIRECTION ( 'NONE',  ( 0.04529798058948680123, 1.504112749676217512E-16, 0.9989735196462991018 ) ) ;
#213573=CARTESIAN_POINT ( 'NONE',  ( 0.06290936665214190426, -8.043994141378489005, -10.94971099608171627 ) ) ;
#213578=CARTESIAN_POINT ( 'NONE',  ( 10.38614328979769041, 3.507114751586604129, 5.996442624206595795 ) ) ;
#213618=DIRECTION ( 'NONE',  ( 0.000000000000000000, 1.000000000000000000, 0.000000000000000000 ) ) ;
#213650=CARTESIAN_POINT ( 'NONE',  ( 0.001121896803084446431, -7.189645481337945121, 9.584290747382876674 ) ) ;
#213682=DIRECTION ( 'NONE',  ( 0.000000000000000000, 0.000000000000000000, 1.000000000000000000 ) ) ;
#213701=CARTESIAN_POINT ( 'NONE',  ( 7.662794434365301832, -5.790678129197942781, -7.045261094876537733 ) ) ;
#213707=AXIS2_PLACEMENT_3D ( 'NONE', #17593, #68481, #84754 ) ;
#213712=VERTEX_POINT ( 'NONE', #163666 ) ;
#213762=ORIENTED_EDGE ( 'NONE', *, *, #151857, .T. ) ;
#213815=B_SPLINE_CURVE_WITH_KNOTS ( 'NONE', 3,
 ( #174588, #91198, #192924, #74930 ),
 .UNSPECIFIED., .F., .F.,
 ( 4, 4 ),
 ( 0.000000000000000000, 0.0002908967400263839909 ),
 .UNSPECIFIED. ) ;
#213856=EDGE_CURVE ( 'NONE', #187130, #170487, #195091, .T. ) ;
#213871=ORIENTED_EDGE ( 'NONE', *, *, #190098, .T. ) ;
#213910=CARTESIAN_POINT ( 'NONE',  ( -0.4373225248172924462, -7.723431457505077979, 10.96785329849814161 ) ) ;
#213919=CARTESIAN_POINT ( 'NONE',  ( 1.408343819019456176E-15, 0.2000000000000057288, 11.50000000000000000 ) ) ;
#213943=CARTESIAN_POINT ( 'NONE',  ( -7.962224162659105708, -5.254973434576998059, 7.552496594302672506 ) ) ;
#213956=CARTESIAN_POINT ( 'NONE',  ( 9.499668754385636404, -7.246166700194470067, 0.07933194154488391880 ) ) ;
#213977=CARTESIAN_POINT ( 'NONE',  ( -10.32992389895503393, 1.000000000000000888, -6.106772653521458594 ) ) ;
#214055=CARTESIAN_POINT ( 'NONE',  ( -10.85277107007939001, 3.956598013261175772, 3.932872935640539414 ) ) ;
#214068=DIRECTION ( 'NONE',  ( 0.000000000000000000, 0.000000000000000000, -1.000000000000000000 ) ) ;
#214085=CARTESIAN_POINT ( 'NONE',  ( -7.905503641038438722, -6.808400134080595301, 7.455003611050304180 ) ) ;
#214101=VERTEX_POINT ( 'NONE', #153800 ) ;
#214114=B_SPLINE_CURVE_WITH_KNOTS ( 'NONE', 3,
 ( #113879, #49862, #10, #1080 ),
 .UNSPECIFIED., .F., .F.,
 ( 4, 4 ),
 ( 0.000000000000000000, 0.0002908967400263839909 ),
 .UNSPECIFIED. ) ;
#214160=CARTESIAN_POINT ( 'NONE',  ( 6.773376348128858915, -7.215568602681178945, 6.661184042391304239 ) ) ;
#214161=EDGE_CURVE ( 'NONE', #205391, #41837, #199321, .T. ) ;
#214264=CARTESIAN_POINT ( 'NONE',  ( -6.708500942254057897E-15, -5.907420853759271395, -11.00029519899099029 ) ) ;
#214339=DIRECTION ( 'NONE',  ( 0.000000000000000000, 0.000000000000000000, 1.000000000000000000 ) ) ;
#214343=STYLED_ITEM ( 'NONE', ( #175257 ), #25207 ) ;
#214365=SURFACE_STYLE_FILL_AREA ( #141206 ) ;
#214398=CARTESIAN_POINT ( 'NONE',  ( -0.09916492693111574053, -9.919999999999998153, -9.499482423651645746 ) ) ;
#214399=CARTESIAN_POINT ( 'NONE',  ( -0.2883962233416142440, -9.094943692057514184, 9.630124952822544770 ) ) ;
ENDSEC;
END-ISO-10303-21;
